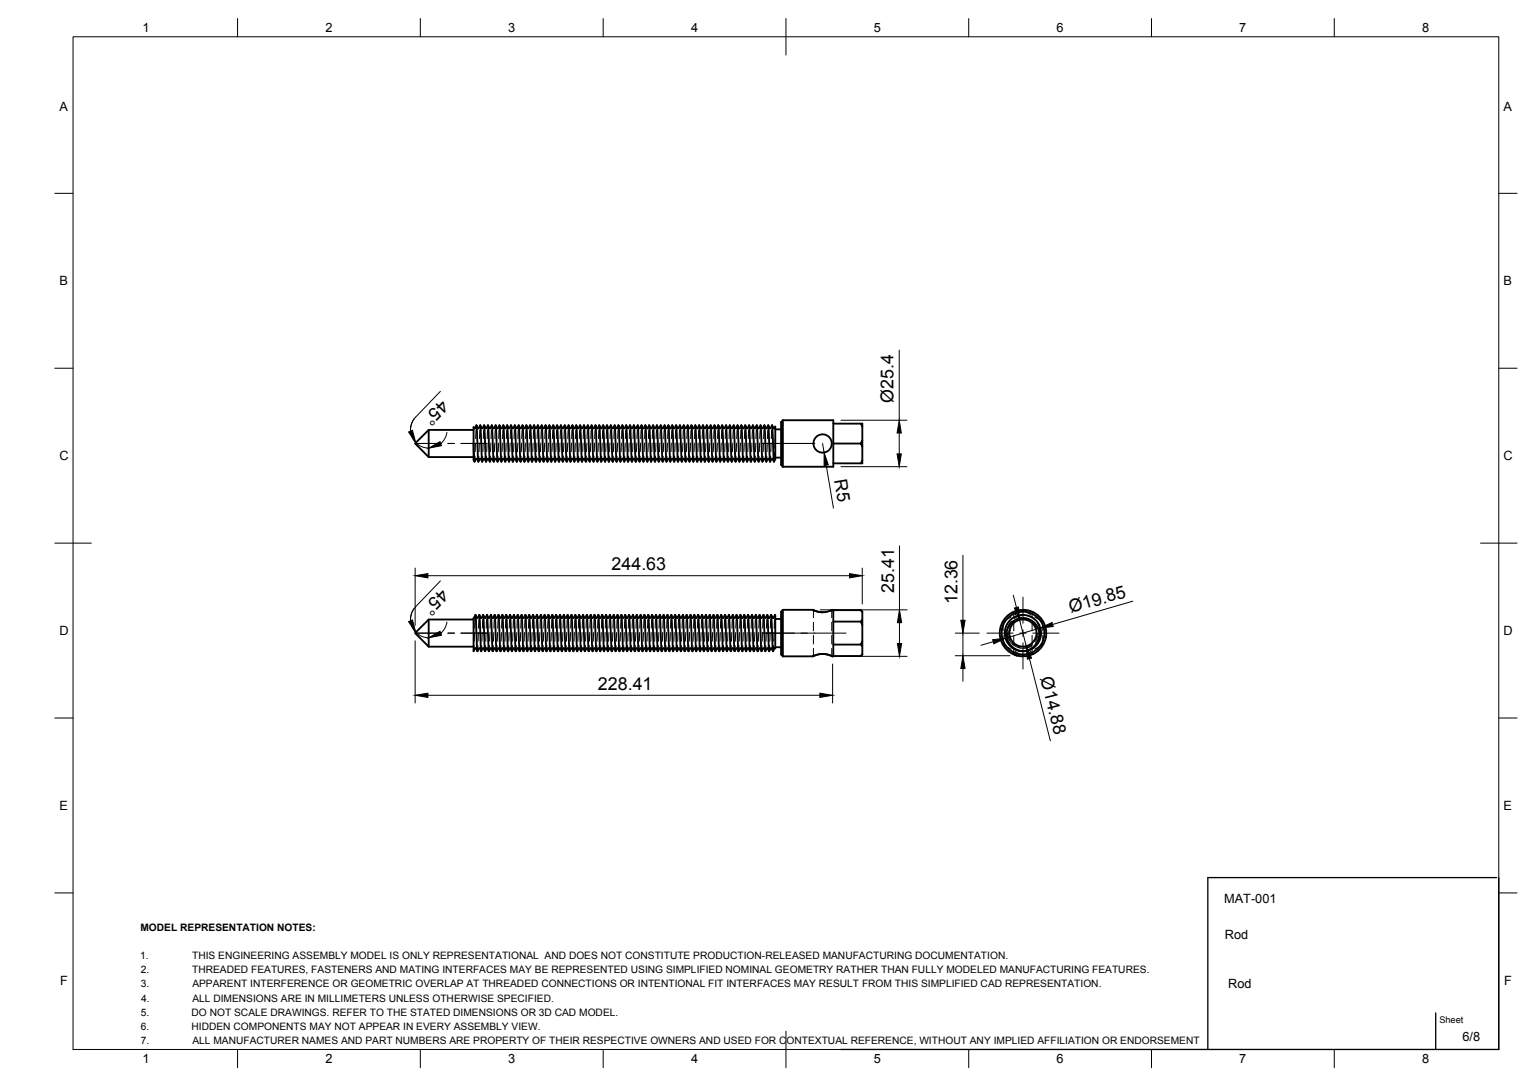
ISO-10303-21;
HEADER;
/* Generated by software containing ST-Developer
 * from STEP Tools, Inc. (www.steptools.com) 
 */

FILE_DESCRIPTION(
/* description */ ('STEP AP214'),
/* implementation_level */ '2;1');

FILE_NAME(
/* name */ 'Rod.step',
/* time_stamp */ '2026-11-14T04:30:00-08:00',
/* author */ (''),
/* organization */ (''),
/* preprocessor_version */ 'ST-DEVELOPER v20.2',
/* originating_system */ 'Autodesk Translation Framework v15.17.0.0',
/* authorisation */ '');

FILE_SCHEMA (('AUTOMOTIVE_DESIGN { 1 0 10303 214 3 1 1 }'));
ENDSEC;

DATA;
#10=MECHANICAL_DESIGN_GEOMETRIC_PRESENTATION_REPRESENTATION('',(#124),#40809);
#108=SHAPE_REPRESENTATION_RELATIONSHIP('SRR','None',#40858,#116);
#116=ADVANCED_BREP_SHAPE_REPRESENTATION('',(#132),#40802);
#124=STYLED_ITEM('',(#40907),#132);
#132=MANIFOLD_SOLID_BREP('Body1',#6299);
#176=(
BOUNDED_SURFACE()
B_SPLINE_SURFACE(3,2,((#27166,#27167,#27168),(#27169,#27170,#27171),(#27172,
#27173,#27174),(#27175,#27176,#27177),(#27178,#27179,#27180),(#27181,#27182,
#27183),(#27184,#27185,#27186),(#27187,#27188,#27189),(#27190,#27191,#27192),
(#27193,#27194,#27195),(#27196,#27197,#27198),(#27199,#27200,#27201),(#27202,
#27203,#27204),(#27205,#27206,#27207),(#27208,#27209,#27210),(#27211,#27212,
#27213),(#27214,#27215,#27216),(#27217,#27218,#27219),(#27220,#27221,#27222),
(#27223,#27224,#27225),(#27226,#27227,#27228),(#27229,#27230,#27231),(#27232,
#27233,#27234),(#27235,#27236,#27237),(#27238,#27239,#27240),(#27241,#27242,
#27243),(#27244,#27245,#27246),(#27247,#27248,#27249),(#27250,#27251,#27252),
(#27253,#27254,#27255),(#27256,#27257,#27258),(#27259,#27260,#27261),(#27262,
#27263,#27264),(#27265,#27266,#27267),(#27268,#27269,#27270),(#27271,#27272,
#27273),(#27274,#27275,#27276),(#27277,#27278,#27279),(#27280,#27281,#27282),
(#27283,#27284,#27285),(#27286,#27287,#27288),(#27289,#27290,#27291)),
 .UNSPECIFIED.,.F.,.F.,.F.)
B_SPLINE_SURFACE_WITH_KNOTS((4,2,2,2,2,2,2,2,2,2,2,2,2,2,2,2,2,2,2,2,4),
(3,3),(-7.80561738159264E-5,0.00108972446965002,0.00217944893930003,0.00326917340895005,
0.00435889787860006,0.00490376011342507,0.00544862234825008,0.00653834681790009,
0.00762807128755011,0.00871779575720013,0.00926265799202513,0.00980752022685014,
0.0103523824616751,0.0108972446965002,0.0119869691661502,0.0130766936358002,
0.0141664181054502,0.0152561425751002,0.0158010048099252,0.0163458670447502,
0.0174687351854262),(-3.31436710259121E-5,1.00007805617382),
 .UNSPECIFIED.)
GEOMETRIC_REPRESENTATION_ITEM()
RATIONAL_B_SPLINE_SURFACE(((1.00003154503853,0.524079561564375,1.00007429459434),
(1.0000315937412,0.523344783661835,1.00007440929844),(1.00003141682542,
0.526013914411658,1.00007399262799),(1.0000307068602,0.536725169717461,
1.0000723205242),(1.00003019055673,0.544514647394406,1.00007110453086),
(1.00002895723913,0.563121727335801,1.00006819983221),(1.0000282411969,
0.573924666524174,1.00006651341591),(1.00002671338234,0.596974826160331,
1.00006291512064),(1.00002591662213,0.608995558662043,1.00006103859807),
(1.00002475586398,0.626507933141575,1.00005830479079),(1.00002437347723,
0.632277007329064,1.00005740419693),(1.00002362687254,0.643541042834223,
1.00005564580019),(1.00002326100253,0.649060928800113,1.00005478410639),
(1.00002222356725,0.664712729342052,1.00005234074805),(1.00002160723677,
0.674011315953667,1.00005088917198),(1.00002057219885,0.689626947600185,
1.00004845145987),(1.00002015115486,0.695979244110157,1.00004745982082),
(1.00001958356106,0.704542539723916,1.00004612302894),(1.00001943064549,
0.706849579098284,1.00004576288355),(1.00001940985656,0.707163222049774,
1.00004571392163),(1.00001943845365,0.706731777363891,1.00004578127324),
(1.00001956476706,0.704826085066601,1.00004607876548),(1.00001966207446,
0.703358006931155,1.00004630794301),(1.00001992151192,0.69944387046907,
1.00004691896779),(1.00002008365206,0.696997659863913,1.00004730083881),
(1.00002047017319,0.691166210187756,1.00004821116994),(1.00002069610127,
0.687757630052989,1.00004874327375),(1.00002145040546,0.676377432111549,
1.00005051980428),(1.00002205383492,0.667273483461506,1.00005194099597),
(1.00002340996085,0.646813592510669,1.00005513493171),(1.0000241670402,
0.635391525693089,1.00005691799827),(1.00002570900064,0.612127947016899,
1.00006054960978),(1.00002650093244,0.600180060818586,1.00006241476052),
(1.0000280417883,0.576933146876439,1.00006604377054),(1.00002877367107,
0.565891221185074,1.00006776749435),(1.00002972027581,0.551609782278378,
1.00006999692941),(1.0000300115584,0.547215197654337,1.00007068295559),
(1.00003053161739,0.53936906050514,1.00007190779388),(1.00003076145279,
0.535901530604989,1.00007244910017),(1.00003133743645,0.527211656986592,
1.00007380565178),(1.00003154549653,0.52407265171366,1.00007429567302),
(1.00003155264458,0.523964808953251,1.00007431250805)))
REPRESENTATION_ITEM('')
SURFACE()
);
#177=(
BOUNDED_SURFACE()
B_SPLINE_SURFACE(3,2,((#27578,#27579,#27580),(#27581,#27582,#27583),(#27584,
#27585,#27586),(#27587,#27588,#27589),(#27590,#27591,#27592),(#27593,#27594,
#27595),(#27596,#27597,#27598),(#27599,#27600,#27601),(#27602,#27603,#27604),
(#27605,#27606,#27607),(#27608,#27609,#27610),(#27611,#27612,#27613),(#27614,
#27615,#27616),(#27617,#27618,#27619),(#27620,#27621,#27622),(#27623,#27624,
#27625),(#27626,#27627,#27628),(#27629,#27630,#27631),(#27632,#27633,#27634),
(#27635,#27636,#27637),(#27638,#27639,#27640),(#27641,#27642,#27643),(#27644,
#27645,#27646),(#27647,#27648,#27649),(#27650,#27651,#27652),(#27653,#27654,
#27655),(#27656,#27657,#27658),(#27659,#27660,#27661),(#27662,#27663,#27664),
(#27665,#27666,#27667),(#27668,#27669,#27670),(#27671,#27672,#27673),(#27674,
#27675,#27676),(#27677,#27678,#27679),(#27680,#27681,#27682),(#27683,#27684,
#27685),(#27686,#27687,#27688),(#27689,#27690,#27691),(#27692,#27693,#27694),
(#27695,#27696,#27697),(#27698,#27699,#27700),(#27701,#27702,#27703)),
 .UNSPECIFIED.,.F.,.F.,.F.)
B_SPLINE_SURFACE_WITH_KNOTS((4,2,2,2,2,2,2,2,2,2,2,2,2,2,2,2,2,2,2,2,4),
(3,3),(0.,0.00108936814645749,0.00217873629291499,0.00326810443937248,0.00435747258582998,
0.00490215665905872,0.00544684073228747,0.00653620887874497,0.00762557702520246,
0.00871494517165995,0.0092596292448887,0.00980431331811745,0.0103489973913462,
0.0108936814645749,0.0119830496110324,0.0130724177574899,0.0141617859039474,
0.0152511540504049,0.0157958381236337,0.0163405221968624,0.0174298903433199),
(0.,1.),.UNSPECIFIED.)
GEOMETRIC_REPRESENTATION_ITEM()
RATIONAL_B_SPLINE_SURFACE(((1.,0.706882331541542,1.),(1.,0.707679638835941,
1.),(1.,0.706337831680188,1.),(1.,0.699641298231053,1.),(1.,0.694186850878167,
1.),(1.,0.680019624674915,1.),(1.,0.671327778173696,1.),(1.,0.65139771038903,
1.),(1.,0.640295384304893,1.),(1.,0.623043177807755,1.),(1.,0.617175274503255,
1.),(1.,0.605346721741376,1.),(1.,0.599355525156456,1.),(1.,0.581798773133271,
1.),(1.,0.570600832874572,1.),(1.,0.550711868458482,1.),(1.,0.541963614343013,
1.),(1.,0.529372137830182,1.),(1.,0.525443344962623,1.),(1.,0.523784577113156,
1.),(1.,0.523945004135255,1.),(1.,0.525692544902627,1.),(1.,0.527267041649223,
1.),(1.,0.531692982742457,1.),(1.,0.534544195639033,1.),(1.,0.541381698420683,
1.),(1.,0.545393688389137,1.),(1.,0.55869257877852,1.),(1.,0.569170005808865,
1.),(1.,0.591697019613681,1.),(1.,0.603798924645628,1.),(1.,0.6273058031179,
1.),(1.,0.638830492715536,1.),(1.,0.660348218640802,1.),(1.,0.670109592161733,
1.),(1.,0.682456253372296,1.),(1.,0.686205595551818,1.),(1.,0.692883150338747,
1.),(1.,0.695824965165441,1.),(1.,0.703162804007318,1.),(1.,0.706044886129699,
1.),(1.,0.706866009891837,1.)))
REPRESENTATION_ITEM('')
SURFACE()
);
#178=(
BOUNDED_SURFACE()
B_SPLINE_SURFACE(1,2,((#28772,#28773,#28774,#28775,#28776,#28777,#28778,
#28779,#28780,#28781,#28782,#28783,#28784,#28785,#28786,#28787,#28788,#28789,
#28790,#28791,#28792,#28793,#28794,#28795,#28796,#28797,#28798,#28799,#28800,
#28801,#28802,#28803,#28804,#28805,#28806,#28807,#28808,#28809,#28810,#28811,
#28812,#28813,#28814,#28815,#28816,#28817,#28818,#28819,#28820,#28821,#28822,
#28823,#28824,#28825,#28826,#28827,#28828,#28829,#28830,#28831,#28832,#28833,
#28834,#28835,#28836,#28837,#28838,#28839,#28840,#28841,#28842,#28843,#28844,
#28845,#28846,#28847,#28848,#28849,#28850,#28851,#28852,#28853,#28854,#28855,
#28856,#28857,#28858,#28859,#28860,#28861,#28862,#28863,#28864,#28865,#28866,
#28867,#28868,#28869,#28870,#28871,#28872,#28873,#28874,#28875,#28876,#28877,
#28878,#28879,#28880,#28881,#28882,#28883,#28884,#28885,#28886,#28887,#28888,
#28889,#28890,#28891,#28892,#28893,#28894,#28895,#28896,#28897,#28898,#28899,
#28900,#28901,#28902,#28903,#28904,#28905,#28906,#28907,#28908,#28909,#28910,
#28911,#28912,#28913,#28914,#28915,#28916,#28917,#28918,#28919,#28920,#28921,
#28922,#28923,#28924,#28925,#28926,#28927,#28928,#28929,#28930,#28931,#28932,
#28933,#28934,#28935,#28936,#28937,#28938,#28939,#28940,#28941,#28942,#28943,
#28944,#28945,#28946,#28947,#28948,#28949,#28950,#28951,#28952,#28953,#28954,
#28955,#28956,#28957,#28958,#28959,#28960,#28961,#28962,#28963,#28964,#28965,
#28966,#28967,#28968,#28969,#28970,#28971,#28972,#28973,#28974,#28975,#28976,
#28977,#28978,#28979,#28980,#28981,#28982,#28983,#28984,#28985,#28986,#28987,
#28988,#28989,#28990,#28991,#28992,#28993,#28994,#28995,#28996,#28997,#28998,
#28999,#29000,#29001,#29002,#29003,#29004,#29005,#29006,#29007,#29008,#29009,
#29010,#29011,#29012,#29013,#29014,#29015,#29016,#29017,#29018,#29019,#29020,
#29021,#29022,#29023,#29024,#29025,#29026,#29027,#29028,#29029,#29030,#29031,
#29032,#29033,#29034,#29035,#29036,#29037,#29038,#29039,#29040,#29041,#29042,
#29043,#29044,#29045,#29046,#29047,#29048,#29049,#29050,#29051,#29052,#29053,
#29054,#29055,#29056,#29057,#29058,#29059,#29060,#29061,#29062,#29063,#29064,
#29065,#29066,#29067,#29068,#29069,#29070,#29071,#29072,#29073,#29074,#29075,
#29076,#29077,#29078,#29079,#29080,#29081,#29082,#29083,#29084,#29085,#29086,
#29087,#29088,#29089,#29090,#29091,#29092,#29093,#29094,#29095,#29096,#29097,
#29098,#29099,#29100,#29101,#29102,#29103,#29104,#29105,#29106,#29107,#29108,
#29109,#29110,#29111,#29112,#29113,#29114,#29115,#29116,#29117,#29118,#29119,
#29120,#29121,#29122,#29123,#29124,#29125,#29126,#29127,#29128,#29129,#29130,
#29131,#29132,#29133,#29134,#29135,#29136,#29137,#29138,#29139,#29140,#29141,
#29142,#29143,#29144,#29145,#29146,#29147,#29148,#29149,#29150,#29151,#29152,
#29153,#29154,#29155,#29156,#29157,#29158,#29159,#29160,#29161,#29162,#29163,
#29164,#29165,#29166,#29167,#29168,#29169,#29170,#29171,#29172,#29173,#29174,
#29175,#29176,#29177,#29178,#29179,#29180,#29181,#29182,#29183,#29184,#29185,
#29186,#29187,#29188,#29189,#29190,#29191,#29192,#29193,#29194,#29195,#29196,
#29197,#29198,#29199,#29200,#29201,#29202,#29203,#29204,#29205,#29206,#29207,
#29208,#29209,#29210,#29211,#29212,#29213,#29214,#29215,#29216,#29217,#29218,
#29219,#29220,#29221,#29222,#29223,#29224,#29225,#29226,#29227,#29228,#29229,
#29230,#29231,#29232,#29233,#29234,#29235,#29236,#29237,#29238,#29239,#29240,
#29241,#29242,#29243,#29244,#29245,#29246,#29247,#29248,#29249,#29250,#29251,
#29252,#29253,#29254,#29255,#29256,#29257,#29258,#29259,#29260,#29261,#29262,
#29263,#29264,#29265,#29266,#29267,#29268,#29269,#29270,#29271,#29272,#29273,
#29274,#29275,#29276,#29277,#29278,#29279,#29280,#29281,#29282,#29283,#29284,
#29285,#29286,#29287,#29288,#29289,#29290,#29291,#29292,#29293,#29294,#29295,
#29296,#29297,#29298,#29299,#29300,#29301,#29302,#29303,#29304,#29305,#29306,
#29307,#29308,#29309,#29310,#29311,#29312,#29313,#29314,#29315,#29316,#29317,
#29318,#29319,#29320,#29321,#29322,#29323,#29324,#29325,#29326,#29327,#29328,
#29329,#29330,#29331,#29332,#29333,#29334,#29335,#29336,#29337,#29338,#29339,
#29340,#29341,#29342,#29343,#29344,#29345,#29346,#29347,#29348,#29349,#29350,
#29351,#29352,#29353,#29354,#29355,#29356,#29357,#29358,#29359,#29360,#29361,
#29362,#29363,#29364,#29365,#29366,#29367,#29368,#29369,#29370,#29371,#29372,
#29373,#29374,#29375,#29376,#29377,#29378,#29379,#29380,#29381,#29382,#29383,
#29384,#29385,#29386,#29387,#29388,#29389,#29390,#29391,#29392,#29393,#29394,
#29395,#29396,#29397,#29398,#29399,#29400,#29401,#29402,#29403,#29404,#29405,
#29406,#29407,#29408,#29409,#29410,#29411,#29412,#29413,#29414,#29415,#29416,
#29417,#29418,#29419,#29420,#29421,#29422,#29423,#29424,#29425,#29426,#29427,
#29428,#29429,#29430,#29431,#29432,#29433,#29434,#29435,#29436,#29437,#29438,
#29439,#29440,#29441,#29442,#29443,#29444,#29445,#29446,#29447,#29448,#29449,
#29450,#29451,#29452,#29453,#29454,#29455,#29456,#29457,#29458,#29459,#29460,
#29461,#29462,#29463,#29464,#29465,#29466,#29467,#29468,#29469,#29470,#29471,
#29472,#29473,#29474,#29475,#29476,#29477,#29478,#29479,#29480,#29481,#29482,
#29483,#29484,#29485,#29486,#29487,#29488,#29489,#29490,#29491,#29492,#29493,
#29494,#29495,#29496,#29497,#29498,#29499,#29500,#29501,#29502,#29503,#29504,
#29505,#29506,#29507,#29508,#29509,#29510,#29511,#29512,#29513,#29514,#29515,
#29516,#29517,#29518,#29519,#29520,#29521,#29522,#29523,#29524,#29525,#29526,
#29527,#29528,#29529,#29530,#29531,#29532,#29533,#29534,#29535,#29536,#29537,
#29538,#29539,#29540,#29541,#29542,#29543,#29544,#29545,#29546,#29547,#29548,
#29549,#29550,#29551,#29552,#29553,#29554,#29555,#29556,#29557,#29558,#29559,
#29560,#29561,#29562,#29563,#29564,#29565,#29566,#29567,#29568,#29569,#29570,
#29571,#29572,#29573,#29574,#29575,#29576,#29577,#29578,#29579,#29580,#29581,
#29582,#29583,#29584,#29585,#29586,#29587,#29588,#29589,#29590,#29591,#29592,
#29593,#29594,#29595,#29596,#29597,#29598,#29599,#29600,#29601,#29602,#29603,
#29604,#29605,#29606,#29607,#29608,#29609,#29610,#29611,#29612,#29613,#29614,
#29615,#29616,#29617,#29618,#29619,#29620,#29621,#29622,#29623,#29624,#29625,
#29626,#29627,#29628,#29629,#29630,#29631,#29632,#29633,#29634,#29635,#29636,
#29637,#29638,#29639,#29640,#29641,#29642,#29643,#29644,#29645,#29646,#29647,
#29648,#29649,#29650,#29651,#29652,#29653,#29654,#29655,#29656,#29657,#29658,
#29659,#29660,#29661,#29662,#29663,#29664,#29665,#29666,#29667,#29668,#29669,
#29670,#29671,#29672,#29673,#29674,#29675,#29676,#29677,#29678,#29679,#29680,
#29681,#29682,#29683,#29684,#29685,#29686,#29687,#29688,#29689,#29690,#29691,
#29692,#29693,#29694,#29695,#29696,#29697,#29698,#29699,#29700,#29701,#29702,
#29703,#29704,#29705,#29706,#29707,#29708,#29709,#29710,#29711,#29712,#29713,
#29714,#29715,#29716,#29717,#29718,#29719,#29720,#29721,#29722,#29723,#29724,
#29725,#29726,#29727,#29728,#29729,#29730,#29731,#29732,#29733,#29734,#29735,
#29736,#29737,#29738,#29739,#29740,#29741,#29742,#29743,#29744),(#29745,
#29746,#29747,#29748,#29749,#29750,#29751,#29752,#29753,#29754,#29755,#29756,
#29757,#29758,#29759,#29760,#29761,#29762,#29763,#29764,#29765,#29766,#29767,
#29768,#29769,#29770,#29771,#29772,#29773,#29774,#29775,#29776,#29777,#29778,
#29779,#29780,#29781,#29782,#29783,#29784,#29785,#29786,#29787,#29788,#29789,
#29790,#29791,#29792,#29793,#29794,#29795,#29796,#29797,#29798,#29799,#29800,
#29801,#29802,#29803,#29804,#29805,#29806,#29807,#29808,#29809,#29810,#29811,
#29812,#29813,#29814,#29815,#29816,#29817,#29818,#29819,#29820,#29821,#29822,
#29823,#29824,#29825,#29826,#29827,#29828,#29829,#29830,#29831,#29832,#29833,
#29834,#29835,#29836,#29837,#29838,#29839,#29840,#29841,#29842,#29843,#29844,
#29845,#29846,#29847,#29848,#29849,#29850,#29851,#29852,#29853,#29854,#29855,
#29856,#29857,#29858,#29859,#29860,#29861,#29862,#29863,#29864,#29865,#29866,
#29867,#29868,#29869,#29870,#29871,#29872,#29873,#29874,#29875,#29876,#29877,
#29878,#29879,#29880,#29881,#29882,#29883,#29884,#29885,#29886,#29887,#29888,
#29889,#29890,#29891,#29892,#29893,#29894,#29895,#29896,#29897,#29898,#29899,
#29900,#29901,#29902,#29903,#29904,#29905,#29906,#29907,#29908,#29909,#29910,
#29911,#29912,#29913,#29914,#29915,#29916,#29917,#29918,#29919,#29920,#29921,
#29922,#29923,#29924,#29925,#29926,#29927,#29928,#29929,#29930,#29931,#29932,
#29933,#29934,#29935,#29936,#29937,#29938,#29939,#29940,#29941,#29942,#29943,
#29944,#29945,#29946,#29947,#29948,#29949,#29950,#29951,#29952,#29953,#29954,
#29955,#29956,#29957,#29958,#29959,#29960,#29961,#29962,#29963,#29964,#29965,
#29966,#29967,#29968,#29969,#29970,#29971,#29972,#29973,#29974,#29975,#29976,
#29977,#29978,#29979,#29980,#29981,#29982,#29983,#29984,#29985,#29986,#29987,
#29988,#29989,#29990,#29991,#29992,#29993,#29994,#29995,#29996,#29997,#29998,
#29999,#30000,#30001,#30002,#30003,#30004,#30005,#30006,#30007,#30008,#30009,
#30010,#30011,#30012,#30013,#30014,#30015,#30016,#30017,#30018,#30019,#30020,
#30021,#30022,#30023,#30024,#30025,#30026,#30027,#30028,#30029,#30030,#30031,
#30032,#30033,#30034,#30035,#30036,#30037,#30038,#30039,#30040,#30041,#30042,
#30043,#30044,#30045,#30046,#30047,#30048,#30049,#30050,#30051,#30052,#30053,
#30054,#30055,#30056,#30057,#30058,#30059,#30060,#30061,#30062,#30063,#30064,
#30065,#30066,#30067,#30068,#30069,#30070,#30071,#30072,#30073,#30074,#30075,
#30076,#30077,#30078,#30079,#30080,#30081,#30082,#30083,#30084,#30085,#30086,
#30087,#30088,#30089,#30090,#30091,#30092,#30093,#30094,#30095,#30096,#30097,
#30098,#30099,#30100,#30101,#30102,#30103,#30104,#30105,#30106,#30107,#30108,
#30109,#30110,#30111,#30112,#30113,#30114,#30115,#30116,#30117,#30118,#30119,
#30120,#30121,#30122,#30123,#30124,#30125,#30126,#30127,#30128,#30129,#30130,
#30131,#30132,#30133,#30134,#30135,#30136,#30137,#30138,#30139,#30140,#30141,
#30142,#30143,#30144,#30145,#30146,#30147,#30148,#30149,#30150,#30151,#30152,
#30153,#30154,#30155,#30156,#30157,#30158,#30159,#30160,#30161,#30162,#30163,
#30164,#30165,#30166,#30167,#30168,#30169,#30170,#30171,#30172,#30173,#30174,
#30175,#30176,#30177,#30178,#30179,#30180,#30181,#30182,#30183,#30184,#30185,
#30186,#30187,#30188,#30189,#30190,#30191,#30192,#30193,#30194,#30195,#30196,
#30197,#30198,#30199,#30200,#30201,#30202,#30203,#30204,#30205,#30206,#30207,
#30208,#30209,#30210,#30211,#30212,#30213,#30214,#30215,#30216,#30217,#30218,
#30219,#30220,#30221,#30222,#30223,#30224,#30225,#30226,#30227,#30228,#30229,
#30230,#30231,#30232,#30233,#30234,#30235,#30236,#30237,#30238,#30239,#30240,
#30241,#30242,#30243,#30244,#30245,#30246,#30247,#30248,#30249,#30250,#30251,
#30252,#30253,#30254,#30255,#30256,#30257,#30258,#30259,#30260,#30261,#30262,
#30263,#30264,#30265,#30266,#30267,#30268,#30269,#30270,#30271,#30272,#30273,
#30274,#30275,#30276,#30277,#30278,#30279,#30280,#30281,#30282,#30283,#30284,
#30285,#30286,#30287,#30288,#30289,#30290,#30291,#30292,#30293,#30294,#30295,
#30296,#30297,#30298,#30299,#30300,#30301,#30302,#30303,#30304,#30305,#30306,
#30307,#30308,#30309,#30310,#30311,#30312,#30313,#30314,#30315,#30316,#30317,
#30318,#30319,#30320,#30321,#30322,#30323,#30324,#30325,#30326,#30327,#30328,
#30329,#30330,#30331,#30332,#30333,#30334,#30335,#30336,#30337,#30338,#30339,
#30340,#30341,#30342,#30343,#30344,#30345,#30346,#30347,#30348,#30349,#30350,
#30351,#30352,#30353,#30354,#30355,#30356,#30357,#30358,#30359,#30360,#30361,
#30362,#30363,#30364,#30365,#30366,#30367,#30368,#30369,#30370,#30371,#30372,
#30373,#30374,#30375,#30376,#30377,#30378,#30379,#30380,#30381,#30382,#30383,
#30384,#30385,#30386,#30387,#30388,#30389,#30390,#30391,#30392,#30393,#30394,
#30395,#30396,#30397,#30398,#30399,#30400,#30401,#30402,#30403,#30404,#30405,
#30406,#30407,#30408,#30409,#30410,#30411,#30412,#30413,#30414,#30415,#30416,
#30417,#30418,#30419,#30420,#30421,#30422,#30423,#30424,#30425,#30426,#30427,
#30428,#30429,#30430,#30431,#30432,#30433,#30434,#30435,#30436,#30437,#30438,
#30439,#30440,#30441,#30442,#30443,#30444,#30445,#30446,#30447,#30448,#30449,
#30450,#30451,#30452,#30453,#30454,#30455,#30456,#30457,#30458,#30459,#30460,
#30461,#30462,#30463,#30464,#30465,#30466,#30467,#30468,#30469,#30470,#30471,
#30472,#30473,#30474,#30475,#30476,#30477,#30478,#30479,#30480,#30481,#30482,
#30483,#30484,#30485,#30486,#30487,#30488,#30489,#30490,#30491,#30492,#30493,
#30494,#30495,#30496,#30497,#30498,#30499,#30500,#30501,#30502,#30503,#30504,
#30505,#30506,#30507,#30508,#30509,#30510,#30511,#30512,#30513,#30514,#30515,
#30516,#30517,#30518,#30519,#30520,#30521,#30522,#30523,#30524,#30525,#30526,
#30527,#30528,#30529,#30530,#30531,#30532,#30533,#30534,#30535,#30536,#30537,
#30538,#30539,#30540,#30541,#30542,#30543,#30544,#30545,#30546,#30547,#30548,
#30549,#30550,#30551,#30552,#30553,#30554,#30555,#30556,#30557,#30558,#30559,
#30560,#30561,#30562,#30563,#30564,#30565,#30566,#30567,#30568,#30569,#30570,
#30571,#30572,#30573,#30574,#30575,#30576,#30577,#30578,#30579,#30580,#30581,
#30582,#30583,#30584,#30585,#30586,#30587,#30588,#30589,#30590,#30591,#30592,
#30593,#30594,#30595,#30596,#30597,#30598,#30599,#30600,#30601,#30602,#30603,
#30604,#30605,#30606,#30607,#30608,#30609,#30610,#30611,#30612,#30613,#30614,
#30615,#30616,#30617,#30618,#30619,#30620,#30621,#30622,#30623,#30624,#30625,
#30626,#30627,#30628,#30629,#30630,#30631,#30632,#30633,#30634,#30635,#30636,
#30637,#30638,#30639,#30640,#30641,#30642,#30643,#30644,#30645,#30646,#30647,
#30648,#30649,#30650,#30651,#30652,#30653,#30654,#30655,#30656,#30657,#30658,
#30659,#30660,#30661,#30662,#30663,#30664,#30665,#30666,#30667,#30668,#30669,
#30670,#30671,#30672,#30673,#30674,#30675,#30676,#30677,#30678,#30679,#30680,
#30681,#30682,#30683,#30684,#30685,#30686,#30687,#30688,#30689,#30690,#30691,
#30692,#30693,#30694,#30695,#30696,#30697,#30698,#30699,#30700,#30701,#30702,
#30703,#30704,#30705,#30706,#30707,#30708,#30709,#30710,#30711,#30712,#30713,
#30714,#30715,#30716,#30717)),.UNSPECIFIED.,.F.,.F.,.F.)
B_SPLINE_SURFACE_WITH_KNOTS((2,2),(3,2,2,2,2,2,2,2,2,2,2,2,2,2,2,2,2,2,
2,2,2,2,2,2,2,2,2,2,2,2,2,2,2,2,2,2,2,2,2,2,2,2,2,2,2,2,2,2,2,2,2,2,2,2,
2,2,2,2,2,2,2,2,2,2,2,2,2,2,2,2,2,2,2,2,2,2,2,2,2,2,2,2,2,2,2,2,2,2,2,2,
2,2,2,2,2,2,2,2,2,2,2,2,2,2,2,2,2,2,2,2,2,2,2,2,2,2,2,2,2,2,2,2,2,2,2,2,
2,2,2,2,2,2,2,2,2,2,2,2,2,2,2,2,2,2,2,2,2,2,2,2,2,2,2,2,2,2,2,2,2,2,2,2,
2,2,2,2,2,2,2,2,2,2,2,2,2,2,2,2,2,2,2,2,2,2,2,2,2,2,2,2,2,2,2,2,2,2,2,2,
2,2,2,2,2,2,2,2,2,2,2,2,2,2,2,2,2,2,2,2,2,2,2,2,2,2,2,2,2,2,2,2,2,2,2,2,
2,2,2,2,2,2,2,2,2,2,2,2,2,2,2,2,2,2,2,2,2,2,2,2,2,2,2,2,2,2,2,2,2,2,2,2,
2,2,2,2,2,2,2,2,2,2,2,2,2,2,2,2,2,2,2,2,2,2,2,2,2,2,2,2,2,2,2,2,2,2,2,2,
2,2,2,2,2,2,2,2,2,2,2,2,2,2,2,2,2,2,2,2,2,2,2,2,2,2,2,2,2,2,2,2,2,2,2,2,
2,2,2,2,2,2,2,2,2,2,2,2,2,2,2,2,2,2,2,2,2,2,2,2,2,2,2,2,2,2,2,2,2,2,2,2,
2,2,2,2,2,2,2,2,2,2,2,2,2,2,2,2,2,2,2,2,2,2,2,2,2,2,2,2,2,2,2,2,2,2,2,2,
2,2,2,2,2,2,2,2,2,2,2,2,2,2,2,2,2,2,2,2,2,2,2,2,2,2,2,2,2,2,2,2,2,2,2,2,
2,2,2,2,2,2,2,2,2,2,2,2,2,2,2,2,2,2,2,2,2,2,2,2,2,2,2,2,2,2,2,2,2,2,2,2,
3),(0.,1.),(0.,0.00205761316872428,0.00411522633744856,0.00617283950617284,
0.00823045267489712,0.0102880658436214,0.0123456790123457,0.01440329218107,
0.0164609053497942,0.0185185185185185,0.0205761316872428,0.0226337448559671,
0.0246913580246914,0.0267489711934156,0.0288065843621399,0.0308641975308642,
0.0329218106995885,0.0349794238683128,0.037037037037037,0.0390946502057613,
0.0411522633744856,0.0432098765432099,0.0452674897119342,0.0473251028806584,
0.0493827160493827,0.051440329218107,0.0534979423868313,0.0555555555555556,
0.0576131687242798,0.0596707818930041,0.0617283950617284,0.0637860082304527,
0.065843621399177,0.0679012345679012,0.0699588477366255,0.0720164609053498,
0.0740740740740741,0.0761316872427984,0.0781893004115226,0.0802469135802469,
0.0823045267489712,0.0843621399176955,0.0864197530864197,0.088477366255144,
0.0905349794238683,0.0925925925925926,0.0946502057613169,0.0967078189300412,
0.0987654320987654,0.10082304526749,0.102880658436214,0.104938271604938,
0.106995884773663,0.109053497942387,0.111111111111111,0.113168724279835,
0.11522633744856,0.117283950617284,0.119341563786008,0.121399176954733,
0.123456790123457,0.125514403292181,0.127572016460905,0.12962962962963,
0.131687242798354,0.133744855967078,0.135802469135802,0.137860082304527,
0.139917695473251,0.141975308641975,0.1440329218107,0.146090534979424,0.148148148148148,
0.150205761316872,0.152263374485597,0.154320987654321,0.156378600823045,
0.15843621399177,0.160493827160494,0.162551440329218,0.164609053497942,
0.166666666666667,0.168724279835391,0.170781893004115,0.172839506172839,
0.174897119341564,0.176954732510288,0.179012345679012,0.181069958847737,
0.183127572016461,0.185185185185185,0.187242798353909,0.189300411522634,
0.191358024691358,0.193415637860082,0.195473251028807,0.197530864197531,
0.199588477366255,0.201646090534979,0.203703703703704,0.205761316872428,
0.207818930041152,0.209876543209877,0.211934156378601,0.213991769547325,
0.216049382716049,0.218106995884774,0.220164609053498,0.222222222222222,
0.224279835390947,0.226337448559671,0.228395061728395,0.230452674897119,
0.232510288065844,0.234567901234568,0.236625514403292,0.238683127572016,
0.240740740740741,0.242798353909465,0.244855967078189,0.246913580246914,
0.248971193415638,0.251028806584362,0.253086419753086,0.255144032921811,
0.257201646090535,0.259259259259259,0.261316872427984,0.263374485596708,
0.265432098765432,0.267489711934156,0.269547325102881,0.271604938271605,
0.273662551440329,0.275720164609054,0.277777777777778,0.279835390946502,
0.281893004115226,0.283950617283951,0.286008230452675,0.288065843621399,
0.290123456790123,0.292181069958848,0.294238683127572,0.296296296296296,
0.298353909465021,0.300411522633745,0.302469135802469,0.304526748971193,
0.306584362139918,0.308641975308642,0.310699588477366,0.312757201646091,
0.314814814814815,0.316872427983539,0.318930041152263,0.320987654320988,
0.323045267489712,0.325102880658436,0.327160493827161,0.329218106995885,
0.331275720164609,0.333333333333333,0.335390946502058,0.337448559670782,
0.339506172839506,0.34156378600823,0.343621399176955,0.345679012345679,
0.347736625514403,0.349794238683128,0.351851851851852,0.353909465020576,
0.3559670781893,0.358024691358025,0.360082304526749,0.362139917695473,0.364197530864198,
0.366255144032922,0.368312757201646,0.37037037037037,0.372427983539095,
0.374485596707819,0.376543209876543,0.378600823045267,0.380658436213992,
0.382716049382716,0.38477366255144,0.386831275720165,0.388888888888889,
0.390946502057613,0.393004115226337,0.395061728395062,0.397119341563786,
0.39917695473251,0.401234567901235,0.403292181069959,0.405349794238683,
0.407407407407407,0.409465020576132,0.411522633744856,0.41358024691358,
0.415637860082305,0.417695473251029,0.419753086419753,0.421810699588477,
0.423868312757202,0.425925925925926,0.42798353909465,0.430041152263374,
0.432098765432099,0.434156378600823,0.436213991769547,0.438271604938272,
0.440329218106996,0.44238683127572,0.444444444444444,0.446502057613169,
0.448559670781893,0.450617283950617,0.452674897119342,0.454732510288066,
0.45679012345679,0.458847736625514,0.460905349794239,0.462962962962963,
0.465020576131687,0.467078189300412,0.469135802469136,0.47119341563786,
0.473251028806584,0.475308641975309,0.477366255144033,0.479423868312757,
0.481481481481481,0.483539094650206,0.48559670781893,0.487654320987654,
0.489711934156379,0.491769547325103,0.493827160493827,0.495884773662551,
0.497942386831276,0.5,0.502057613168724,0.504115226337449,0.506172839506173,
0.508230452674897,0.510288065843621,0.512345679012346,0.51440329218107,
0.516460905349794,0.518518518518518,0.520576131687243,0.522633744855967,
0.524691358024691,0.526748971193416,0.52880658436214,0.530864197530864,
0.532921810699588,0.534979423868313,0.537037037037037,0.539094650205761,
0.541152263374486,0.54320987654321,0.545267489711934,0.547325102880658,
0.549382716049383,0.551440329218107,0.553497942386831,0.555555555555556,
0.55761316872428,0.559670781893004,0.561728395061728,0.563786008230453,
0.565843621399177,0.567901234567901,0.569958847736626,0.57201646090535,
0.574074074074074,0.576131687242798,0.578189300411523,0.580246913580247,
0.582304526748971,0.584362139917695,0.58641975308642,0.588477366255144,
0.590534979423868,0.592592592592593,0.594650205761317,0.596707818930041,
0.598765432098765,0.60082304526749,0.602880658436214,0.604938271604938,
0.606995884773663,0.609053497942387,0.611111111111111,0.613168724279835,
0.61522633744856,0.617283950617284,0.619341563786008,0.621399176954732,
0.623456790123457,0.625514403292181,0.627572016460905,0.62962962962963,
0.631687242798354,0.633744855967078,0.635802469135803,0.637860082304527,
0.639917695473251,0.641975308641975,0.6440329218107,0.646090534979424,0.648148148148148,
0.650205761316872,0.652263374485597,0.654320987654321,0.656378600823045,
0.65843621399177,0.660493827160494,0.662551440329218,0.664609053497942,
0.666666666666667,0.668724279835391,0.670781893004115,0.672839506172839,
0.674897119341564,0.676954732510288,0.679012345679012,0.681069958847737,
0.683127572016461,0.685185185185185,0.687242798353909,0.689300411522634,
0.691358024691358,0.693415637860082,0.695473251028807,0.697530864197531,
0.699588477366255,0.701646090534979,0.703703703703704,0.705761316872428,
0.707818930041152,0.709876543209877,0.711934156378601,0.713991769547325,
0.716049382716049,0.718106995884774,0.720164609053498,0.722222222222222,
0.724279835390947,0.726337448559671,0.728395061728395,0.730452674897119,
0.732510288065844,0.734567901234568,0.736625514403292,0.738683127572016,
0.740740740740741,0.742798353909465,0.744855967078189,0.746913580246914,
0.748971193415638,0.751028806584362,0.753086419753086,0.755144032921811,
0.757201646090535,0.759259259259259,0.761316872427984,0.763374485596708,
0.765432098765432,0.767489711934156,0.769547325102881,0.771604938271605,
0.773662551440329,0.775720164609053,0.777777777777778,0.779835390946502,
0.781893004115226,0.783950617283951,0.786008230452675,0.788065843621399,
0.790123456790123,0.792181069958848,0.794238683127572,0.796296296296296,
0.798353909465021,0.800411522633745,0.802469135802469,0.804526748971193,
0.806584362139918,0.808641975308642,0.810699588477366,0.812757201646091,
0.814814814814815,0.816872427983539,0.818930041152263,0.820987654320988,
0.823045267489712,0.825102880658436,0.827160493827161,0.829218106995885,
0.831275720164609,0.833333333333333,0.835390946502058,0.837448559670782,
0.839506172839506,0.84156378600823,0.843621399176955,0.845679012345679,
0.847736625514403,0.849794238683128,0.851851851851852,0.853909465020576,
0.8559670781893,0.858024691358025,0.860082304526749,0.862139917695473,0.864197530864197,
0.866255144032922,0.868312757201646,0.87037037037037,0.872427983539095,
0.874485596707819,0.876543209876543,0.878600823045268,0.880658436213992,
0.882716049382716,0.88477366255144,0.886831275720165,0.888888888888889,
0.890946502057613,0.893004115226337,0.895061728395062,0.897119341563786,
0.89917695473251,0.901234567901235,0.903292181069959,0.905349794238683,
0.907407407407407,0.909465020576132,0.911522633744856,0.91358024691358,
0.915637860082305,0.917695473251029,0.919753086419753,0.921810699588477,
0.923868312757202,0.925925925925926,0.92798353909465,0.930041152263374,
0.932098765432099,0.934156378600823,0.936213991769547,0.938271604938272,
0.940329218106996,0.94238683127572,0.944444444444444,0.946502057613169,
0.948559670781893,0.950617283950617,0.952674897119342,0.954732510288066,
0.95679012345679,0.958847736625514,0.960905349794239,0.962962962962963,
0.965020576131687,0.967078189300412,0.969135802469136,0.97119341563786,
0.973251028806584,0.975308641975309,0.977366255144033,0.979423868312757,
0.981481481481482,0.983539094650206,0.98559670781893,0.987654320987654,
0.989711934156379,0.991769547325103,0.993827160493827,0.995884773662551,
0.997942386831276,1.),.UNSPECIFIED.)
GEOMETRIC_REPRESENTATION_ITEM()
RATIONAL_B_SPLINE_SURFACE(((1.,0.866025403784439,1.,0.866025403784439,1.,
0.866025403784439,1.,0.866025403784439,1.,0.866025403784439,1.,0.866025403784439,
1.,0.866025403784439,1.,0.866025403784439,1.,0.866025403784439,1.,0.866025403784439,
1.,0.866025403784439,1.,0.866025403784439,1.,0.866025403784439,1.,0.866025403784439,
1.,0.866025403784439,1.,0.866025403784439,1.,0.866025403784439,1.,0.866025403784439,
1.,0.866025403784439,1.,0.866025403784439,1.,0.866025403784439,1.,0.866025403784439,
1.,0.866025403784439,1.,0.866025403784439,1.,0.866025403784439,1.,0.866025403784439,
1.,0.866025403784439,1.,0.866025403784439,1.,0.866025403784439,1.,0.866025403784439,
1.,0.866025403784439,1.,0.866025403784439,1.,0.866025403784439,1.,0.866025403784439,
1.,0.866025403784439,1.,0.866025403784439,1.,0.866025403784439,1.,0.866025403784439,
1.,0.866025403784439,1.,0.866025403784439,1.,0.866025403784439,1.,0.866025403784439,
1.,0.866025403784439,1.,0.866025403784439,1.,0.866025403784439,1.,0.866025403784439,
1.,0.866025403784439,1.,0.866025403784439,1.,0.866025403784439,1.,0.866025403784439,
1.,0.866025403784439,1.,0.866025403784439,1.,0.866025403784439,1.,0.866025403784439,
1.,0.866025403784439,1.,0.866025403784439,1.,0.866025403784439,1.,0.866025403784439,
1.,0.866025403784439,1.,0.866025403784439,1.,0.866025403784439,1.,0.866025403784439,
1.,0.866025403784439,1.,0.866025403784439,1.,0.866025403784439,1.,0.866025403784439,
1.,0.866025403784439,1.,0.866025403784439,1.,0.866025403784439,1.,0.866025403784439,
1.,0.866025403784439,1.,0.866025403784439,1.,0.866025403784439,1.,0.866025403784439,
1.,0.866025403784439,1.,0.866025403784439,1.,0.866025403784439,1.,0.866025403784439,
1.,0.866025403784439,1.,0.866025403784439,1.,0.866025403784439,1.,0.866025403784439,
1.,0.866025403784439,1.,0.866025403784439,1.,0.866025403784439,1.,0.866025403784439,
1.,0.866025403784439,1.,0.866025403784439,1.,0.866025403784439,1.,0.866025403784439,
1.,0.866025403784439,1.,0.866025403784439,1.,0.866025403784439,1.,0.866025403784439,
1.,0.866025403784439,1.,0.866025403784439,1.,0.866025403784439,1.,0.866025403784439,
1.,0.866025403784439,1.,0.866025403784439,1.,0.866025403784439,1.,0.866025403784439,
1.,0.866025403784439,1.,0.866025403784439,1.,0.866025403784439,1.,0.866025403784439,
1.,0.866025403784439,1.,0.866025403784439,1.,0.866025403784439,1.,0.866025403784439,
1.,0.866025403784439,1.,0.866025403784439,1.,0.866025403784439,1.,0.866025403784439,
1.,0.866025403784439,1.,0.866025403784439,1.,0.866025403784439,1.,0.866025403784439,
1.,0.866025403784439,1.,0.866025403784439,1.,0.866025403784439,1.,0.866025403784439,
1.,0.866025403784439,1.,0.866025403784439,1.,0.866025403784439,1.,0.866025403784439,
1.,0.866025403784439,1.,0.866025403784439,1.,0.866025403784439,1.,0.866025403784439,
1.,0.866025403784439,1.,0.866025403784439,1.,0.866025403784439,1.,0.866025403784439,
1.,0.866025403784439,1.,0.866025403784439,1.,0.866025403784439,1.,0.866025403784439,
1.,0.866025403784439,1.,0.866025403784439,1.,0.866025403784439,1.,0.866025403784439,
1.,0.866025403784439,1.,0.866025403784439,1.,0.866025403784439,1.,0.866025403784439,
1.,0.866025403784439,1.,0.866025403784439,1.,0.866025403784439,1.,0.866025403784439,
1.,0.866025403784439,1.,0.866025403784439,1.,0.866025403784439,1.,0.866025403784439,
1.,0.866025403784439,1.,0.866025403784439,1.,0.866025403784439,1.,0.866025403784439,
1.,0.866025403784439,1.,0.866025403784439,1.,0.866025403784439,1.,0.866025403784439,
1.,0.866025403784439,1.,0.866025403784439,1.,0.866025403784439,1.,0.866025403784439,
1.,0.866025403784439,1.,0.866025403784439,1.,0.866025403784439,1.,0.866025403784439,
1.,0.866025403784439,1.,0.866025403784439,1.,0.866025403784439,1.,0.866025403784439,
1.,0.866025403784439,1.,0.866025403784439,1.,0.866025403784439,1.,0.866025403784439,
1.,0.866025403784439,1.,0.866025403784439,1.,0.866025403784439,1.,0.866025403784439,
1.,0.866025403784439,1.,0.866025403784439,1.,0.866025403784439,1.,0.866025403784439,
1.,0.866025403784439,1.,0.866025403784439,1.,0.866025403784439,1.,0.866025403784439,
1.,0.866025403784439,1.,0.866025403784439,1.,0.866025403784439,1.,0.866025403784439,
1.,0.866025403784439,1.,0.866025403784439,1.,0.866025403784439,1.,0.866025403784439,
1.,0.866025403784439,1.,0.866025403784439,1.,0.866025403784439,1.,0.866025403784439,
1.,0.866025403784439,1.,0.866025403784439,1.,0.866025403784439,1.,0.866025403784439,
1.,0.866025403784439,1.,0.866025403784439,1.,0.866025403784439,1.,0.866025403784439,
1.,0.866025403784439,1.,0.866025403784439,1.,0.866025403784439,1.,0.866025403784439,
1.,0.866025403784439,1.,0.866025403784439,1.,0.866025403784439,1.,0.866025403784439,
1.,0.866025403784439,1.,0.866025403784439,1.,0.866025403784439,1.,0.866025403784439,
1.,0.866025403784439,1.,0.866025403784439,1.,0.866025403784439,1.,0.866025403784439,
1.,0.866025403784439,1.,0.866025403784439,1.,0.866025403784439,1.,0.866025403784439,
1.,0.866025403784439,1.,0.866025403784439,1.,0.866025403784439,1.,0.866025403784439,
1.,0.866025403784439,1.,0.866025403784439,1.,0.866025403784439,1.,0.866025403784439,
1.,0.866025403784439,1.,0.866025403784439,1.,0.866025403784439,1.,0.866025403784439,
1.,0.866025403784439,1.,0.866025403784439,1.,0.866025403784439,1.,0.866025403784439,
1.,0.866025403784439,1.,0.866025403784439,1.,0.866025403784439,1.,0.866025403784439,
1.,0.866025403784439,1.,0.866025403784439,1.,0.866025403784439,1.,0.866025403784439,
1.,0.866025403784439,1.,0.866025403784439,1.,0.866025403784439,1.,0.866025403784439,
1.,0.866025403784439,1.,0.866025403784439,1.,0.866025403784439,1.,0.866025403784439,
1.,0.866025403784439,1.,0.866025403784439,1.,0.866025403784439,1.,0.866025403784439,
1.,0.866025403784439,1.,0.866025403784439,1.,0.866025403784439,1.,0.866025403784439,
1.,0.866025403784439,1.,0.866025403784439,1.,0.866025403784439,1.,0.866025403784439,
1.,0.866025403784439,1.,0.866025403784439,1.,0.866025403784439,1.,0.866025403784439,
1.,0.866025403784439,1.,0.866025403784439,1.,0.866025403784439,1.,0.866025403784439,
1.,0.866025403784439,1.,0.866025403784439,1.,0.866025403784439,1.,0.866025403784439,
1.,0.866025403784439,1.,0.866025403784439,1.,0.866025403784439,1.,0.866025403784439,
1.,0.866025403784439,1.,0.866025403784439,1.,0.866025403784439,1.,0.866025403784439,
1.,0.866025403784439,1.,0.866025403784439,1.,0.866025403784439,1.,0.866025403784439,
1.,0.866025403784439,1.,0.866025403784439,1.,0.866025403784439,1.,0.866025403784439,
1.,0.866025403784439,1.,0.866025403784439,1.,0.866025403784439,1.,0.866025403784439,
1.,0.866025403784439,1.,0.866025403784439,1.,0.866025403784439,1.,0.866025403784439,
1.,0.866025403784439,1.,0.866025403784439,1.,0.866025403784439,1.,0.866025403784439,
1.,0.866025403784439,1.,0.866025403784439,1.,0.866025403784439,1.,0.866025403784439,
1.,0.866025403784439,1.,0.866025403784439,1.,0.866025403784439,1.,0.866025403784439,
1.,0.866025403784439,1.,0.866025403784439,1.,0.866025403784439,1.,0.866025403784439,
1.,0.866025403784439,1.,0.866025403784439,1.,0.866025403784439,1.,0.866025403784439,
1.,0.866025403784439,1.,0.866025403784439,1.,0.866025403784439,1.,0.866025403784439,
1.,0.866025403784439,1.,0.866025403784439,1.,0.866025403784439,1.,0.866025403784439,
1.,0.866025403784439,1.,0.866025403784439,1.,0.866025403784439,1.,0.866025403784439,
1.,0.866025403784439,1.,0.866025403784439,1.,0.866025403784439,1.,0.866025403784439,
1.,0.866025403784439,1.,0.866025403784439,1.,0.866025403784439,1.,0.866025403784439,
1.,0.866025403784439,1.,0.866025403784439,1.,0.866025403784439,1.,0.866025403784439,
1.,0.866025403784439,1.,0.866025403784439,1.,0.866025403784439,1.,0.866025403784439,
1.,0.866025403784439,1.,0.866025403784439,1.,0.866025403784439,1.,0.866025403784439,
1.,0.866025403784439,1.,0.866025403784439,1.,0.866025403784439,1.,0.866025403784439,
1.,0.866025403784439,1.,0.866025403784439,1.,0.866025403784439,1.,0.866025403784439,
1.,0.866025403784439,1.,0.866025403784439,1.,0.866025403784439,1.,0.866025403784439,
1.,0.866025403784439,1.,0.866025403784439,1.,0.866025403784439,1.,0.866025403784439,
1.,0.866025403784439,1.,0.866025403784439,1.,0.866025403784439,1.,0.866025403784439,
1.,0.866025403784439,1.,0.866025403784439,1.,0.866025403784439,1.,0.866025403784439,
1.,0.866025403784439,1.,0.866025403784439,1.,0.866025403784439,1.,0.866025403784439,
1.,0.866025403784439,1.,0.866025403784439,1.,0.866025403784439,1.,0.866025403784439,
1.,0.866025403784439,1.,0.866025403784439,1.,0.866025403784439,1.,0.866025403784439,
1.,0.866025403784439,1.,0.866025403784439,1.,0.866025403784439,1.,0.866025403784439,
1.,0.866025403784439,1.,0.866025403784439,1.,0.866025403784439,1.,0.866025403784439,
1.,0.866025403784439,1.,0.866025403784439,1.,0.866025403784439,1.,0.866025403784439,
1.,0.866025403784439,1.,0.866025403784439,1.,0.866025403784439,1.,0.866025403784439,
1.,0.866025403784439,1.,0.866025403784439,1.,0.866025403784439,1.,0.866025403784439,
1.,0.866025403784439,1.,0.866025403784439,1.,0.866025403784439,1.,0.866025403784439,
1.,0.866025403784439,1.,0.866025403784439,1.,0.866025403784439,1.,0.866025403784439,
1.,0.866025403784439,1.,0.866025403784439,1.,0.866025403784439,1.,0.866025403784439,
1.,0.866025403784439,1.,0.866025403784439,1.,0.866025403784439,1.,0.866025403784439,
1.,0.866025403784439,1.,0.866025403784439,1.,0.866025403784439,1.,0.866025403784439,
1.,0.866025403784439,1.,0.866025403784439,1.,0.866025403784439,1.,0.866025403784439,
1.,0.866025403784439,1.,0.866025403784439,1.,0.866025403784439,1.,0.866025403784439,
1.,0.866025403784439,1.,0.866025403784439,1.,0.866025403784439,1.,0.866025403784439,
1.,0.866025403784439,1.,0.866025403784439,1.,0.866025403784439,1.,0.866025403784439,
1.,0.866025403784439,1.,0.866025403784439,1.,0.866025403784439,1.,0.866025403784439,
1.,0.866025403784439,1.,0.866025403784439,1.,0.866025403784439,1.,0.866025403784439,
1.,0.866025403784439,1.,0.866025403784439,1.,0.866025403784439,1.,0.866025403784439,
1.,0.866025403784439,1.,0.866025403784439,1.,0.866025403784439,1.,0.866025403784439,
1.,0.866025403784439,1.,0.866025403784439,1.,0.866025403784439,1.,0.866025403784439,
1.,0.866025403784439,1.,0.866025403784439,1.,0.866025403784439,1.,0.866025403784439,
1.,0.866025403784439,1.,0.866025403784439,1.,0.866025403784439,1.,0.866025403784439,
1.,0.866025403784439,1.,0.866025403784439,1.,0.866025403784439,1.,0.866025403784439,
1.),(1.,0.866025403784439,1.,0.866025403784439,1.,0.866025403784439,1.,
0.866025403784439,1.,0.866025403784439,1.,0.866025403784439,1.,0.866025403784439,
1.,0.866025403784439,1.,0.866025403784439,1.,0.866025403784439,1.,0.866025403784439,
1.,0.866025403784439,1.,0.866025403784439,1.,0.866025403784439,1.,0.866025403784439,
1.,0.866025403784439,1.,0.866025403784439,1.,0.866025403784439,1.,0.866025403784439,
1.,0.866025403784439,1.,0.866025403784439,1.,0.866025403784439,1.,0.866025403784439,
1.,0.866025403784439,1.,0.866025403784439,1.,0.866025403784439,1.,0.866025403784439,
1.,0.866025403784439,1.,0.866025403784439,1.,0.866025403784439,1.,0.866025403784439,
1.,0.866025403784439,1.,0.866025403784439,1.,0.866025403784439,1.,0.866025403784439,
1.,0.866025403784439,1.,0.866025403784439,1.,0.866025403784439,1.,0.866025403784439,
1.,0.866025403784439,1.,0.866025403784439,1.,0.866025403784439,1.,0.866025403784439,
1.,0.866025403784439,1.,0.866025403784439,1.,0.866025403784439,1.,0.866025403784439,
1.,0.866025403784439,1.,0.866025403784439,1.,0.866025403784439,1.,0.866025403784439,
1.,0.866025403784439,1.,0.866025403784439,1.,0.866025403784439,1.,0.866025403784439,
1.,0.866025403784439,1.,0.866025403784439,1.,0.866025403784439,1.,0.866025403784439,
1.,0.866025403784439,1.,0.866025403784439,1.,0.866025403784439,1.,0.866025403784439,
1.,0.866025403784439,1.,0.866025403784439,1.,0.866025403784439,1.,0.866025403784439,
1.,0.866025403784439,1.,0.866025403784439,1.,0.866025403784439,1.,0.866025403784439,
1.,0.866025403784439,1.,0.866025403784439,1.,0.866025403784439,1.,0.866025403784439,
1.,0.866025403784439,1.,0.866025403784439,1.,0.866025403784439,1.,0.866025403784439,
1.,0.866025403784439,1.,0.866025403784439,1.,0.866025403784439,1.,0.866025403784439,
1.,0.866025403784439,1.,0.866025403784439,1.,0.866025403784439,1.,0.866025403784439,
1.,0.866025403784439,1.,0.866025403784439,1.,0.866025403784439,1.,0.866025403784439,
1.,0.866025403784439,1.,0.866025403784439,1.,0.866025403784439,1.,0.866025403784439,
1.,0.866025403784439,1.,0.866025403784439,1.,0.866025403784439,1.,0.866025403784439,
1.,0.866025403784439,1.,0.866025403784439,1.,0.866025403784439,1.,0.866025403784439,
1.,0.866025403784439,1.,0.866025403784439,1.,0.866025403784439,1.,0.866025403784439,
1.,0.866025403784439,1.,0.866025403784439,1.,0.866025403784439,1.,0.866025403784439,
1.,0.866025403784439,1.,0.866025403784439,1.,0.866025403784439,1.,0.866025403784439,
1.,0.866025403784439,1.,0.866025403784439,1.,0.866025403784439,1.,0.866025403784439,
1.,0.866025403784439,1.,0.866025403784439,1.,0.866025403784439,1.,0.866025403784439,
1.,0.866025403784439,1.,0.866025403784439,1.,0.866025403784439,1.,0.866025403784439,
1.,0.866025403784439,1.,0.866025403784439,1.,0.866025403784439,1.,0.866025403784439,
1.,0.866025403784439,1.,0.866025403784439,1.,0.866025403784439,1.,0.866025403784439,
1.,0.866025403784439,1.,0.866025403784439,1.,0.866025403784439,1.,0.866025403784439,
1.,0.866025403784439,1.,0.866025403784439,1.,0.866025403784439,1.,0.866025403784439,
1.,0.866025403784439,1.,0.866025403784439,1.,0.866025403784439,1.,0.866025403784439,
1.,0.866025403784439,1.,0.866025403784439,1.,0.866025403784439,1.,0.866025403784439,
1.,0.866025403784439,1.,0.866025403784439,1.,0.866025403784439,1.,0.866025403784439,
1.,0.866025403784439,1.,0.866025403784439,1.,0.866025403784439,1.,0.866025403784439,
1.,0.866025403784439,1.,0.866025403784439,1.,0.866025403784439,1.,0.866025403784439,
1.,0.866025403784439,1.,0.866025403784439,1.,0.866025403784439,1.,0.866025403784439,
1.,0.866025403784439,1.,0.866025403784439,1.,0.866025403784439,1.,0.866025403784439,
1.,0.866025403784439,1.,0.866025403784439,1.,0.866025403784439,1.,0.866025403784439,
1.,0.866025403784439,1.,0.866025403784439,1.,0.866025403784439,1.,0.866025403784439,
1.,0.866025403784439,1.,0.866025403784439,1.,0.866025403784439,1.,0.866025403784439,
1.,0.866025403784439,1.,0.866025403784439,1.,0.866025403784439,1.,0.866025403784439,
1.,0.866025403784439,1.,0.866025403784439,1.,0.866025403784439,1.,0.866025403784439,
1.,0.866025403784439,1.,0.866025403784439,1.,0.866025403784439,1.,0.866025403784439,
1.,0.866025403784439,1.,0.866025403784439,1.,0.866025403784439,1.,0.866025403784439,
1.,0.866025403784439,1.,0.866025403784439,1.,0.866025403784439,1.,0.866025403784439,
1.,0.866025403784439,1.,0.866025403784439,1.,0.866025403784439,1.,0.866025403784439,
1.,0.866025403784439,1.,0.866025403784439,1.,0.866025403784439,1.,0.866025403784439,
1.,0.866025403784439,1.,0.866025403784439,1.,0.866025403784439,1.,0.866025403784439,
1.,0.866025403784439,1.,0.866025403784439,1.,0.866025403784439,1.,0.866025403784439,
1.,0.866025403784439,1.,0.866025403784439,1.,0.866025403784439,1.,0.866025403784439,
1.,0.866025403784439,1.,0.866025403784439,1.,0.866025403784439,1.,0.866025403784439,
1.,0.866025403784439,1.,0.866025403784439,1.,0.866025403784439,1.,0.866025403784439,
1.,0.866025403784439,1.,0.866025403784439,1.,0.866025403784439,1.,0.866025403784439,
1.,0.866025403784439,1.,0.866025403784439,1.,0.866025403784439,1.,0.866025403784439,
1.,0.866025403784439,1.,0.866025403784439,1.,0.866025403784439,1.,0.866025403784439,
1.,0.866025403784439,1.,0.866025403784439,1.,0.866025403784439,1.,0.866025403784439,
1.,0.866025403784439,1.,0.866025403784439,1.,0.866025403784439,1.,0.866025403784439,
1.,0.866025403784439,1.,0.866025403784439,1.,0.866025403784439,1.,0.866025403784439,
1.,0.866025403784439,1.,0.866025403784439,1.,0.866025403784439,1.,0.866025403784439,
1.,0.866025403784439,1.,0.866025403784439,1.,0.866025403784439,1.,0.866025403784439,
1.,0.866025403784439,1.,0.866025403784439,1.,0.866025403784439,1.,0.866025403784439,
1.,0.866025403784439,1.,0.866025403784439,1.,0.866025403784439,1.,0.866025403784439,
1.,0.866025403784439,1.,0.866025403784439,1.,0.866025403784439,1.,0.866025403784439,
1.,0.866025403784439,1.,0.866025403784439,1.,0.866025403784439,1.,0.866025403784439,
1.,0.866025403784439,1.,0.866025403784439,1.,0.866025403784439,1.,0.866025403784439,
1.,0.866025403784439,1.,0.866025403784439,1.,0.866025403784439,1.,0.866025403784439,
1.,0.866025403784439,1.,0.866025403784439,1.,0.866025403784439,1.,0.866025403784439,
1.,0.866025403784439,1.,0.866025403784439,1.,0.866025403784439,1.,0.866025403784439,
1.,0.866025403784439,1.,0.866025403784439,1.,0.866025403784439,1.,0.866025403784439,
1.,0.866025403784439,1.,0.866025403784439,1.,0.866025403784439,1.,0.866025403784439,
1.,0.866025403784439,1.,0.866025403784439,1.,0.866025403784439,1.,0.866025403784439,
1.,0.866025403784439,1.,0.866025403784439,1.,0.866025403784439,1.,0.866025403784439,
1.,0.866025403784439,1.,0.866025403784439,1.,0.866025403784439,1.,0.866025403784439,
1.,0.866025403784439,1.,0.866025403784439,1.,0.866025403784439,1.,0.866025403784439,
1.,0.866025403784439,1.,0.866025403784439,1.,0.866025403784439,1.,0.866025403784439,
1.,0.866025403784439,1.,0.866025403784439,1.,0.866025403784439,1.,0.866025403784439,
1.,0.866025403784439,1.,0.866025403784439,1.,0.866025403784439,1.,0.866025403784439,
1.,0.866025403784439,1.,0.866025403784439,1.,0.866025403784439,1.,0.866025403784439,
1.,0.866025403784439,1.,0.866025403784439,1.,0.866025403784439,1.,0.866025403784439,
1.,0.866025403784439,1.,0.866025403784439,1.,0.866025403784439,1.,0.866025403784439,
1.,0.866025403784439,1.,0.866025403784439,1.,0.866025403784439,1.,0.866025403784439,
1.,0.866025403784439,1.,0.866025403784439,1.,0.866025403784439,1.,0.866025403784439,
1.,0.866025403784439,1.,0.866025403784439,1.,0.866025403784439,1.,0.866025403784439,
1.,0.866025403784439,1.,0.866025403784439,1.,0.866025403784439,1.,0.866025403784439,
1.,0.866025403784439,1.,0.866025403784439,1.,0.866025403784439,1.,0.866025403784439,
1.,0.866025403784439,1.,0.866025403784439,1.,0.866025403784439,1.,0.866025403784439,
1.,0.866025403784439,1.,0.866025403784439,1.,0.866025403784439,1.,0.866025403784439,
1.,0.866025403784439,1.,0.866025403784439,1.,0.866025403784439,1.,0.866025403784439,
1.,0.866025403784439,1.,0.866025403784439,1.,0.866025403784439,1.,0.866025403784439,
1.,0.866025403784439,1.,0.866025403784439,1.,0.866025403784439,1.,0.866025403784439,
1.,0.866025403784439,1.,0.866025403784439,1.,0.866025403784439,1.,0.866025403784439,
1.,0.866025403784439,1.,0.866025403784439,1.,0.866025403784439,1.,0.866025403784439,
1.,0.866025403784439,1.,0.866025403784439,1.,0.866025403784439,1.,0.866025403784439,
1.,0.866025403784439,1.,0.866025403784439,1.,0.866025403784439,1.,0.866025403784439,
1.,0.866025403784439,1.,0.866025403784439,1.,0.866025403784439,1.,0.866025403784439,
1.,0.866025403784439,1.,0.866025403784439,1.,0.866025403784439,1.,0.866025403784439,
1.,0.866025403784439,1.,0.866025403784439,1.,0.866025403784439,1.,0.866025403784439,
1.,0.866025403784439,1.,0.866025403784439,1.,0.866025403784439,1.,0.866025403784439,
1.,0.866025403784439,1.,0.866025403784439,1.,0.866025403784439,1.,0.866025403784439,
1.,0.866025403784439,1.,0.866025403784439,1.,0.866025403784439,1.,0.866025403784439,
1.,0.866025403784439,1.,0.866025403784439,1.,0.866025403784439,1.,0.866025403784439,
1.,0.866025403784439,1.,0.866025403784439,1.,0.866025403784439,1.,0.866025403784439,
1.,0.866025403784439,1.,0.866025403784439,1.,0.866025403784439,1.,0.866025403784439,
1.,0.866025403784439,1.,0.866025403784439,1.,0.866025403784439,1.,0.866025403784439,
1.,0.866025403784439,1.,0.866025403784439,1.,0.866025403784439,1.,0.866025403784439,
1.,0.866025403784439,1.,0.866025403784439,1.,0.866025403784439,1.,0.866025403784439,
1.,0.866025403784439,1.,0.866025403784439,1.,0.866025403784439,1.,0.866025403784439,
1.,0.866025403784439,1.,0.866025403784439,1.,0.866025403784439,1.,0.866025403784439,
1.,0.866025403784439,1.,0.866025403784439,1.,0.866025403784439,1.,0.866025403784439,
1.,0.866025403784439,1.,0.866025403784439,1.,0.866025403784439,1.,0.866025403784439,
1.,0.866025403784439,1.,0.866025403784439,1.,0.866025403784439,1.,0.866025403784439,
1.,0.866025403784439,1.,0.866025403784439,1.,0.866025403784439,1.,0.866025403784439,
1.,0.866025403784439,1.,0.866025403784439,1.,0.866025403784439,1.,0.866025403784439,
1.,0.866025403784439,1.,0.866025403784439,1.,0.866025403784439,1.,0.866025403784439,
1.,0.866025403784439,1.,0.866025403784439,1.,0.866025403784439,1.,0.866025403784439,
1.,0.866025403784439,1.,0.866025403784439,1.,0.866025403784439,1.)))
REPRESENTATION_ITEM('')
SURFACE()
);
#179=(
BOUNDED_SURFACE()
B_SPLINE_SURFACE(3,2,((#32628,#32629,#32630,#32631,#32632,#32633,#32634,
#32635,#32636,#32637,#32638,#32639,#32640,#32641,#32642,#32643,#32644,#32645,
#32646,#32647,#32648,#32649,#32650,#32651,#32652,#32653,#32654,#32655,#32656,
#32657,#32658,#32659,#32660,#32661,#32662,#32663,#32664,#32665,#32666,#32667,
#32668,#32669,#32670,#32671,#32672,#32673,#32674,#32675,#32676,#32677,#32678,
#32679,#32680,#32681,#32682,#32683,#32684,#32685,#32686,#32687,#32688,#32689,
#32690,#32691,#32692,#32693,#32694,#32695,#32696,#32697,#32698,#32699,#32700,
#32701,#32702,#32703,#32704,#32705,#32706,#32707,#32708,#32709,#32710,#32711,
#32712,#32713,#32714,#32715,#32716,#32717,#32718,#32719,#32720,#32721,#32722,
#32723,#32724,#32725,#32726,#32727,#32728,#32729,#32730,#32731,#32732,#32733,
#32734,#32735,#32736,#32737,#32738,#32739,#32740,#32741,#32742,#32743,#32744,
#32745,#32746,#32747,#32748,#32749,#32750,#32751,#32752,#32753,#32754,#32755,
#32756,#32757,#32758,#32759,#32760,#32761,#32762,#32763,#32764,#32765,#32766,
#32767,#32768,#32769,#32770,#32771,#32772,#32773,#32774,#32775,#32776,#32777,
#32778,#32779,#32780,#32781,#32782,#32783,#32784,#32785,#32786,#32787,#32788,
#32789,#32790,#32791,#32792,#32793,#32794,#32795,#32796,#32797,#32798,#32799,
#32800,#32801,#32802,#32803,#32804,#32805,#32806,#32807,#32808,#32809,#32810,
#32811,#32812,#32813,#32814,#32815,#32816,#32817,#32818,#32819,#32820,#32821,
#32822,#32823,#32824,#32825,#32826,#32827,#32828,#32829,#32830,#32831,#32832,
#32833,#32834,#32835,#32836,#32837,#32838,#32839,#32840,#32841,#32842,#32843,
#32844,#32845,#32846,#32847,#32848,#32849,#32850,#32851,#32852,#32853,#32854,
#32855,#32856,#32857,#32858,#32859,#32860,#32861,#32862,#32863,#32864,#32865,
#32866,#32867,#32868,#32869,#32870,#32871,#32872,#32873,#32874,#32875,#32876,
#32877,#32878,#32879,#32880,#32881,#32882,#32883,#32884,#32885,#32886,#32887,
#32888,#32889,#32890,#32891,#32892,#32893,#32894,#32895,#32896,#32897,#32898,
#32899,#32900,#32901,#32902,#32903,#32904,#32905,#32906,#32907,#32908,#32909,
#32910,#32911,#32912,#32913,#32914,#32915,#32916,#32917,#32918,#32919,#32920,
#32921,#32922,#32923,#32924,#32925,#32926,#32927,#32928,#32929,#32930,#32931,
#32932,#32933,#32934,#32935,#32936,#32937,#32938,#32939,#32940,#32941,#32942,
#32943,#32944,#32945,#32946,#32947,#32948,#32949,#32950,#32951,#32952,#32953,
#32954,#32955,#32956,#32957,#32958,#32959,#32960,#32961,#32962,#32963,#32964,
#32965,#32966,#32967,#32968,#32969,#32970,#32971,#32972,#32973,#32974,#32975,
#32976,#32977,#32978,#32979,#32980,#32981,#32982,#32983,#32984,#32985,#32986,
#32987,#32988,#32989,#32990,#32991,#32992,#32993,#32994,#32995,#32996,#32997,
#32998,#32999,#33000,#33001,#33002,#33003,#33004,#33005,#33006,#33007,#33008,
#33009,#33010,#33011,#33012,#33013,#33014,#33015,#33016,#33017,#33018,#33019,
#33020,#33021,#33022,#33023,#33024,#33025,#33026,#33027,#33028,#33029,#33030,
#33031,#33032,#33033,#33034,#33035,#33036,#33037,#33038,#33039,#33040,#33041,
#33042,#33043,#33044,#33045,#33046,#33047,#33048,#33049,#33050,#33051,#33052,
#33053,#33054,#33055,#33056,#33057,#33058,#33059,#33060,#33061,#33062,#33063,
#33064,#33065,#33066,#33067,#33068,#33069,#33070,#33071,#33072,#33073,#33074,
#33075,#33076,#33077,#33078,#33079,#33080,#33081,#33082,#33083,#33084,#33085,
#33086,#33087,#33088,#33089,#33090,#33091,#33092,#33093,#33094,#33095,#33096,
#33097,#33098,#33099,#33100,#33101,#33102,#33103,#33104,#33105,#33106,#33107,
#33108,#33109,#33110,#33111,#33112,#33113,#33114,#33115,#33116,#33117,#33118,
#33119,#33120,#33121,#33122,#33123,#33124,#33125,#33126,#33127,#33128,#33129,
#33130,#33131,#33132,#33133,#33134,#33135,#33136,#33137,#33138,#33139,#33140,
#33141,#33142,#33143,#33144,#33145,#33146,#33147,#33148,#33149,#33150,#33151,
#33152,#33153,#33154,#33155,#33156,#33157,#33158,#33159,#33160,#33161,#33162,
#33163,#33164,#33165,#33166,#33167,#33168,#33169,#33170,#33171,#33172,#33173,
#33174,#33175,#33176,#33177,#33178,#33179,#33180,#33181,#33182,#33183,#33184,
#33185,#33186,#33187,#33188,#33189,#33190,#33191,#33192,#33193,#33194,#33195,
#33196,#33197,#33198,#33199,#33200,#33201,#33202,#33203,#33204,#33205,#33206,
#33207,#33208,#33209,#33210,#33211,#33212,#33213,#33214,#33215,#33216,#33217,
#33218,#33219,#33220,#33221,#33222,#33223,#33224,#33225,#33226,#33227,#33228,
#33229,#33230,#33231,#33232,#33233,#33234,#33235,#33236,#33237,#33238,#33239,
#33240,#33241,#33242,#33243,#33244,#33245,#33246,#33247,#33248,#33249,#33250,
#33251,#33252,#33253,#33254,#33255,#33256,#33257,#33258,#33259,#33260,#33261,
#33262,#33263,#33264,#33265,#33266,#33267,#33268,#33269,#33270,#33271,#33272,
#33273,#33274,#33275,#33276,#33277,#33278,#33279,#33280,#33281,#33282,#33283,
#33284,#33285,#33286,#33287,#33288,#33289,#33290,#33291,#33292,#33293,#33294,
#33295,#33296,#33297,#33298,#33299,#33300,#33301,#33302,#33303,#33304,#33305,
#33306,#33307,#33308,#33309,#33310,#33311,#33312,#33313,#33314,#33315,#33316,
#33317,#33318,#33319,#33320,#33321,#33322,#33323,#33324,#33325,#33326,#33327,
#33328,#33329,#33330,#33331,#33332,#33333,#33334,#33335,#33336,#33337,#33338,
#33339,#33340,#33341,#33342,#33343,#33344,#33345,#33346,#33347,#33348,#33349,
#33350,#33351,#33352,#33353,#33354,#33355,#33356,#33357,#33358,#33359,#33360,
#33361,#33362,#33363,#33364,#33365,#33366,#33367,#33368,#33369,#33370,#33371,
#33372,#33373,#33374,#33375,#33376,#33377,#33378,#33379,#33380,#33381,#33382,
#33383,#33384,#33385,#33386,#33387,#33388,#33389,#33390,#33391,#33392,#33393,
#33394,#33395,#33396,#33397,#33398,#33399,#33400,#33401,#33402,#33403,#33404,
#33405,#33406,#33407,#33408,#33409,#33410,#33411,#33412,#33413,#33414,#33415,
#33416,#33417,#33418,#33419,#33420,#33421,#33422,#33423,#33424,#33425,#33426,
#33427,#33428,#33429,#33430,#33431,#33432,#33433,#33434,#33435,#33436,#33437,
#33438,#33439,#33440,#33441,#33442,#33443,#33444,#33445,#33446,#33447,#33448,
#33449,#33450,#33451,#33452,#33453,#33454,#33455,#33456,#33457,#33458,#33459,
#33460,#33461,#33462,#33463,#33464,#33465,#33466,#33467,#33468,#33469,#33470,
#33471,#33472,#33473,#33474,#33475,#33476,#33477,#33478,#33479,#33480,#33481,
#33482,#33483,#33484,#33485,#33486,#33487,#33488,#33489,#33490,#33491,#33492,
#33493,#33494,#33495,#33496,#33497,#33498,#33499,#33500,#33501,#33502,#33503,
#33504,#33505,#33506,#33507,#33508,#33509,#33510,#33511,#33512,#33513,#33514,
#33515,#33516,#33517,#33518,#33519,#33520,#33521,#33522,#33523,#33524,#33525,
#33526,#33527,#33528,#33529,#33530,#33531,#33532,#33533,#33534,#33535,#33536,
#33537,#33538,#33539,#33540,#33541,#33542,#33543,#33544,#33545,#33546,#33547,
#33548,#33549,#33550,#33551,#33552,#33553,#33554,#33555,#33556,#33557,#33558,
#33559,#33560,#33561,#33562,#33563,#33564,#33565,#33566,#33567,#33568,#33569,
#33570,#33571,#33572,#33573,#33574,#33575,#33576,#33577,#33578,#33579,#33580,
#33581,#33582,#33583,#33584,#33585,#33586,#33587,#33588,#33589,#33590,#33591,
#33592,#33593,#33594,#33595,#33596,#33597,#33598,#33599,#33600),(#33601,
#33602,#33603,#33604,#33605,#33606,#33607,#33608,#33609,#33610,#33611,#33612,
#33613,#33614,#33615,#33616,#33617,#33618,#33619,#33620,#33621,#33622,#33623,
#33624,#33625,#33626,#33627,#33628,#33629,#33630,#33631,#33632,#33633,#33634,
#33635,#33636,#33637,#33638,#33639,#33640,#33641,#33642,#33643,#33644,#33645,
#33646,#33647,#33648,#33649,#33650,#33651,#33652,#33653,#33654,#33655,#33656,
#33657,#33658,#33659,#33660,#33661,#33662,#33663,#33664,#33665,#33666,#33667,
#33668,#33669,#33670,#33671,#33672,#33673,#33674,#33675,#33676,#33677,#33678,
#33679,#33680,#33681,#33682,#33683,#33684,#33685,#33686,#33687,#33688,#33689,
#33690,#33691,#33692,#33693,#33694,#33695,#33696,#33697,#33698,#33699,#33700,
#33701,#33702,#33703,#33704,#33705,#33706,#33707,#33708,#33709,#33710,#33711,
#33712,#33713,#33714,#33715,#33716,#33717,#33718,#33719,#33720,#33721,#33722,
#33723,#33724,#33725,#33726,#33727,#33728,#33729,#33730,#33731,#33732,#33733,
#33734,#33735,#33736,#33737,#33738,#33739,#33740,#33741,#33742,#33743,#33744,
#33745,#33746,#33747,#33748,#33749,#33750,#33751,#33752,#33753,#33754,#33755,
#33756,#33757,#33758,#33759,#33760,#33761,#33762,#33763,#33764,#33765,#33766,
#33767,#33768,#33769,#33770,#33771,#33772,#33773,#33774,#33775,#33776,#33777,
#33778,#33779,#33780,#33781,#33782,#33783,#33784,#33785,#33786,#33787,#33788,
#33789,#33790,#33791,#33792,#33793,#33794,#33795,#33796,#33797,#33798,#33799,
#33800,#33801,#33802,#33803,#33804,#33805,#33806,#33807,#33808,#33809,#33810,
#33811,#33812,#33813,#33814,#33815,#33816,#33817,#33818,#33819,#33820,#33821,
#33822,#33823,#33824,#33825,#33826,#33827,#33828,#33829,#33830,#33831,#33832,
#33833,#33834,#33835,#33836,#33837,#33838,#33839,#33840,#33841,#33842,#33843,
#33844,#33845,#33846,#33847,#33848,#33849,#33850,#33851,#33852,#33853,#33854,
#33855,#33856,#33857,#33858,#33859,#33860,#33861,#33862,#33863,#33864,#33865,
#33866,#33867,#33868,#33869,#33870,#33871,#33872,#33873,#33874,#33875,#33876,
#33877,#33878,#33879,#33880,#33881,#33882,#33883,#33884,#33885,#33886,#33887,
#33888,#33889,#33890,#33891,#33892,#33893,#33894,#33895,#33896,#33897,#33898,
#33899,#33900,#33901,#33902,#33903,#33904,#33905,#33906,#33907,#33908,#33909,
#33910,#33911,#33912,#33913,#33914,#33915,#33916,#33917,#33918,#33919,#33920,
#33921,#33922,#33923,#33924,#33925,#33926,#33927,#33928,#33929,#33930,#33931,
#33932,#33933,#33934,#33935,#33936,#33937,#33938,#33939,#33940,#33941,#33942,
#33943,#33944,#33945,#33946,#33947,#33948,#33949,#33950,#33951,#33952,#33953,
#33954,#33955,#33956,#33957,#33958,#33959,#33960,#33961,#33962,#33963,#33964,
#33965,#33966,#33967,#33968,#33969,#33970,#33971,#33972,#33973,#33974,#33975,
#33976,#33977,#33978,#33979,#33980,#33981,#33982,#33983,#33984,#33985,#33986,
#33987,#33988,#33989,#33990,#33991,#33992,#33993,#33994,#33995,#33996,#33997,
#33998,#33999,#34000,#34001,#34002,#34003,#34004,#34005,#34006,#34007,#34008,
#34009,#34010,#34011,#34012,#34013,#34014,#34015,#34016,#34017,#34018,#34019,
#34020,#34021,#34022,#34023,#34024,#34025,#34026,#34027,#34028,#34029,#34030,
#34031,#34032,#34033,#34034,#34035,#34036,#34037,#34038,#34039,#34040,#34041,
#34042,#34043,#34044,#34045,#34046,#34047,#34048,#34049,#34050,#34051,#34052,
#34053,#34054,#34055,#34056,#34057,#34058,#34059,#34060,#34061,#34062,#34063,
#34064,#34065,#34066,#34067,#34068,#34069,#34070,#34071,#34072,#34073,#34074,
#34075,#34076,#34077,#34078,#34079,#34080,#34081,#34082,#34083,#34084,#34085,
#34086,#34087,#34088,#34089,#34090,#34091,#34092,#34093,#34094,#34095,#34096,
#34097,#34098,#34099,#34100,#34101,#34102,#34103,#34104,#34105,#34106,#34107,
#34108,#34109,#34110,#34111,#34112,#34113,#34114,#34115,#34116,#34117,#34118,
#34119,#34120,#34121,#34122,#34123,#34124,#34125,#34126,#34127,#34128,#34129,
#34130,#34131,#34132,#34133,#34134,#34135,#34136,#34137,#34138,#34139,#34140,
#34141,#34142,#34143,#34144,#34145,#34146,#34147,#34148,#34149,#34150,#34151,
#34152,#34153,#34154,#34155,#34156,#34157,#34158,#34159,#34160,#34161,#34162,
#34163,#34164,#34165,#34166,#34167,#34168,#34169,#34170,#34171,#34172,#34173,
#34174,#34175,#34176,#34177,#34178,#34179,#34180,#34181,#34182,#34183,#34184,
#34185,#34186,#34187,#34188,#34189,#34190,#34191,#34192,#34193,#34194,#34195,
#34196,#34197,#34198,#34199,#34200,#34201,#34202,#34203,#34204,#34205,#34206,
#34207,#34208,#34209,#34210,#34211,#34212,#34213,#34214,#34215,#34216,#34217,
#34218,#34219,#34220,#34221,#34222,#34223,#34224,#34225,#34226,#34227,#34228,
#34229,#34230,#34231,#34232,#34233,#34234,#34235,#34236,#34237,#34238,#34239,
#34240,#34241,#34242,#34243,#34244,#34245,#34246,#34247,#34248,#34249,#34250,
#34251,#34252,#34253,#34254,#34255,#34256,#34257,#34258,#34259,#34260,#34261,
#34262,#34263,#34264,#34265,#34266,#34267,#34268,#34269,#34270,#34271,#34272,
#34273,#34274,#34275,#34276,#34277,#34278,#34279,#34280,#34281,#34282,#34283,
#34284,#34285,#34286,#34287,#34288,#34289,#34290,#34291,#34292,#34293,#34294,
#34295,#34296,#34297,#34298,#34299,#34300,#34301,#34302,#34303,#34304,#34305,
#34306,#34307,#34308,#34309,#34310,#34311,#34312,#34313,#34314,#34315,#34316,
#34317,#34318,#34319,#34320,#34321,#34322,#34323,#34324,#34325,#34326,#34327,
#34328,#34329,#34330,#34331,#34332,#34333,#34334,#34335,#34336,#34337,#34338,
#34339,#34340,#34341,#34342,#34343,#34344,#34345,#34346,#34347,#34348,#34349,
#34350,#34351,#34352,#34353,#34354,#34355,#34356,#34357,#34358,#34359,#34360,
#34361,#34362,#34363,#34364,#34365,#34366,#34367,#34368,#34369,#34370,#34371,
#34372,#34373,#34374,#34375,#34376,#34377,#34378,#34379,#34380,#34381,#34382,
#34383,#34384,#34385,#34386,#34387,#34388,#34389,#34390,#34391,#34392,#34393,
#34394,#34395,#34396,#34397,#34398,#34399,#34400,#34401,#34402,#34403,#34404,
#34405,#34406,#34407,#34408,#34409,#34410,#34411,#34412,#34413,#34414,#34415,
#34416,#34417,#34418,#34419,#34420,#34421,#34422,#34423,#34424,#34425,#34426,
#34427,#34428,#34429,#34430,#34431,#34432,#34433,#34434,#34435,#34436,#34437,
#34438,#34439,#34440,#34441,#34442,#34443,#34444,#34445,#34446,#34447,#34448,
#34449,#34450,#34451,#34452,#34453,#34454,#34455,#34456,#34457,#34458,#34459,
#34460,#34461,#34462,#34463,#34464,#34465,#34466,#34467,#34468,#34469,#34470,
#34471,#34472,#34473,#34474,#34475,#34476,#34477,#34478,#34479,#34480,#34481,
#34482,#34483,#34484,#34485,#34486,#34487,#34488,#34489,#34490,#34491,#34492,
#34493,#34494,#34495,#34496,#34497,#34498,#34499,#34500,#34501,#34502,#34503,
#34504,#34505,#34506,#34507,#34508,#34509,#34510,#34511,#34512,#34513,#34514,
#34515,#34516,#34517,#34518,#34519,#34520,#34521,#34522,#34523,#34524,#34525,
#34526,#34527,#34528,#34529,#34530,#34531,#34532,#34533,#34534,#34535,#34536,
#34537,#34538,#34539,#34540,#34541,#34542,#34543,#34544,#34545,#34546,#34547,
#34548,#34549,#34550,#34551,#34552,#34553,#34554,#34555,#34556,#34557,#34558,
#34559,#34560,#34561,#34562,#34563,#34564,#34565,#34566,#34567,#34568,#34569,
#34570,#34571,#34572,#34573),(#34574,#34575,#34576,#34577,#34578,#34579,
#34580,#34581,#34582,#34583,#34584,#34585,#34586,#34587,#34588,#34589,#34590,
#34591,#34592,#34593,#34594,#34595,#34596,#34597,#34598,#34599,#34600,#34601,
#34602,#34603,#34604,#34605,#34606,#34607,#34608,#34609,#34610,#34611,#34612,
#34613,#34614,#34615,#34616,#34617,#34618,#34619,#34620,#34621,#34622,#34623,
#34624,#34625,#34626,#34627,#34628,#34629,#34630,#34631,#34632,#34633,#34634,
#34635,#34636,#34637,#34638,#34639,#34640,#34641,#34642,#34643,#34644,#34645,
#34646,#34647,#34648,#34649,#34650,#34651,#34652,#34653,#34654,#34655,#34656,
#34657,#34658,#34659,#34660,#34661,#34662,#34663,#34664,#34665,#34666,#34667,
#34668,#34669,#34670,#34671,#34672,#34673,#34674,#34675,#34676,#34677,#34678,
#34679,#34680,#34681,#34682,#34683,#34684,#34685,#34686,#34687,#34688,#34689,
#34690,#34691,#34692,#34693,#34694,#34695,#34696,#34697,#34698,#34699,#34700,
#34701,#34702,#34703,#34704,#34705,#34706,#34707,#34708,#34709,#34710,#34711,
#34712,#34713,#34714,#34715,#34716,#34717,#34718,#34719,#34720,#34721,#34722,
#34723,#34724,#34725,#34726,#34727,#34728,#34729,#34730,#34731,#34732,#34733,
#34734,#34735,#34736,#34737,#34738,#34739,#34740,#34741,#34742,#34743,#34744,
#34745,#34746,#34747,#34748,#34749,#34750,#34751,#34752,#34753,#34754,#34755,
#34756,#34757,#34758,#34759,#34760,#34761,#34762,#34763,#34764,#34765,#34766,
#34767,#34768,#34769,#34770,#34771,#34772,#34773,#34774,#34775,#34776,#34777,
#34778,#34779,#34780,#34781,#34782,#34783,#34784,#34785,#34786,#34787,#34788,
#34789,#34790,#34791,#34792,#34793,#34794,#34795,#34796,#34797,#34798,#34799,
#34800,#34801,#34802,#34803,#34804,#34805,#34806,#34807,#34808,#34809,#34810,
#34811,#34812,#34813,#34814,#34815,#34816,#34817,#34818,#34819,#34820,#34821,
#34822,#34823,#34824,#34825,#34826,#34827,#34828,#34829,#34830,#34831,#34832,
#34833,#34834,#34835,#34836,#34837,#34838,#34839,#34840,#34841,#34842,#34843,
#34844,#34845,#34846,#34847,#34848,#34849,#34850,#34851,#34852,#34853,#34854,
#34855,#34856,#34857,#34858,#34859,#34860,#34861,#34862,#34863,#34864,#34865,
#34866,#34867,#34868,#34869,#34870,#34871,#34872,#34873,#34874,#34875,#34876,
#34877,#34878,#34879,#34880,#34881,#34882,#34883,#34884,#34885,#34886,#34887,
#34888,#34889,#34890,#34891,#34892,#34893,#34894,#34895,#34896,#34897,#34898,
#34899,#34900,#34901,#34902,#34903,#34904,#34905,#34906,#34907,#34908,#34909,
#34910,#34911,#34912,#34913,#34914,#34915,#34916,#34917,#34918,#34919,#34920,
#34921,#34922,#34923,#34924,#34925,#34926,#34927,#34928,#34929,#34930,#34931,
#34932,#34933,#34934,#34935,#34936,#34937,#34938,#34939,#34940,#34941,#34942,
#34943,#34944,#34945,#34946,#34947,#34948,#34949,#34950,#34951,#34952,#34953,
#34954,#34955,#34956,#34957,#34958,#34959,#34960,#34961,#34962,#34963,#34964,
#34965,#34966,#34967,#34968,#34969,#34970,#34971,#34972,#34973,#34974,#34975,
#34976,#34977,#34978,#34979,#34980,#34981,#34982,#34983,#34984,#34985,#34986,
#34987,#34988,#34989,#34990,#34991,#34992,#34993,#34994,#34995,#34996,#34997,
#34998,#34999,#35000,#35001,#35002,#35003,#35004,#35005,#35006,#35007,#35008,
#35009,#35010,#35011,#35012,#35013,#35014,#35015,#35016,#35017,#35018,#35019,
#35020,#35021,#35022,#35023,#35024,#35025,#35026,#35027,#35028,#35029,#35030,
#35031,#35032,#35033,#35034,#35035,#35036,#35037,#35038,#35039,#35040,#35041,
#35042,#35043,#35044,#35045,#35046,#35047,#35048,#35049,#35050,#35051,#35052,
#35053,#35054,#35055,#35056,#35057,#35058,#35059,#35060,#35061,#35062,#35063,
#35064,#35065,#35066,#35067,#35068,#35069,#35070,#35071,#35072,#35073,#35074,
#35075,#35076,#35077,#35078,#35079,#35080,#35081,#35082,#35083,#35084,#35085,
#35086,#35087,#35088,#35089,#35090,#35091,#35092,#35093,#35094,#35095,#35096,
#35097,#35098,#35099,#35100,#35101,#35102,#35103,#35104,#35105,#35106,#35107,
#35108,#35109,#35110,#35111,#35112,#35113,#35114,#35115,#35116,#35117,#35118,
#35119,#35120,#35121,#35122,#35123,#35124,#35125,#35126,#35127,#35128,#35129,
#35130,#35131,#35132,#35133,#35134,#35135,#35136,#35137,#35138,#35139,#35140,
#35141,#35142,#35143,#35144,#35145,#35146,#35147,#35148,#35149,#35150,#35151,
#35152,#35153,#35154,#35155,#35156,#35157,#35158,#35159,#35160,#35161,#35162,
#35163,#35164,#35165,#35166,#35167,#35168,#35169,#35170,#35171,#35172,#35173,
#35174,#35175,#35176,#35177,#35178,#35179,#35180,#35181,#35182,#35183,#35184,
#35185,#35186,#35187,#35188,#35189,#35190,#35191,#35192,#35193,#35194,#35195,
#35196,#35197,#35198,#35199,#35200,#35201,#35202,#35203,#35204,#35205,#35206,
#35207,#35208,#35209,#35210,#35211,#35212,#35213,#35214,#35215,#35216,#35217,
#35218,#35219,#35220,#35221,#35222,#35223,#35224,#35225,#35226,#35227,#35228,
#35229,#35230,#35231,#35232,#35233,#35234,#35235,#35236,#35237,#35238,#35239,
#35240,#35241,#35242,#35243,#35244,#35245,#35246,#35247,#35248,#35249,#35250,
#35251,#35252,#35253,#35254,#35255,#35256,#35257,#35258,#35259,#35260,#35261,
#35262,#35263,#35264,#35265,#35266,#35267,#35268,#35269,#35270,#35271,#35272,
#35273,#35274,#35275,#35276,#35277,#35278,#35279,#35280,#35281,#35282,#35283,
#35284,#35285,#35286,#35287,#35288,#35289,#35290,#35291,#35292,#35293,#35294,
#35295,#35296,#35297,#35298,#35299,#35300,#35301,#35302,#35303,#35304,#35305,
#35306,#35307,#35308,#35309,#35310,#35311,#35312,#35313,#35314,#35315,#35316,
#35317,#35318,#35319,#35320,#35321,#35322,#35323,#35324,#35325,#35326,#35327,
#35328,#35329,#35330,#35331,#35332,#35333,#35334,#35335,#35336,#35337,#35338,
#35339,#35340,#35341,#35342,#35343,#35344,#35345,#35346,#35347,#35348,#35349,
#35350,#35351,#35352,#35353,#35354,#35355,#35356,#35357,#35358,#35359,#35360,
#35361,#35362,#35363,#35364,#35365,#35366,#35367,#35368,#35369,#35370,#35371,
#35372,#35373,#35374,#35375,#35376,#35377,#35378,#35379,#35380,#35381,#35382,
#35383,#35384,#35385,#35386,#35387,#35388,#35389,#35390,#35391,#35392,#35393,
#35394,#35395,#35396,#35397,#35398,#35399,#35400,#35401,#35402,#35403,#35404,
#35405,#35406,#35407,#35408,#35409,#35410,#35411,#35412,#35413,#35414,#35415,
#35416,#35417,#35418,#35419,#35420,#35421,#35422,#35423,#35424,#35425,#35426,
#35427,#35428,#35429,#35430,#35431,#35432,#35433,#35434,#35435,#35436,#35437,
#35438,#35439,#35440,#35441,#35442,#35443,#35444,#35445,#35446,#35447,#35448,
#35449,#35450,#35451,#35452,#35453,#35454,#35455,#35456,#35457,#35458,#35459,
#35460,#35461,#35462,#35463,#35464,#35465,#35466,#35467,#35468,#35469,#35470,
#35471,#35472,#35473,#35474,#35475,#35476,#35477,#35478,#35479,#35480,#35481,
#35482,#35483,#35484,#35485,#35486,#35487,#35488,#35489,#35490,#35491,#35492,
#35493,#35494,#35495,#35496,#35497,#35498,#35499,#35500,#35501,#35502,#35503,
#35504,#35505,#35506,#35507,#35508,#35509,#35510,#35511,#35512,#35513,#35514,
#35515,#35516,#35517,#35518,#35519,#35520,#35521,#35522,#35523,#35524,#35525,
#35526,#35527,#35528,#35529,#35530,#35531,#35532,#35533,#35534,#35535,#35536,
#35537,#35538,#35539,#35540,#35541,#35542,#35543,#35544,#35545,#35546),
(#35547,#35548,#35549,#35550,#35551,#35552,#35553,#35554,#35555,#35556,
#35557,#35558,#35559,#35560,#35561,#35562,#35563,#35564,#35565,#35566,#35567,
#35568,#35569,#35570,#35571,#35572,#35573,#35574,#35575,#35576,#35577,#35578,
#35579,#35580,#35581,#35582,#35583,#35584,#35585,#35586,#35587,#35588,#35589,
#35590,#35591,#35592,#35593,#35594,#35595,#35596,#35597,#35598,#35599,#35600,
#35601,#35602,#35603,#35604,#35605,#35606,#35607,#35608,#35609,#35610,#35611,
#35612,#35613,#35614,#35615,#35616,#35617,#35618,#35619,#35620,#35621,#35622,
#35623,#35624,#35625,#35626,#35627,#35628,#35629,#35630,#35631,#35632,#35633,
#35634,#35635,#35636,#35637,#35638,#35639,#35640,#35641,#35642,#35643,#35644,
#35645,#35646,#35647,#35648,#35649,#35650,#35651,#35652,#35653,#35654,#35655,
#35656,#35657,#35658,#35659,#35660,#35661,#35662,#35663,#35664,#35665,#35666,
#35667,#35668,#35669,#35670,#35671,#35672,#35673,#35674,#35675,#35676,#35677,
#35678,#35679,#35680,#35681,#35682,#35683,#35684,#35685,#35686,#35687,#35688,
#35689,#35690,#35691,#35692,#35693,#35694,#35695,#35696,#35697,#35698,#35699,
#35700,#35701,#35702,#35703,#35704,#35705,#35706,#35707,#35708,#35709,#35710,
#35711,#35712,#35713,#35714,#35715,#35716,#35717,#35718,#35719,#35720,#35721,
#35722,#35723,#35724,#35725,#35726,#35727,#35728,#35729,#35730,#35731,#35732,
#35733,#35734,#35735,#35736,#35737,#35738,#35739,#35740,#35741,#35742,#35743,
#35744,#35745,#35746,#35747,#35748,#35749,#35750,#35751,#35752,#35753,#35754,
#35755,#35756,#35757,#35758,#35759,#35760,#35761,#35762,#35763,#35764,#35765,
#35766,#35767,#35768,#35769,#35770,#35771,#35772,#35773,#35774,#35775,#35776,
#35777,#35778,#35779,#35780,#35781,#35782,#35783,#35784,#35785,#35786,#35787,
#35788,#35789,#35790,#35791,#35792,#35793,#35794,#35795,#35796,#35797,#35798,
#35799,#35800,#35801,#35802,#35803,#35804,#35805,#35806,#35807,#35808,#35809,
#35810,#35811,#35812,#35813,#35814,#35815,#35816,#35817,#35818,#35819,#35820,
#35821,#35822,#35823,#35824,#35825,#35826,#35827,#35828,#35829,#35830,#35831,
#35832,#35833,#35834,#35835,#35836,#35837,#35838,#35839,#35840,#35841,#35842,
#35843,#35844,#35845,#35846,#35847,#35848,#35849,#35850,#35851,#35852,#35853,
#35854,#35855,#35856,#35857,#35858,#35859,#35860,#35861,#35862,#35863,#35864,
#35865,#35866,#35867,#35868,#35869,#35870,#35871,#35872,#35873,#35874,#35875,
#35876,#35877,#35878,#35879,#35880,#35881,#35882,#35883,#35884,#35885,#35886,
#35887,#35888,#35889,#35890,#35891,#35892,#35893,#35894,#35895,#35896,#35897,
#35898,#35899,#35900,#35901,#35902,#35903,#35904,#35905,#35906,#35907,#35908,
#35909,#35910,#35911,#35912,#35913,#35914,#35915,#35916,#35917,#35918,#35919,
#35920,#35921,#35922,#35923,#35924,#35925,#35926,#35927,#35928,#35929,#35930,
#35931,#35932,#35933,#35934,#35935,#35936,#35937,#35938,#35939,#35940,#35941,
#35942,#35943,#35944,#35945,#35946,#35947,#35948,#35949,#35950,#35951,#35952,
#35953,#35954,#35955,#35956,#35957,#35958,#35959,#35960,#35961,#35962,#35963,
#35964,#35965,#35966,#35967,#35968,#35969,#35970,#35971,#35972,#35973,#35974,
#35975,#35976,#35977,#35978,#35979,#35980,#35981,#35982,#35983,#35984,#35985,
#35986,#35987,#35988,#35989,#35990,#35991,#35992,#35993,#35994,#35995,#35996,
#35997,#35998,#35999,#36000,#36001,#36002,#36003,#36004,#36005,#36006,#36007,
#36008,#36009,#36010,#36011,#36012,#36013,#36014,#36015,#36016,#36017,#36018,
#36019,#36020,#36021,#36022,#36023,#36024,#36025,#36026,#36027,#36028,#36029,
#36030,#36031,#36032,#36033,#36034,#36035,#36036,#36037,#36038,#36039,#36040,
#36041,#36042,#36043,#36044,#36045,#36046,#36047,#36048,#36049,#36050,#36051,
#36052,#36053,#36054,#36055,#36056,#36057,#36058,#36059,#36060,#36061,#36062,
#36063,#36064,#36065,#36066,#36067,#36068,#36069,#36070,#36071,#36072,#36073,
#36074,#36075,#36076,#36077,#36078,#36079,#36080,#36081,#36082,#36083,#36084,
#36085,#36086,#36087,#36088,#36089,#36090,#36091,#36092,#36093,#36094,#36095,
#36096,#36097,#36098,#36099,#36100,#36101,#36102,#36103,#36104,#36105,#36106,
#36107,#36108,#36109,#36110,#36111,#36112,#36113,#36114,#36115,#36116,#36117,
#36118,#36119,#36120,#36121,#36122,#36123,#36124,#36125,#36126,#36127,#36128,
#36129,#36130,#36131,#36132,#36133,#36134,#36135,#36136,#36137,#36138,#36139,
#36140,#36141,#36142,#36143,#36144,#36145,#36146,#36147,#36148,#36149,#36150,
#36151,#36152,#36153,#36154,#36155,#36156,#36157,#36158,#36159,#36160,#36161,
#36162,#36163,#36164,#36165,#36166,#36167,#36168,#36169,#36170,#36171,#36172,
#36173,#36174,#36175,#36176,#36177,#36178,#36179,#36180,#36181,#36182,#36183,
#36184,#36185,#36186,#36187,#36188,#36189,#36190,#36191,#36192,#36193,#36194,
#36195,#36196,#36197,#36198,#36199,#36200,#36201,#36202,#36203,#36204,#36205,
#36206,#36207,#36208,#36209,#36210,#36211,#36212,#36213,#36214,#36215,#36216,
#36217,#36218,#36219,#36220,#36221,#36222,#36223,#36224,#36225,#36226,#36227,
#36228,#36229,#36230,#36231,#36232,#36233,#36234,#36235,#36236,#36237,#36238,
#36239,#36240,#36241,#36242,#36243,#36244,#36245,#36246,#36247,#36248,#36249,
#36250,#36251,#36252,#36253,#36254,#36255,#36256,#36257,#36258,#36259,#36260,
#36261,#36262,#36263,#36264,#36265,#36266,#36267,#36268,#36269,#36270,#36271,
#36272,#36273,#36274,#36275,#36276,#36277,#36278,#36279,#36280,#36281,#36282,
#36283,#36284,#36285,#36286,#36287,#36288,#36289,#36290,#36291,#36292,#36293,
#36294,#36295,#36296,#36297,#36298,#36299,#36300,#36301,#36302,#36303,#36304,
#36305,#36306,#36307,#36308,#36309,#36310,#36311,#36312,#36313,#36314,#36315,
#36316,#36317,#36318,#36319,#36320,#36321,#36322,#36323,#36324,#36325,#36326,
#36327,#36328,#36329,#36330,#36331,#36332,#36333,#36334,#36335,#36336,#36337,
#36338,#36339,#36340,#36341,#36342,#36343,#36344,#36345,#36346,#36347,#36348,
#36349,#36350,#36351,#36352,#36353,#36354,#36355,#36356,#36357,#36358,#36359,
#36360,#36361,#36362,#36363,#36364,#36365,#36366,#36367,#36368,#36369,#36370,
#36371,#36372,#36373,#36374,#36375,#36376,#36377,#36378,#36379,#36380,#36381,
#36382,#36383,#36384,#36385,#36386,#36387,#36388,#36389,#36390,#36391,#36392,
#36393,#36394,#36395,#36396,#36397,#36398,#36399,#36400,#36401,#36402,#36403,
#36404,#36405,#36406,#36407,#36408,#36409,#36410,#36411,#36412,#36413,#36414,
#36415,#36416,#36417,#36418,#36419,#36420,#36421,#36422,#36423,#36424,#36425,
#36426,#36427,#36428,#36429,#36430,#36431,#36432,#36433,#36434,#36435,#36436,
#36437,#36438,#36439,#36440,#36441,#36442,#36443,#36444,#36445,#36446,#36447,
#36448,#36449,#36450,#36451,#36452,#36453,#36454,#36455,#36456,#36457,#36458,
#36459,#36460,#36461,#36462,#36463,#36464,#36465,#36466,#36467,#36468,#36469,
#36470,#36471,#36472,#36473,#36474,#36475,#36476,#36477,#36478,#36479,#36480,
#36481,#36482,#36483,#36484,#36485,#36486,#36487,#36488,#36489,#36490,#36491,
#36492,#36493,#36494,#36495,#36496,#36497,#36498,#36499,#36500,#36501,#36502,
#36503,#36504,#36505,#36506,#36507,#36508,#36509,#36510,#36511,#36512,#36513,
#36514,#36515,#36516,#36517,#36518,#36519)),.UNSPECIFIED.,.F.,.F.,.F.)
B_SPLINE_SURFACE_WITH_KNOTS((4,4),(3,2,2,2,2,2,2,2,2,2,2,2,2,2,2,2,2,2,
2,2,2,2,2,2,2,2,2,2,2,2,2,2,2,2,2,2,2,2,2,2,2,2,2,2,2,2,2,2,2,2,2,2,2,2,
2,2,2,2,2,2,2,2,2,2,2,2,2,2,2,2,2,2,2,2,2,2,2,2,2,2,2,2,2,2,2,2,2,2,2,2,
2,2,2,2,2,2,2,2,2,2,2,2,2,2,2,2,2,2,2,2,2,2,2,2,2,2,2,2,2,2,2,2,2,2,2,2,
2,2,2,2,2,2,2,2,2,2,2,2,2,2,2,2,2,2,2,2,2,2,2,2,2,2,2,2,2,2,2,2,2,2,2,2,
2,2,2,2,2,2,2,2,2,2,2,2,2,2,2,2,2,2,2,2,2,2,2,2,2,2,2,2,2,2,2,2,2,2,2,2,
2,2,2,2,2,2,2,2,2,2,2,2,2,2,2,2,2,2,2,2,2,2,2,2,2,2,2,2,2,2,2,2,2,2,2,2,
2,2,2,2,2,2,2,2,2,2,2,2,2,2,2,2,2,2,2,2,2,2,2,2,2,2,2,2,2,2,2,2,2,2,2,2,
2,2,2,2,2,2,2,2,2,2,2,2,2,2,2,2,2,2,2,2,2,2,2,2,2,2,2,2,2,2,2,2,2,2,2,2,
2,2,2,2,2,2,2,2,2,2,2,2,2,2,2,2,2,2,2,2,2,2,2,2,2,2,2,2,2,2,2,2,2,2,2,2,
2,2,2,2,2,2,2,2,2,2,2,2,2,2,2,2,2,2,2,2,2,2,2,2,2,2,2,2,2,2,2,2,2,2,2,2,
2,2,2,2,2,2,2,2,2,2,2,2,2,2,2,2,2,2,2,2,2,2,2,2,2,2,2,2,2,2,2,2,2,2,2,2,
2,2,2,2,2,2,2,2,2,2,2,2,2,2,2,2,2,2,2,2,2,2,2,2,2,2,2,2,2,2,2,2,2,2,2,2,
2,2,2,2,2,2,2,2,2,2,2,2,2,2,2,2,2,2,2,2,2,2,2,2,2,2,2,2,2,2,2,2,2,2,2,2,
3),(0.,1.),(0.,0.00205761316872428,0.00411522633744856,0.00617283950617284,
0.00823045267489712,0.0102880658436214,0.0123456790123457,0.01440329218107,
0.0164609053497942,0.0185185185185185,0.0205761316872428,0.0226337448559671,
0.0246913580246914,0.0267489711934156,0.0288065843621399,0.0308641975308642,
0.0329218106995885,0.0349794238683128,0.037037037037037,0.0390946502057613,
0.0411522633744856,0.0432098765432099,0.0452674897119342,0.0473251028806584,
0.0493827160493827,0.051440329218107,0.0534979423868313,0.0555555555555556,
0.0576131687242798,0.0596707818930041,0.0617283950617284,0.0637860082304527,
0.065843621399177,0.0679012345679012,0.0699588477366255,0.0720164609053498,
0.0740740740740741,0.0761316872427984,0.0781893004115226,0.0802469135802469,
0.0823045267489712,0.0843621399176955,0.0864197530864197,0.088477366255144,
0.0905349794238683,0.0925925925925926,0.0946502057613169,0.0967078189300412,
0.0987654320987654,0.10082304526749,0.102880658436214,0.104938271604938,
0.106995884773663,0.109053497942387,0.111111111111111,0.113168724279835,
0.11522633744856,0.117283950617284,0.119341563786008,0.121399176954733,
0.123456790123457,0.125514403292181,0.127572016460905,0.12962962962963,
0.131687242798354,0.133744855967078,0.135802469135802,0.137860082304527,
0.139917695473251,0.141975308641975,0.1440329218107,0.146090534979424,0.148148148148148,
0.150205761316872,0.152263374485597,0.154320987654321,0.156378600823045,
0.15843621399177,0.160493827160494,0.162551440329218,0.164609053497942,
0.166666666666667,0.168724279835391,0.170781893004115,0.172839506172839,
0.174897119341564,0.176954732510288,0.179012345679012,0.181069958847737,
0.183127572016461,0.185185185185185,0.187242798353909,0.189300411522634,
0.191358024691358,0.193415637860082,0.195473251028807,0.197530864197531,
0.199588477366255,0.201646090534979,0.203703703703704,0.205761316872428,
0.207818930041152,0.209876543209877,0.211934156378601,0.213991769547325,
0.216049382716049,0.218106995884774,0.220164609053498,0.222222222222222,
0.224279835390947,0.226337448559671,0.228395061728395,0.230452674897119,
0.232510288065844,0.234567901234568,0.236625514403292,0.238683127572016,
0.240740740740741,0.242798353909465,0.244855967078189,0.246913580246914,
0.248971193415638,0.251028806584362,0.253086419753086,0.255144032921811,
0.257201646090535,0.259259259259259,0.261316872427984,0.263374485596708,
0.265432098765432,0.267489711934156,0.269547325102881,0.271604938271605,
0.273662551440329,0.275720164609054,0.277777777777778,0.279835390946502,
0.281893004115226,0.283950617283951,0.286008230452675,0.288065843621399,
0.290123456790123,0.292181069958848,0.294238683127572,0.296296296296296,
0.298353909465021,0.300411522633745,0.302469135802469,0.304526748971193,
0.306584362139918,0.308641975308642,0.310699588477366,0.312757201646091,
0.314814814814815,0.316872427983539,0.318930041152263,0.320987654320988,
0.323045267489712,0.325102880658436,0.327160493827161,0.329218106995885,
0.331275720164609,0.333333333333333,0.335390946502058,0.337448559670782,
0.339506172839506,0.34156378600823,0.343621399176955,0.345679012345679,
0.347736625514403,0.349794238683128,0.351851851851852,0.353909465020576,
0.3559670781893,0.358024691358025,0.360082304526749,0.362139917695473,0.364197530864198,
0.366255144032922,0.368312757201646,0.37037037037037,0.372427983539095,
0.374485596707819,0.376543209876543,0.378600823045267,0.380658436213992,
0.382716049382716,0.38477366255144,0.386831275720165,0.388888888888889,
0.390946502057613,0.393004115226337,0.395061728395062,0.397119341563786,
0.39917695473251,0.401234567901235,0.403292181069959,0.405349794238683,
0.407407407407407,0.409465020576132,0.411522633744856,0.41358024691358,
0.415637860082305,0.417695473251029,0.419753086419753,0.421810699588477,
0.423868312757202,0.425925925925926,0.42798353909465,0.430041152263374,
0.432098765432099,0.434156378600823,0.436213991769547,0.438271604938272,
0.440329218106996,0.44238683127572,0.444444444444444,0.446502057613169,
0.448559670781893,0.450617283950617,0.452674897119342,0.454732510288066,
0.45679012345679,0.458847736625514,0.460905349794239,0.462962962962963,
0.465020576131687,0.467078189300412,0.469135802469136,0.47119341563786,
0.473251028806584,0.475308641975309,0.477366255144033,0.479423868312757,
0.481481481481481,0.483539094650206,0.48559670781893,0.487654320987654,
0.489711934156379,0.491769547325103,0.493827160493827,0.495884773662551,
0.497942386831276,0.5,0.502057613168724,0.504115226337449,0.506172839506173,
0.508230452674897,0.510288065843621,0.512345679012346,0.51440329218107,
0.516460905349794,0.518518518518518,0.520576131687243,0.522633744855967,
0.524691358024691,0.526748971193416,0.52880658436214,0.530864197530864,
0.532921810699588,0.534979423868313,0.537037037037037,0.539094650205761,
0.541152263374486,0.54320987654321,0.545267489711934,0.547325102880658,
0.549382716049383,0.551440329218107,0.553497942386831,0.555555555555556,
0.55761316872428,0.559670781893004,0.561728395061728,0.563786008230453,
0.565843621399177,0.567901234567901,0.569958847736626,0.57201646090535,
0.574074074074074,0.576131687242798,0.578189300411523,0.580246913580247,
0.582304526748971,0.584362139917695,0.58641975308642,0.588477366255144,
0.590534979423868,0.592592592592593,0.594650205761317,0.596707818930041,
0.598765432098765,0.60082304526749,0.602880658436214,0.604938271604938,
0.606995884773663,0.609053497942387,0.611111111111111,0.613168724279835,
0.61522633744856,0.617283950617284,0.619341563786008,0.621399176954732,
0.623456790123457,0.625514403292181,0.627572016460905,0.62962962962963,
0.631687242798354,0.633744855967078,0.635802469135803,0.637860082304527,
0.639917695473251,0.641975308641975,0.6440329218107,0.646090534979424,0.648148148148148,
0.650205761316872,0.652263374485597,0.654320987654321,0.656378600823045,
0.65843621399177,0.660493827160494,0.662551440329218,0.664609053497942,
0.666666666666667,0.668724279835391,0.670781893004115,0.672839506172839,
0.674897119341564,0.676954732510288,0.679012345679012,0.681069958847737,
0.683127572016461,0.685185185185185,0.687242798353909,0.689300411522634,
0.691358024691358,0.693415637860082,0.695473251028807,0.697530864197531,
0.699588477366255,0.701646090534979,0.703703703703704,0.705761316872428,
0.707818930041152,0.709876543209877,0.711934156378601,0.713991769547325,
0.716049382716049,0.718106995884774,0.720164609053498,0.722222222222222,
0.724279835390947,0.726337448559671,0.728395061728395,0.730452674897119,
0.732510288065844,0.734567901234568,0.736625514403292,0.738683127572016,
0.740740740740741,0.742798353909465,0.744855967078189,0.746913580246914,
0.748971193415638,0.751028806584362,0.753086419753086,0.755144032921811,
0.757201646090535,0.759259259259259,0.761316872427984,0.763374485596708,
0.765432098765432,0.767489711934156,0.769547325102881,0.771604938271605,
0.773662551440329,0.775720164609053,0.777777777777778,0.779835390946502,
0.781893004115226,0.783950617283951,0.786008230452675,0.788065843621399,
0.790123456790123,0.792181069958848,0.794238683127572,0.796296296296296,
0.798353909465021,0.800411522633745,0.802469135802469,0.804526748971193,
0.806584362139918,0.808641975308642,0.810699588477366,0.812757201646091,
0.814814814814815,0.816872427983539,0.818930041152263,0.820987654320988,
0.823045267489712,0.825102880658436,0.827160493827161,0.829218106995885,
0.831275720164609,0.833333333333333,0.835390946502058,0.837448559670782,
0.839506172839506,0.84156378600823,0.843621399176955,0.845679012345679,
0.847736625514403,0.849794238683128,0.851851851851852,0.853909465020576,
0.8559670781893,0.858024691358025,0.860082304526749,0.862139917695473,0.864197530864197,
0.866255144032922,0.868312757201646,0.87037037037037,0.872427983539095,
0.874485596707819,0.876543209876543,0.878600823045268,0.880658436213992,
0.882716049382716,0.88477366255144,0.886831275720165,0.888888888888889,
0.890946502057613,0.893004115226337,0.895061728395062,0.897119341563786,
0.89917695473251,0.901234567901235,0.903292181069959,0.905349794238683,
0.907407407407407,0.909465020576132,0.911522633744856,0.91358024691358,
0.915637860082305,0.917695473251029,0.919753086419753,0.921810699588477,
0.923868312757202,0.925925925925926,0.92798353909465,0.930041152263374,
0.932098765432099,0.934156378600823,0.936213991769547,0.938271604938272,
0.940329218106996,0.94238683127572,0.944444444444444,0.946502057613169,
0.948559670781893,0.950617283950617,0.952674897119342,0.954732510288066,
0.95679012345679,0.958847736625514,0.960905349794239,0.962962962962963,
0.965020576131687,0.967078189300412,0.969135802469136,0.97119341563786,
0.973251028806584,0.975308641975309,0.977366255144033,0.979423868312757,
0.981481481481482,0.983539094650206,0.98559670781893,0.987654320987654,
0.989711934156379,0.991769547325103,0.993827160493827,0.995884773662551,
0.997942386831276,1.),.UNSPECIFIED.)
GEOMETRIC_REPRESENTATION_ITEM()
RATIONAL_B_SPLINE_SURFACE(((1.,0.866025403784439,1.,0.866025403784439,1.,
0.866025403784439,1.,0.866025403784439,1.,0.866025403784439,1.,0.866025403784439,
1.,0.866025403784439,1.,0.866025403784439,1.,0.866025403784439,1.,0.866025403784439,
1.,0.866025403784439,1.,0.866025403784439,1.,0.866025403784439,1.,0.866025403784439,
1.,0.866025403784439,1.,0.866025403784439,1.,0.866025403784439,1.,0.866025403784439,
1.,0.866025403784439,1.,0.866025403784439,1.,0.866025403784439,1.,0.866025403784439,
1.,0.866025403784439,1.,0.866025403784439,1.,0.866025403784439,1.,0.866025403784439,
1.,0.866025403784439,1.,0.866025403784439,1.,0.866025403784439,1.,0.866025403784439,
1.,0.866025403784439,1.,0.866025403784439,1.,0.866025403784439,1.,0.866025403784439,
1.,0.866025403784439,1.,0.866025403784439,1.,0.866025403784439,1.,0.866025403784439,
1.,0.866025403784439,1.,0.866025403784439,1.,0.866025403784439,1.,0.866025403784439,
1.,0.866025403784439,1.,0.866025403784439,1.,0.866025403784439,1.,0.866025403784439,
1.,0.866025403784439,1.,0.866025403784439,1.,0.866025403784439,1.,0.866025403784439,
1.,0.866025403784439,1.,0.866025403784439,1.,0.866025403784439,1.,0.866025403784439,
1.,0.866025403784439,1.,0.866025403784439,1.,0.866025403784439,1.,0.866025403784439,
1.,0.866025403784439,1.,0.866025403784439,1.,0.866025403784439,1.,0.866025403784439,
1.,0.866025403784439,1.,0.866025403784439,1.,0.866025403784439,1.,0.866025403784439,
1.,0.866025403784439,1.,0.866025403784439,1.,0.866025403784439,1.,0.866025403784439,
1.,0.866025403784439,1.,0.866025403784439,1.,0.866025403784439,1.,0.866025403784439,
1.,0.866025403784439,1.,0.866025403784439,1.,0.866025403784439,1.,0.866025403784439,
1.,0.866025403784439,1.,0.866025403784439,1.,0.866025403784439,1.,0.866025403784439,
1.,0.866025403784439,1.,0.866025403784439,1.,0.866025403784439,1.,0.866025403784439,
1.,0.866025403784439,1.,0.866025403784439,1.,0.866025403784439,1.,0.866025403784439,
1.,0.866025403784439,1.,0.866025403784439,1.,0.866025403784439,1.,0.866025403784439,
1.,0.866025403784439,1.,0.866025403784439,1.,0.866025403784439,1.,0.866025403784439,
1.,0.866025403784439,1.,0.866025403784439,1.,0.866025403784439,1.,0.866025403784439,
1.,0.866025403784439,1.,0.866025403784439,1.,0.866025403784439,1.,0.866025403784439,
1.,0.866025403784439,1.,0.866025403784439,1.,0.866025403784439,1.,0.866025403784439,
1.,0.866025403784439,1.,0.866025403784439,1.,0.866025403784439,1.,0.866025403784439,
1.,0.866025403784439,1.,0.866025403784439,1.,0.866025403784439,1.,0.866025403784439,
1.,0.866025403784439,1.,0.866025403784439,1.,0.866025403784439,1.,0.866025403784439,
1.,0.866025403784439,1.,0.866025403784439,1.,0.866025403784439,1.,0.866025403784439,
1.,0.866025403784439,1.,0.866025403784439,1.,0.866025403784439,1.,0.866025403784439,
1.,0.866025403784439,1.,0.866025403784439,1.,0.866025403784439,1.,0.866025403784439,
1.,0.866025403784439,1.,0.866025403784439,1.,0.866025403784439,1.,0.866025403784439,
1.,0.866025403784439,1.,0.866025403784439,1.,0.866025403784439,1.,0.866025403784439,
1.,0.866025403784439,1.,0.866025403784439,1.,0.866025403784439,1.,0.866025403784439,
1.,0.866025403784439,1.,0.866025403784439,1.,0.866025403784439,1.,0.866025403784439,
1.,0.866025403784439,1.,0.866025403784439,1.,0.866025403784439,1.,0.866025403784439,
1.,0.866025403784439,1.,0.866025403784439,1.,0.866025403784439,1.,0.866025403784439,
1.,0.866025403784439,1.,0.866025403784439,1.,0.866025403784439,1.,0.866025403784439,
1.,0.866025403784439,1.,0.866025403784439,1.,0.866025403784439,1.,0.866025403784439,
1.,0.866025403784439,1.,0.866025403784439,1.,0.866025403784439,1.,0.866025403784439,
1.,0.866025403784439,1.,0.866025403784439,1.,0.866025403784439,1.,0.866025403784439,
1.,0.866025403784439,1.,0.866025403784439,1.,0.866025403784439,1.,0.866025403784439,
1.,0.866025403784439,1.,0.866025403784439,1.,0.866025403784439,1.,0.866025403784439,
1.,0.866025403784439,1.,0.866025403784439,1.,0.866025403784439,1.,0.866025403784439,
1.,0.866025403784439,1.,0.866025403784439,1.,0.866025403784439,1.,0.866025403784439,
1.,0.866025403784439,1.,0.866025403784439,1.,0.866025403784439,1.,0.866025403784439,
1.,0.866025403784439,1.,0.866025403784439,1.,0.866025403784439,1.,0.866025403784439,
1.,0.866025403784439,1.,0.866025403784439,1.,0.866025403784439,1.,0.866025403784439,
1.,0.866025403784439,1.,0.866025403784439,1.,0.866025403784439,1.,0.866025403784439,
1.,0.866025403784439,1.,0.866025403784439,1.,0.866025403784439,1.,0.866025403784439,
1.,0.866025403784439,1.,0.866025403784439,1.,0.866025403784439,1.,0.866025403784439,
1.,0.866025403784439,1.,0.866025403784439,1.,0.866025403784439,1.,0.866025403784439,
1.,0.866025403784439,1.,0.866025403784439,1.,0.866025403784439,1.,0.866025403784439,
1.,0.866025403784439,1.,0.866025403784439,1.,0.866025403784439,1.,0.866025403784439,
1.,0.866025403784439,1.,0.866025403784439,1.,0.866025403784439,1.,0.866025403784439,
1.,0.866025403784439,1.,0.866025403784439,1.,0.866025403784439,1.,0.866025403784439,
1.,0.866025403784439,1.,0.866025403784439,1.,0.866025403784439,1.,0.866025403784439,
1.,0.866025403784439,1.,0.866025403784439,1.,0.866025403784439,1.,0.866025403784439,
1.,0.866025403784439,1.,0.866025403784439,1.,0.866025403784439,1.,0.866025403784439,
1.,0.866025403784439,1.,0.866025403784439,1.,0.866025403784439,1.,0.866025403784439,
1.,0.866025403784439,1.,0.866025403784439,1.,0.866025403784439,1.,0.866025403784439,
1.,0.866025403784439,1.,0.866025403784439,1.,0.866025403784439,1.,0.866025403784439,
1.,0.866025403784439,1.,0.866025403784439,1.,0.866025403784439,1.,0.866025403784439,
1.,0.866025403784439,1.,0.866025403784439,1.,0.866025403784439,1.,0.866025403784439,
1.,0.866025403784439,1.,0.866025403784439,1.,0.866025403784439,1.,0.866025403784439,
1.,0.866025403784439,1.,0.866025403784439,1.,0.866025403784439,1.,0.866025403784439,
1.,0.866025403784439,1.,0.866025403784439,1.,0.866025403784439,1.,0.866025403784439,
1.,0.866025403784439,1.,0.866025403784439,1.,0.866025403784439,1.,0.866025403784439,
1.,0.866025403784439,1.,0.866025403784439,1.,0.866025403784439,1.,0.866025403784439,
1.,0.866025403784439,1.,0.866025403784439,1.,0.866025403784439,1.,0.866025403784439,
1.,0.866025403784439,1.,0.866025403784439,1.,0.866025403784439,1.,0.866025403784439,
1.,0.866025403784439,1.,0.866025403784439,1.,0.866025403784439,1.,0.866025403784439,
1.,0.866025403784439,1.,0.866025403784439,1.,0.866025403784439,1.,0.866025403784439,
1.,0.866025403784439,1.,0.866025403784439,1.,0.866025403784439,1.,0.866025403784439,
1.,0.866025403784439,1.,0.866025403784439,1.,0.866025403784439,1.,0.866025403784439,
1.,0.866025403784439,1.,0.866025403784439,1.,0.866025403784439,1.,0.866025403784439,
1.,0.866025403784439,1.,0.866025403784439,1.,0.866025403784439,1.,0.866025403784439,
1.,0.866025403784439,1.,0.866025403784439,1.,0.866025403784439,1.,0.866025403784439,
1.,0.866025403784439,1.,0.866025403784439,1.,0.866025403784439,1.,0.866025403784439,
1.,0.866025403784439,1.,0.866025403784439,1.,0.866025403784439,1.,0.866025403784439,
1.,0.866025403784439,1.,0.866025403784439,1.,0.866025403784439,1.,0.866025403784439,
1.,0.866025403784439,1.,0.866025403784439,1.,0.866025403784439,1.,0.866025403784439,
1.,0.866025403784439,1.,0.866025403784439,1.,0.866025403784439,1.,0.866025403784439,
1.,0.866025403784439,1.,0.866025403784439,1.,0.866025403784439,1.,0.866025403784439,
1.,0.866025403784439,1.,0.866025403784439,1.,0.866025403784439,1.,0.866025403784439,
1.,0.866025403784439,1.,0.866025403784439,1.,0.866025403784439,1.,0.866025403784439,
1.,0.866025403784439,1.,0.866025403784439,1.,0.866025403784439,1.,0.866025403784439,
1.,0.866025403784439,1.,0.866025403784439,1.,0.866025403784439,1.,0.866025403784439,
1.,0.866025403784439,1.,0.866025403784439,1.,0.866025403784439,1.,0.866025403784439,
1.,0.866025403784439,1.,0.866025403784439,1.,0.866025403784439,1.,0.866025403784439,
1.,0.866025403784439,1.,0.866025403784439,1.,0.866025403784439,1.,0.866025403784439,
1.,0.866025403784439,1.,0.866025403784439,1.,0.866025403784439,1.,0.866025403784439,
1.,0.866025403784439,1.,0.866025403784439,1.,0.866025403784439,1.,0.866025403784439,
1.,0.866025403784439,1.,0.866025403784439,1.,0.866025403784439,1.,0.866025403784439,
1.,0.866025403784439,1.,0.866025403784439,1.,0.866025403784439,1.,0.866025403784439,
1.,0.866025403784439,1.,0.866025403784439,1.,0.866025403784439,1.,0.866025403784439,
1.,0.866025403784439,1.,0.866025403784439,1.,0.866025403784439,1.,0.866025403784439,
1.,0.866025403784439,1.,0.866025403784439,1.,0.866025403784439,1.,0.866025403784439,
1.,0.866025403784439,1.,0.866025403784439,1.,0.866025403784439,1.,0.866025403784439,
1.,0.866025403784439,1.,0.866025403784439,1.,0.866025403784439,1.,0.866025403784439,
1.,0.866025403784439,1.,0.866025403784439,1.,0.866025403784439,1.,0.866025403784439,
1.,0.866025403784439,1.,0.866025403784439,1.,0.866025403784439,1.,0.866025403784439,
1.,0.866025403784439,1.,0.866025403784439,1.,0.866025403784439,1.,0.866025403784439,
1.,0.866025403784439,1.,0.866025403784439,1.,0.866025403784439,1.,0.866025403784439,
1.,0.866025403784439,1.,0.866025403784439,1.,0.866025403784439,1.,0.866025403784439,
1.,0.866025403784439,1.,0.866025403784439,1.,0.866025403784439,1.,0.866025403784439,
1.,0.866025403784439,1.,0.866025403784439,1.,0.866025403784439,1.,0.866025403784439,
1.,0.866025403784439,1.,0.866025403784439,1.,0.866025403784439,1.,0.866025403784439,
1.,0.866025403784439,1.,0.866025403784439,1.,0.866025403784439,1.,0.866025403784439,
1.,0.866025403784439,1.,0.866025403784439,1.,0.866025403784439,1.,0.866025403784439,
1.,0.866025403784439,1.,0.866025403784439,1.,0.866025403784439,1.,0.866025403784439,
1.,0.866025403784439,1.,0.866025403784439,1.,0.866025403784439,1.,0.866025403784439,
1.,0.866025403784439,1.,0.866025403784439,1.,0.866025403784439,1.,0.866025403784439,
1.,0.866025403784439,1.,0.866025403784439,1.,0.866025403784439,1.,0.866025403784439,
1.,0.866025403784439,1.,0.866025403784439,1.,0.866025403784439,1.,0.866025403784439,
1.,0.866025403784439,1.,0.866025403784439,1.,0.866025403784439,1.,0.866025403784439,
1.,0.866025403784439,1.,0.866025403784439,1.,0.866025403784439,1.,0.866025403784439,
1.,0.866025403784439,1.,0.866025403784439,1.,0.866025403784439,1.,0.866025403784439,
1.,0.866025403784439,1.,0.866025403784439,1.,0.866025403784439,1.,0.866025403784439,
1.),(0.641165742156689,0.555265820743996,0.641165742156689,0.555265820743996,
0.641165742156689,0.555265820743996,0.641165742156689,0.555265820743996,
0.641165742156689,0.555265820743996,0.641165742156689,0.555265820743996,
0.641165742156689,0.555265820743996,0.641165742156689,0.555265820743996,
0.641165742156689,0.555265820743996,0.641165742156689,0.555265820743996,
0.641165742156689,0.555265820743996,0.641165742156689,0.555265820743996,
0.641165742156689,0.555265820743996,0.641165742156689,0.555265820743996,
0.641165742156689,0.555265820743996,0.641165742156689,0.555265820743996,
0.641165742156689,0.555265820743996,0.641165742156689,0.555265820743996,
0.641165742156689,0.555265820743996,0.641165742156689,0.555265820743996,
0.641165742156689,0.555265820743996,0.641165742156689,0.555265820743996,
0.641165742156689,0.555265820743996,0.641165742156689,0.555265820743996,
0.641165742156689,0.555265820743996,0.641165742156689,0.555265820743996,
0.641165742156689,0.555265820743996,0.641165742156689,0.555265820743996,
0.641165742156689,0.555265820743996,0.641165742156689,0.555265820743996,
0.641165742156689,0.555265820743996,0.641165742156689,0.555265820743996,
0.641165742156689,0.555265820743996,0.641165742156689,0.555265820743996,
0.641165742156689,0.555265820743996,0.641165742156689,0.555265820743996,
0.641165742156689,0.555265820743996,0.641165742156689,0.555265820743996,
0.641165742156689,0.555265820743996,0.641165742156689,0.555265820743996,
0.641165742156689,0.555265820743996,0.641165742156689,0.555265820743996,
0.641165742156689,0.555265820743996,0.641165742156689,0.555265820743996,
0.641165742156689,0.555265820743996,0.641165742156689,0.555265820743996,
0.641165742156689,0.555265820743996,0.641165742156689,0.555265820743996,
0.641165742156689,0.555265820743996,0.641165742156689,0.555265820743996,
0.641165742156689,0.555265820743996,0.641165742156689,0.555265820743996,
0.641165742156689,0.555265820743996,0.641165742156689,0.555265820743996,
0.641165742156689,0.555265820743996,0.641165742156689,0.555265820743996,
0.641165742156689,0.555265820743996,0.641165742156689,0.555265820743996,
0.641165742156689,0.555265820743996,0.641165742156689,0.555265820743996,
0.641165742156689,0.555265820743996,0.641165742156689,0.555265820743996,
0.641165742156689,0.555265820743996,0.641165742156689,0.555265820743996,
0.641165742156689,0.555265820743996,0.641165742156689,0.555265820743996,
0.641165742156689,0.555265820743996,0.641165742156689,0.555265820743996,
0.641165742156689,0.555265820743996,0.641165742156689,0.555265820743996,
0.641165742156689,0.555265820743996,0.641165742156689,0.555265820743996,
0.641165742156689,0.555265820743996,0.641165742156689,0.555265820743996,
0.641165742156689,0.555265820743996,0.641165742156689,0.555265820743996,
0.641165742156689,0.555265820743996,0.641165742156689,0.555265820743996,
0.641165742156689,0.555265820743996,0.641165742156689,0.555265820743996,
0.641165742156689,0.555265820743996,0.641165742156689,0.555265820743996,
0.641165742156689,0.555265820743996,0.641165742156689,0.555265820743996,
0.641165742156689,0.555265820743996,0.641165742156689,0.555265820743996,
0.641165742156689,0.555265820743996,0.641165742156689,0.555265820743996,
0.641165742156689,0.555265820743996,0.641165742156689,0.555265820743996,
0.641165742156689,0.555265820743996,0.641165742156689,0.555265820743996,
0.641165742156689,0.555265820743996,0.641165742156689,0.555265820743996,
0.641165742156689,0.555265820743996,0.641165742156689,0.555265820743996,
0.641165742156689,0.555265820743996,0.641165742156689,0.555265820743996,
0.641165742156689,0.555265820743996,0.641165742156689,0.555265820743996,
0.641165742156689,0.555265820743996,0.641165742156689,0.555265820743996,
0.641165742156689,0.555265820743996,0.641165742156689,0.555265820743996,
0.641165742156689,0.555265820743996,0.641165742156689,0.555265820743996,
0.641165742156689,0.555265820743996,0.641165742156689,0.555265820743996,
0.641165742156689,0.555265820743996,0.641165742156689,0.555265820743996,
0.641165742156689,0.555265820743996,0.641165742156689,0.555265820743996,
0.641165742156689,0.555265820743996,0.641165742156689,0.555265820743996,
0.641165742156689,0.555265820743996,0.641165742156689,0.555265820743996,
0.641165742156689,0.555265820743996,0.641165742156689,0.555265820743996,
0.641165742156689,0.555265820743996,0.641165742156689,0.555265820743996,
0.641165742156689,0.555265820743996,0.641165742156689,0.555265820743996,
0.641165742156689,0.555265820743996,0.641165742156689,0.555265820743996,
0.641165742156689,0.555265820743996,0.641165742156689,0.555265820743996,
0.641165742156689,0.555265820743996,0.641165742156689,0.555265820743996,
0.641165742156689,0.555265820743996,0.641165742156689,0.555265820743996,
0.641165742156689,0.555265820743996,0.641165742156689,0.555265820743996,
0.641165742156689,0.555265820743996,0.641165742156689,0.555265820743996,
0.641165742156689,0.555265820743996,0.641165742156689,0.555265820743996,
0.641165742156689,0.555265820743996,0.641165742156689,0.555265820743996,
0.641165742156689,0.555265820743996,0.641165742156689,0.555265820743996,
0.641165742156689,0.555265820743996,0.641165742156689,0.555265820743996,
0.641165742156689,0.555265820743996,0.641165742156689,0.555265820743996,
0.641165742156689,0.555265820743996,0.641165742156689,0.555265820743996,
0.641165742156689,0.555265820743996,0.641165742156689,0.555265820743996,
0.641165742156689,0.555265820743996,0.641165742156689,0.555265820743996,
0.641165742156689,0.555265820743996,0.641165742156689,0.555265820743996,
0.641165742156689,0.555265820743996,0.641165742156689,0.555265820743996,
0.641165742156689,0.555265820743996,0.641165742156689,0.555265820743996,
0.641165742156689,0.555265820743996,0.641165742156689,0.555265820743996,
0.641165742156689,0.555265820743996,0.641165742156689,0.555265820743996,
0.641165742156689,0.555265820743996,0.641165742156689,0.555265820743996,
0.641165742156689,0.555265820743996,0.641165742156689,0.555265820743996,
0.641165742156689,0.555265820743996,0.641165742156689,0.555265820743996,
0.641165742156689,0.555265820743996,0.641165742156689,0.555265820743996,
0.641165742156689,0.555265820743996,0.641165742156689,0.555265820743996,
0.641165742156689,0.555265820743996,0.641165742156689,0.555265820743996,
0.641165742156689,0.555265820743996,0.641165742156689,0.555265820743996,
0.641165742156689,0.555265820743996,0.641165742156689,0.555265820743996,
0.641165742156689,0.555265820743996,0.641165742156689,0.555265820743996,
0.641165742156689,0.555265820743996,0.641165742156689,0.555265820743996,
0.641165742156689,0.555265820743996,0.641165742156689,0.555265820743996,
0.641165742156689,0.555265820743996,0.641165742156689,0.555265820743996,
0.641165742156689,0.555265820743996,0.641165742156689,0.555265820743996,
0.641165742156689,0.555265820743996,0.641165742156689,0.555265820743996,
0.641165742156689,0.555265820743996,0.641165742156689,0.555265820743996,
0.641165742156689,0.555265820743996,0.641165742156689,0.555265820743996,
0.641165742156689,0.555265820743996,0.641165742156689,0.555265820743996,
0.641165742156689,0.555265820743996,0.641165742156689,0.555265820743996,
0.641165742156689,0.555265820743996,0.641165742156689,0.555265820743996,
0.641165742156689,0.555265820743996,0.641165742156689,0.555265820743996,
0.641165742156689,0.555265820743996,0.641165742156689,0.555265820743996,
0.641165742156689,0.555265820743996,0.641165742156689,0.555265820743996,
0.641165742156689,0.555265820743996,0.641165742156689,0.555265820743996,
0.641165742156689,0.555265820743996,0.641165742156689,0.555265820743996,
0.641165742156689,0.555265820743996,0.641165742156689,0.555265820743996,
0.641165742156689,0.555265820743996,0.641165742156689,0.555265820743996,
0.641165742156689,0.555265820743996,0.641165742156689,0.555265820743996,
0.641165742156689,0.555265820743996,0.641165742156689,0.555265820743996,
0.641165742156689,0.555265820743996,0.641165742156689,0.555265820743996,
0.641165742156689,0.555265820743996,0.641165742156689,0.555265820743996,
0.641165742156689,0.555265820743996,0.641165742156689,0.555265820743996,
0.641165742156689,0.555265820743996,0.641165742156689,0.555265820743996,
0.641165742156689,0.555265820743996,0.641165742156689,0.555265820743996,
0.641165742156689,0.555265820743996,0.641165742156689,0.555265820743996,
0.641165742156689,0.555265820743996,0.641165742156689,0.555265820743996,
0.641165742156689,0.555265820743996,0.641165742156689,0.555265820743996,
0.641165742156689,0.555265820743996,0.641165742156689,0.555265820743996,
0.641165742156689,0.555265820743996,0.641165742156689,0.555265820743996,
0.641165742156689,0.555265820743996,0.641165742156689,0.555265820743996,
0.641165742156689,0.555265820743996,0.641165742156689,0.555265820743996,
0.641165742156689,0.555265820743996,0.641165742156689,0.555265820743996,
0.641165742156689,0.555265820743996,0.641165742156689,0.555265820743996,
0.641165742156689,0.555265820743996,0.641165742156689,0.555265820743996,
0.641165742156689,0.555265820743996,0.641165742156689,0.555265820743996,
0.641165742156689,0.555265820743996,0.641165742156689,0.555265820743996,
0.641165742156689,0.555265820743996,0.641165742156689,0.555265820743996,
0.641165742156689,0.555265820743996,0.641165742156689,0.555265820743996,
0.641165742156689,0.555265820743996,0.641165742156689,0.555265820743996,
0.641165742156689,0.555265820743996,0.641165742156689,0.555265820743996,
0.641165742156689,0.555265820743996,0.641165742156689,0.555265820743996,
0.641165742156689,0.555265820743996,0.641165742156689,0.555265820743996,
0.641165742156689,0.555265820743996,0.641165742156689,0.555265820743996,
0.641165742156689,0.555265820743996,0.641165742156689,0.555265820743996,
0.641165742156689,0.555265820743996,0.641165742156689,0.555265820743996,
0.641165742156689,0.555265820743996,0.641165742156689,0.555265820743996,
0.641165742156689,0.555265820743996,0.641165742156689,0.555265820743996,
0.641165742156689,0.555265820743996,0.641165742156689,0.555265820743996,
0.641165742156689,0.555265820743996,0.641165742156689,0.555265820743996,
0.641165742156689,0.555265820743996,0.641165742156689,0.555265820743996,
0.641165742156689,0.555265820743996,0.641165742156689,0.555265820743996,
0.641165742156689,0.555265820743996,0.641165742156689,0.555265820743996,
0.641165742156689,0.555265820743996,0.641165742156689,0.555265820743996,
0.641165742156689,0.555265820743996,0.641165742156689,0.555265820743996,
0.641165742156689,0.555265820743996,0.641165742156689,0.555265820743996,
0.641165742156689,0.555265820743996,0.641165742156689,0.555265820743996,
0.641165742156689,0.555265820743996,0.641165742156689,0.555265820743996,
0.641165742156689,0.555265820743996,0.641165742156689,0.555265820743996,
0.641165742156689,0.555265820743996,0.641165742156689,0.555265820743996,
0.641165742156689,0.555265820743996,0.641165742156689,0.555265820743996,
0.641165742156689,0.555265820743996,0.641165742156689,0.555265820743996,
0.641165742156689,0.555265820743996,0.641165742156689,0.555265820743996,
0.641165742156689,0.555265820743996,0.641165742156689,0.555265820743996,
0.641165742156689,0.555265820743996,0.641165742156689,0.555265820743996,
0.641165742156689,0.555265820743996,0.641165742156689,0.555265820743996,
0.641165742156689,0.555265820743996,0.641165742156689,0.555265820743996,
0.641165742156689,0.555265820743996,0.641165742156689,0.555265820743996,
0.641165742156689,0.555265820743996,0.641165742156689,0.555265820743996,
0.641165742156689,0.555265820743996,0.641165742156689,0.555265820743996,
0.641165742156689,0.555265820743996,0.641165742156689,0.555265820743996,
0.641165742156689,0.555265820743996,0.641165742156689,0.555265820743996,
0.641165742156689,0.555265820743996,0.641165742156689,0.555265820743996,
0.641165742156689,0.555265820743996,0.641165742156689,0.555265820743996,
0.641165742156689,0.555265820743996,0.641165742156689,0.555265820743996,
0.641165742156689,0.555265820743996,0.641165742156689,0.555265820743996,
0.641165742156689,0.555265820743996,0.641165742156689,0.555265820743996,
0.641165742156689,0.555265820743996,0.641165742156689,0.555265820743996,
0.641165742156689,0.555265820743996,0.641165742156689,0.555265820743996,
0.641165742156689,0.555265820743996,0.641165742156689,0.555265820743996,
0.641165742156689,0.555265820743996,0.641165742156689,0.555265820743996,
0.641165742156689,0.555265820743996,0.641165742156689,0.555265820743996,
0.641165742156689,0.555265820743996,0.641165742156689,0.555265820743996,
0.641165742156689,0.555265820743996,0.641165742156689,0.555265820743996,
0.641165742156689,0.555265820743996,0.641165742156689,0.555265820743996,
0.641165742156689,0.555265820743996,0.641165742156689,0.555265820743996,
0.641165742156689,0.555265820743996,0.641165742156689,0.555265820743996,
0.641165742156689,0.555265820743996,0.641165742156689,0.555265820743996,
0.641165742156689,0.555265820743996,0.641165742156689,0.555265820743996,
0.641165742156689,0.555265820743996,0.641165742156689,0.555265820743996,
0.641165742156689,0.555265820743996,0.641165742156689,0.555265820743996,
0.641165742156689,0.555265820743996,0.641165742156689,0.555265820743996,
0.641165742156689,0.555265820743996,0.641165742156689,0.555265820743996,
0.641165742156689,0.555265820743996,0.641165742156689,0.555265820743996,
0.641165742156689,0.555265820743996,0.641165742156689,0.555265820743996,
0.641165742156689,0.555265820743996,0.641165742156689,0.555265820743996,
0.641165742156689,0.555265820743996,0.641165742156689,0.555265820743996,
0.641165742156689,0.555265820743996,0.641165742156689,0.555265820743996,
0.641165742156689,0.555265820743996,0.641165742156689,0.555265820743996,
0.641165742156689,0.555265820743996,0.641165742156689,0.555265820743996,
0.641165742156689,0.555265820743996,0.641165742156689,0.555265820743996,
0.641165742156689,0.555265820743996,0.641165742156689,0.555265820743996,
0.641165742156689,0.555265820743996,0.641165742156689,0.555265820743996,
0.641165742156689,0.555265820743996,0.641165742156689,0.555265820743996,
0.641165742156689,0.555265820743996,0.641165742156689,0.555265820743996,
0.641165742156689,0.555265820743996,0.641165742156689,0.555265820743996,
0.641165742156689,0.555265820743996,0.641165742156689,0.555265820743996,
0.641165742156689,0.555265820743996,0.641165742156689,0.555265820743996,
0.641165742156689,0.555265820743996,0.641165742156689,0.555265820743996,
0.641165742156689,0.555265820743996,0.641165742156689,0.555265820743996,
0.641165742156689,0.555265820743996,0.641165742156689,0.555265820743996,
0.641165742156689,0.555265820743996,0.641165742156689,0.555265820743996,
0.641165742156689,0.555265820743996,0.641165742156689,0.555265820743996,
0.641165742156689,0.555265820743996,0.641165742156689,0.555265820743996,
0.641165742156689,0.555265820743996,0.641165742156689,0.555265820743996,
0.641165742156689,0.555265820743996,0.641165742156689,0.555265820743996,
0.641165742156689,0.555265820743996,0.641165742156689,0.555265820743996,
0.641165742156689,0.555265820743996,0.641165742156689,0.555265820743996,
0.641165742156689,0.555265820743996,0.641165742156689,0.555265820743996,
0.641165742156689,0.555265820743996,0.641165742156689,0.555265820743996,
0.641165742156689,0.555265820743996,0.641165742156689,0.555265820743996,
0.641165742156689,0.555265820743996,0.641165742156689,0.555265820743996,
0.641165742156689,0.555265820743996,0.641165742156689,0.555265820743996,
0.641165742156689,0.555265820743996,0.641165742156689,0.555265820743996,
0.641165742156689,0.555265820743996,0.641165742156689,0.555265820743996,
0.641165742156689,0.555265820743996,0.641165742156689,0.555265820743996,
0.641165742156689,0.555265820743996,0.641165742156689,0.555265820743996,
0.641165742156689,0.555265820743996,0.641165742156689,0.555265820743996,
0.641165742156689,0.555265820743996,0.641165742156689,0.555265820743996,
0.641165742156689,0.555265820743996,0.641165742156689,0.555265820743996,
0.641165742156689,0.555265820743996,0.641165742156689,0.555265820743996,
0.641165742156689,0.555265820743996,0.641165742156689,0.555265820743996,
0.641165742156689,0.555265820743996,0.641165742156689,0.555265820743996,
0.641165742156689,0.555265820743996,0.641165742156689,0.555265820743996,
0.641165742156689,0.555265820743996,0.641165742156689,0.555265820743996,
0.641165742156689,0.555265820743996,0.641165742156689,0.555265820743996,
0.641165742156689,0.555265820743996,0.641165742156689,0.555265820743996,
0.641165742156689,0.555265820743996,0.641165742156689,0.555265820743996,
0.641165742156689,0.555265820743996,0.641165742156689,0.555265820743996,
0.641165742156689,0.555265820743996,0.641165742156689,0.555265820743996,
0.641165742156689,0.555265820743996,0.641165742156689,0.555265820743996,
0.641165742156689,0.555265820743996,0.641165742156689,0.555265820743996,
0.641165742156689,0.555265820743996,0.641165742156689,0.555265820743996,
0.641165742156689,0.555265820743996,0.641165742156689,0.555265820743996,
0.641165742156689,0.555265820743996,0.641165742156689,0.555265820743996,
0.641165742156689,0.555265820743996,0.641165742156689,0.555265820743996,
0.641165742156689,0.555265820743996,0.641165742156689,0.555265820743996,
0.641165742156689,0.555265820743996,0.641165742156689,0.555265820743996,
0.641165742156689,0.555265820743996,0.641165742156689,0.555265820743996,
0.641165742156689,0.555265820743996,0.641165742156689,0.555265820743996,
0.641165742156689,0.555265820743996,0.641165742156689,0.555265820743996,
0.641165742156689,0.555265820743996,0.641165742156689,0.555265820743996,
0.641165742156689,0.555265820743996,0.641165742156689,0.555265820743996,
0.641165742156689,0.555265820743996,0.641165742156689,0.555265820743996,
0.641165742156689,0.555265820743996,0.641165742156689,0.555265820743996,
0.641165742156689),(0.641165742156689,0.555265820743996,0.641165742156689,
0.555265820743996,0.641165742156689,0.555265820743996,0.641165742156689,
0.555265820743996,0.641165742156689,0.555265820743996,0.641165742156689,
0.555265820743996,0.641165742156689,0.555265820743996,0.641165742156689,
0.555265820743996,0.641165742156689,0.555265820743996,0.641165742156689,
0.555265820743996,0.641165742156689,0.555265820743996,0.641165742156689,
0.555265820743996,0.641165742156689,0.555265820743996,0.641165742156689,
0.555265820743996,0.641165742156689,0.555265820743996,0.641165742156689,
0.555265820743996,0.641165742156689,0.555265820743996,0.641165742156689,
0.555265820743996,0.641165742156689,0.555265820743996,0.641165742156689,
0.555265820743996,0.641165742156689,0.555265820743996,0.641165742156689,
0.555265820743996,0.641165742156689,0.555265820743996,0.641165742156689,
0.555265820743996,0.641165742156689,0.555265820743996,0.641165742156689,
0.555265820743996,0.641165742156689,0.555265820743996,0.641165742156689,
0.555265820743996,0.641165742156689,0.555265820743996,0.641165742156689,
0.555265820743996,0.641165742156689,0.555265820743996,0.641165742156689,
0.555265820743996,0.641165742156689,0.555265820743996,0.641165742156689,
0.555265820743996,0.641165742156689,0.555265820743996,0.641165742156689,
0.555265820743996,0.641165742156689,0.555265820743996,0.641165742156689,
0.555265820743996,0.641165742156689,0.555265820743996,0.641165742156689,
0.555265820743996,0.641165742156689,0.555265820743996,0.641165742156689,
0.555265820743996,0.641165742156689,0.555265820743996,0.641165742156689,
0.555265820743996,0.641165742156689,0.555265820743996,0.641165742156689,
0.555265820743996,0.641165742156689,0.555265820743996,0.641165742156689,
0.555265820743996,0.641165742156689,0.555265820743996,0.641165742156689,
0.555265820743996,0.641165742156689,0.555265820743996,0.641165742156689,
0.555265820743996,0.641165742156689,0.555265820743996,0.641165742156689,
0.555265820743996,0.641165742156689,0.555265820743996,0.641165742156689,
0.555265820743996,0.641165742156689,0.555265820743996,0.641165742156689,
0.555265820743996,0.641165742156689,0.555265820743996,0.641165742156689,
0.555265820743996,0.641165742156689,0.555265820743996,0.641165742156689,
0.555265820743996,0.641165742156689,0.555265820743996,0.641165742156689,
0.555265820743996,0.641165742156689,0.555265820743996,0.641165742156689,
0.555265820743996,0.641165742156689,0.555265820743996,0.641165742156689,
0.555265820743996,0.641165742156689,0.555265820743996,0.641165742156689,
0.555265820743996,0.641165742156689,0.555265820743996,0.641165742156689,
0.555265820743996,0.641165742156689,0.555265820743996,0.641165742156689,
0.555265820743996,0.641165742156689,0.555265820743996,0.641165742156689,
0.555265820743996,0.641165742156689,0.555265820743996,0.641165742156689,
0.555265820743996,0.641165742156689,0.555265820743996,0.641165742156689,
0.555265820743996,0.641165742156689,0.555265820743996,0.641165742156689,
0.555265820743996,0.641165742156689,0.555265820743996,0.641165742156689,
0.555265820743996,0.641165742156689,0.555265820743996,0.641165742156689,
0.555265820743996,0.641165742156689,0.555265820743996,0.641165742156689,
0.555265820743996,0.641165742156689,0.555265820743996,0.641165742156689,
0.555265820743996,0.641165742156689,0.555265820743996,0.641165742156689,
0.555265820743996,0.641165742156689,0.555265820743996,0.641165742156689,
0.555265820743996,0.641165742156689,0.555265820743996,0.641165742156689,
0.555265820743996,0.641165742156689,0.555265820743996,0.641165742156689,
0.555265820743996,0.641165742156689,0.555265820743996,0.641165742156689,
0.555265820743996,0.641165742156689,0.555265820743996,0.641165742156689,
0.555265820743996,0.641165742156689,0.555265820743996,0.641165742156689,
0.555265820743996,0.641165742156689,0.555265820743996,0.641165742156689,
0.555265820743996,0.641165742156689,0.555265820743996,0.641165742156689,
0.555265820743996,0.641165742156689,0.555265820743996,0.641165742156689,
0.555265820743996,0.641165742156689,0.555265820743996,0.641165742156689,
0.555265820743996,0.641165742156689,0.555265820743996,0.641165742156689,
0.555265820743996,0.641165742156689,0.555265820743996,0.641165742156689,
0.555265820743996,0.641165742156689,0.555265820743996,0.641165742156689,
0.555265820743996,0.641165742156689,0.555265820743996,0.641165742156689,
0.555265820743996,0.641165742156689,0.555265820743996,0.641165742156689,
0.555265820743996,0.641165742156689,0.555265820743996,0.641165742156689,
0.555265820743996,0.641165742156689,0.555265820743996,0.641165742156689,
0.555265820743996,0.641165742156689,0.555265820743996,0.641165742156689,
0.555265820743996,0.641165742156689,0.555265820743996,0.641165742156689,
0.555265820743996,0.641165742156689,0.555265820743996,0.641165742156689,
0.555265820743996,0.641165742156689,0.555265820743996,0.641165742156689,
0.555265820743996,0.641165742156689,0.555265820743996,0.641165742156689,
0.555265820743996,0.641165742156689,0.555265820743996,0.641165742156689,
0.555265820743996,0.641165742156689,0.555265820743996,0.641165742156689,
0.555265820743996,0.641165742156689,0.555265820743996,0.641165742156689,
0.555265820743996,0.641165742156689,0.555265820743996,0.641165742156689,
0.555265820743996,0.641165742156689,0.555265820743996,0.641165742156689,
0.555265820743996,0.641165742156689,0.555265820743996,0.641165742156689,
0.555265820743996,0.641165742156689,0.555265820743996,0.641165742156689,
0.555265820743996,0.641165742156689,0.555265820743996,0.641165742156689,
0.555265820743996,0.641165742156689,0.555265820743996,0.641165742156689,
0.555265820743996,0.641165742156689,0.555265820743996,0.641165742156689,
0.555265820743996,0.641165742156689,0.555265820743996,0.641165742156689,
0.555265820743996,0.641165742156689,0.555265820743996,0.641165742156689,
0.555265820743996,0.641165742156689,0.555265820743996,0.641165742156689,
0.555265820743996,0.641165742156689,0.555265820743996,0.641165742156689,
0.555265820743996,0.641165742156689,0.555265820743996,0.641165742156689,
0.555265820743996,0.641165742156689,0.555265820743996,0.641165742156689,
0.555265820743996,0.641165742156689,0.555265820743996,0.641165742156689,
0.555265820743996,0.641165742156689,0.555265820743996,0.641165742156689,
0.555265820743996,0.641165742156689,0.555265820743996,0.641165742156689,
0.555265820743996,0.641165742156689,0.555265820743996,0.641165742156689,
0.555265820743996,0.641165742156689,0.555265820743996,0.641165742156689,
0.555265820743996,0.641165742156689,0.555265820743996,0.641165742156689,
0.555265820743996,0.641165742156689,0.555265820743996,0.641165742156689,
0.555265820743996,0.641165742156689,0.555265820743996,0.641165742156689,
0.555265820743996,0.641165742156689,0.555265820743996,0.641165742156689,
0.555265820743996,0.641165742156689,0.555265820743996,0.641165742156689,
0.555265820743996,0.641165742156689,0.555265820743996,0.641165742156689,
0.555265820743996,0.641165742156689,0.555265820743996,0.641165742156689,
0.555265820743996,0.641165742156689,0.555265820743996,0.641165742156689,
0.555265820743996,0.641165742156689,0.555265820743996,0.641165742156689,
0.555265820743996,0.641165742156689,0.555265820743996,0.641165742156689,
0.555265820743996,0.641165742156689,0.555265820743996,0.641165742156689,
0.555265820743996,0.641165742156689,0.555265820743996,0.641165742156689,
0.555265820743996,0.641165742156689,0.555265820743996,0.641165742156689,
0.555265820743996,0.641165742156689,0.555265820743996,0.641165742156689,
0.555265820743996,0.641165742156689,0.555265820743996,0.641165742156689,
0.555265820743996,0.641165742156689,0.555265820743996,0.641165742156689,
0.555265820743996,0.641165742156689,0.555265820743996,0.641165742156689,
0.555265820743996,0.641165742156689,0.555265820743996,0.641165742156689,
0.555265820743996,0.641165742156689,0.555265820743996,0.641165742156689,
0.555265820743996,0.641165742156689,0.555265820743996,0.641165742156689,
0.555265820743996,0.641165742156689,0.555265820743996,0.641165742156689,
0.555265820743996,0.641165742156689,0.555265820743996,0.641165742156689,
0.555265820743996,0.641165742156689,0.555265820743996,0.641165742156689,
0.555265820743996,0.641165742156689,0.555265820743996,0.641165742156689,
0.555265820743996,0.641165742156689,0.555265820743996,0.641165742156689,
0.555265820743996,0.641165742156689,0.555265820743996,0.641165742156689,
0.555265820743996,0.641165742156689,0.555265820743996,0.641165742156689,
0.555265820743996,0.641165742156689,0.555265820743996,0.641165742156689,
0.555265820743996,0.641165742156689,0.555265820743996,0.641165742156689,
0.555265820743996,0.641165742156689,0.555265820743996,0.641165742156689,
0.555265820743996,0.641165742156689,0.555265820743996,0.641165742156689,
0.555265820743996,0.641165742156689,0.555265820743996,0.641165742156689,
0.555265820743996,0.641165742156689,0.555265820743996,0.641165742156689,
0.555265820743996,0.641165742156689,0.555265820743996,0.641165742156689,
0.555265820743996,0.641165742156689,0.555265820743996,0.641165742156689,
0.555265820743996,0.641165742156689,0.555265820743996,0.641165742156689,
0.555265820743996,0.641165742156689,0.555265820743996,0.641165742156689,
0.555265820743996,0.641165742156689,0.555265820743996,0.641165742156689,
0.555265820743996,0.641165742156689,0.555265820743996,0.641165742156689,
0.555265820743996,0.641165742156689,0.555265820743996,0.641165742156689,
0.555265820743996,0.641165742156689,0.555265820743996,0.641165742156689,
0.555265820743996,0.641165742156689,0.555265820743996,0.641165742156689,
0.555265820743996,0.641165742156689,0.555265820743996,0.641165742156689,
0.555265820743996,0.641165742156689,0.555265820743996,0.641165742156689,
0.555265820743996,0.641165742156689,0.555265820743996,0.641165742156689,
0.555265820743996,0.641165742156689,0.555265820743996,0.641165742156689,
0.555265820743996,0.641165742156689,0.555265820743996,0.641165742156689,
0.555265820743996,0.641165742156689,0.555265820743996,0.641165742156689,
0.555265820743996,0.641165742156689,0.555265820743996,0.641165742156689,
0.555265820743996,0.641165742156689,0.555265820743996,0.641165742156689,
0.555265820743996,0.641165742156689,0.555265820743996,0.641165742156689,
0.555265820743996,0.641165742156689,0.555265820743996,0.641165742156689,
0.555265820743996,0.641165742156689,0.555265820743996,0.641165742156689,
0.555265820743996,0.641165742156689,0.555265820743996,0.641165742156689,
0.555265820743996,0.641165742156689,0.555265820743996,0.641165742156689,
0.555265820743996,0.641165742156689,0.555265820743996,0.641165742156689,
0.555265820743996,0.641165742156689,0.555265820743996,0.641165742156689,
0.555265820743996,0.641165742156689,0.555265820743996,0.641165742156689,
0.555265820743996,0.641165742156689,0.555265820743996,0.641165742156689,
0.555265820743996,0.641165742156689,0.555265820743996,0.641165742156689,
0.555265820743996,0.641165742156689,0.555265820743996,0.641165742156689,
0.555265820743996,0.641165742156689,0.555265820743996,0.641165742156689,
0.555265820743996,0.641165742156689,0.555265820743996,0.641165742156689,
0.555265820743996,0.641165742156689,0.555265820743996,0.641165742156689,
0.555265820743996,0.641165742156689,0.555265820743996,0.641165742156689,
0.555265820743996,0.641165742156689,0.555265820743996,0.641165742156689,
0.555265820743996,0.641165742156689,0.555265820743996,0.641165742156689,
0.555265820743996,0.641165742156689,0.555265820743996,0.641165742156689,
0.555265820743996,0.641165742156689,0.555265820743996,0.641165742156689,
0.555265820743996,0.641165742156689,0.555265820743996,0.641165742156689,
0.555265820743996,0.641165742156689,0.555265820743996,0.641165742156689,
0.555265820743996,0.641165742156689,0.555265820743996,0.641165742156689,
0.555265820743996,0.641165742156689,0.555265820743996,0.641165742156689,
0.555265820743996,0.641165742156689,0.555265820743996,0.641165742156689,
0.555265820743996,0.641165742156689,0.555265820743996,0.641165742156689,
0.555265820743996,0.641165742156689,0.555265820743996,0.641165742156689,
0.555265820743996,0.641165742156689,0.555265820743996,0.641165742156689,
0.555265820743996,0.641165742156689,0.555265820743996,0.641165742156689,
0.555265820743996,0.641165742156689,0.555265820743996,0.641165742156689,
0.555265820743996,0.641165742156689,0.555265820743996,0.641165742156689,
0.555265820743996,0.641165742156689,0.555265820743996,0.641165742156689,
0.555265820743996,0.641165742156689,0.555265820743996,0.641165742156689,
0.555265820743996,0.641165742156689,0.555265820743996,0.641165742156689,
0.555265820743996,0.641165742156689,0.555265820743996,0.641165742156689,
0.555265820743996,0.641165742156689,0.555265820743996,0.641165742156689,
0.555265820743996,0.641165742156689,0.555265820743996,0.641165742156689,
0.555265820743996,0.641165742156689,0.555265820743996,0.641165742156689,
0.555265820743996,0.641165742156689,0.555265820743996,0.641165742156689,
0.555265820743996,0.641165742156689,0.555265820743996,0.641165742156689,
0.555265820743996,0.641165742156689,0.555265820743996,0.641165742156689,
0.555265820743996,0.641165742156689,0.555265820743996,0.641165742156689,
0.555265820743996,0.641165742156689,0.555265820743996,0.641165742156689,
0.555265820743996,0.641165742156689,0.555265820743996,0.641165742156689,
0.555265820743996,0.641165742156689,0.555265820743996,0.641165742156689,
0.555265820743996,0.641165742156689,0.555265820743996,0.641165742156689,
0.555265820743996,0.641165742156689,0.555265820743996,0.641165742156689,
0.555265820743996,0.641165742156689,0.555265820743996,0.641165742156689,
0.555265820743996,0.641165742156689,0.555265820743996,0.641165742156689,
0.555265820743996,0.641165742156689,0.555265820743996,0.641165742156689,
0.555265820743996,0.641165742156689,0.555265820743996,0.641165742156689,
0.555265820743996,0.641165742156689,0.555265820743996,0.641165742156689,
0.555265820743996,0.641165742156689,0.555265820743996,0.641165742156689,
0.555265820743996,0.641165742156689,0.555265820743996,0.641165742156689,
0.555265820743996,0.641165742156689,0.555265820743996,0.641165742156689,
0.555265820743996,0.641165742156689,0.555265820743996,0.641165742156689,
0.555265820743996,0.641165742156689,0.555265820743996,0.641165742156689,
0.555265820743996,0.641165742156689,0.555265820743996,0.641165742156689,
0.555265820743996,0.641165742156689,0.555265820743996,0.641165742156689,
0.555265820743996,0.641165742156689,0.555265820743996,0.641165742156689,
0.555265820743996,0.641165742156689,0.555265820743996,0.641165742156689,
0.555265820743996,0.641165742156689,0.555265820743996,0.641165742156689,
0.555265820743996,0.641165742156689,0.555265820743996,0.641165742156689,
0.555265820743996,0.641165742156689,0.555265820743996,0.641165742156689,
0.555265820743996,0.641165742156689,0.555265820743996,0.641165742156689,
0.555265820743996,0.641165742156689,0.555265820743996,0.641165742156689,
0.555265820743996,0.641165742156689,0.555265820743996,0.641165742156689,
0.555265820743996,0.641165742156689,0.555265820743996,0.641165742156689,
0.555265820743996,0.641165742156689,0.555265820743996,0.641165742156689,
0.555265820743996,0.641165742156689,0.555265820743996,0.641165742156689,
0.555265820743996,0.641165742156689,0.555265820743996,0.641165742156689,
0.555265820743996,0.641165742156689,0.555265820743996,0.641165742156689,
0.555265820743996,0.641165742156689,0.555265820743996,0.641165742156689,
0.555265820743996,0.641165742156689,0.555265820743996,0.641165742156689,
0.555265820743996,0.641165742156689,0.555265820743996,0.641165742156689,
0.555265820743996,0.641165742156689,0.555265820743996,0.641165742156689,
0.555265820743996,0.641165742156689,0.555265820743996,0.641165742156689,
0.555265820743996,0.641165742156689,0.555265820743996,0.641165742156689,
0.555265820743996,0.641165742156689,0.555265820743996,0.641165742156689,
0.555265820743996,0.641165742156689,0.555265820743996,0.641165742156689,
0.555265820743996,0.641165742156689,0.555265820743996,0.641165742156689,
0.555265820743996,0.641165742156689,0.555265820743996,0.641165742156689,
0.555265820743996,0.641165742156689,0.555265820743996,0.641165742156689,
0.555265820743996,0.641165742156689,0.555265820743996,0.641165742156689,
0.555265820743996,0.641165742156689,0.555265820743996,0.641165742156689,
0.555265820743996,0.641165742156689,0.555265820743996,0.641165742156689,
0.555265820743996,0.641165742156689,0.555265820743996,0.641165742156689,
0.555265820743996,0.641165742156689,0.555265820743996,0.641165742156689,
0.555265820743996,0.641165742156689,0.555265820743996,0.641165742156689,
0.555265820743996,0.641165742156689,0.555265820743996,0.641165742156689,
0.555265820743996,0.641165742156689,0.555265820743996,0.641165742156689,
0.555265820743996,0.641165742156689,0.555265820743996,0.641165742156689,
0.555265820743996,0.641165742156689,0.555265820743996,0.641165742156689,
0.555265820743996,0.641165742156689,0.555265820743996,0.641165742156689,
0.555265820743996,0.641165742156689,0.555265820743996,0.641165742156689,
0.555265820743996,0.641165742156689,0.555265820743996,0.641165742156689,
0.555265820743996,0.641165742156689,0.555265820743996,0.641165742156689,
0.555265820743996,0.641165742156689,0.555265820743996,0.641165742156689,
0.555265820743996,0.641165742156689,0.555265820743996,0.641165742156689,
0.555265820743996,0.641165742156689,0.555265820743996,0.641165742156689,
0.555265820743996,0.641165742156689,0.555265820743996,0.641165742156689,
0.555265820743996,0.641165742156689,0.555265820743996,0.641165742156689,
0.555265820743996,0.641165742156689,0.555265820743996,0.641165742156689,
0.555265820743996,0.641165742156689,0.555265820743996,0.641165742156689,
0.555265820743996,0.641165742156689,0.555265820743996,0.641165742156689,
0.555265820743996,0.641165742156689),(1.,0.866025403784439,1.,0.866025403784439,
1.,0.866025403784439,1.,0.866025403784439,1.,0.866025403784439,1.,0.866025403784439,
1.,0.866025403784439,1.,0.866025403784439,1.,0.866025403784439,1.,0.866025403784439,
1.,0.866025403784439,1.,0.866025403784439,1.,0.866025403784439,1.,0.866025403784439,
1.,0.866025403784439,1.,0.866025403784439,1.,0.866025403784439,1.,0.866025403784439,
1.,0.866025403784439,1.,0.866025403784439,1.,0.866025403784439,1.,0.866025403784439,
1.,0.866025403784439,1.,0.866025403784439,1.,0.866025403784439,1.,0.866025403784439,
1.,0.866025403784439,1.,0.866025403784439,1.,0.866025403784439,1.,0.866025403784439,
1.,0.866025403784439,1.,0.866025403784439,1.,0.866025403784439,1.,0.866025403784439,
1.,0.866025403784439,1.,0.866025403784439,1.,0.866025403784439,1.,0.866025403784439,
1.,0.866025403784439,1.,0.866025403784439,1.,0.866025403784439,1.,0.866025403784439,
1.,0.866025403784439,1.,0.866025403784439,1.,0.866025403784439,1.,0.866025403784439,
1.,0.866025403784439,1.,0.866025403784439,1.,0.866025403784439,1.,0.866025403784439,
1.,0.866025403784439,1.,0.866025403784439,1.,0.866025403784439,1.,0.866025403784439,
1.,0.866025403784439,1.,0.866025403784439,1.,0.866025403784439,1.,0.866025403784439,
1.,0.866025403784439,1.,0.866025403784439,1.,0.866025403784439,1.,0.866025403784439,
1.,0.866025403784439,1.,0.866025403784439,1.,0.866025403784439,1.,0.866025403784439,
1.,0.866025403784439,1.,0.866025403784439,1.,0.866025403784439,1.,0.866025403784439,
1.,0.866025403784439,1.,0.866025403784439,1.,0.866025403784439,1.,0.866025403784439,
1.,0.866025403784439,1.,0.866025403784439,1.,0.866025403784439,1.,0.866025403784439,
1.,0.866025403784439,1.,0.866025403784439,1.,0.866025403784439,1.,0.866025403784439,
1.,0.866025403784439,1.,0.866025403784439,1.,0.866025403784439,1.,0.866025403784439,
1.,0.866025403784439,1.,0.866025403784439,1.,0.866025403784439,1.,0.866025403784439,
1.,0.866025403784439,1.,0.866025403784439,1.,0.866025403784439,1.,0.866025403784439,
1.,0.866025403784439,1.,0.866025403784439,1.,0.866025403784439,1.,0.866025403784439,
1.,0.866025403784439,1.,0.866025403784439,1.,0.866025403784439,1.,0.866025403784439,
1.,0.866025403784439,1.,0.866025403784439,1.,0.866025403784439,1.,0.866025403784439,
1.,0.866025403784439,1.,0.866025403784439,1.,0.866025403784439,1.,0.866025403784439,
1.,0.866025403784439,1.,0.866025403784439,1.,0.866025403784439,1.,0.866025403784439,
1.,0.866025403784439,1.,0.866025403784439,1.,0.866025403784439,1.,0.866025403784439,
1.,0.866025403784439,1.,0.866025403784439,1.,0.866025403784439,1.,0.866025403784439,
1.,0.866025403784439,1.,0.866025403784439,1.,0.866025403784439,1.,0.866025403784439,
1.,0.866025403784439,1.,0.866025403784439,1.,0.866025403784439,1.,0.866025403784439,
1.,0.866025403784439,1.,0.866025403784439,1.,0.866025403784439,1.,0.866025403784439,
1.,0.866025403784439,1.,0.866025403784439,1.,0.866025403784439,1.,0.866025403784439,
1.,0.866025403784439,1.,0.866025403784439,1.,0.866025403784439,1.,0.866025403784439,
1.,0.866025403784439,1.,0.866025403784439,1.,0.866025403784439,1.,0.866025403784439,
1.,0.866025403784439,1.,0.866025403784439,1.,0.866025403784439,1.,0.866025403784439,
1.,0.866025403784439,1.,0.866025403784439,1.,0.866025403784439,1.,0.866025403784439,
1.,0.866025403784439,1.,0.866025403784439,1.,0.866025403784439,1.,0.866025403784439,
1.,0.866025403784439,1.,0.866025403784439,1.,0.866025403784439,1.,0.866025403784439,
1.,0.866025403784439,1.,0.866025403784439,1.,0.866025403784439,1.,0.866025403784439,
1.,0.866025403784439,1.,0.866025403784439,1.,0.866025403784439,1.,0.866025403784439,
1.,0.866025403784439,1.,0.866025403784439,1.,0.866025403784439,1.,0.866025403784439,
1.,0.866025403784439,1.,0.866025403784439,1.,0.866025403784439,1.,0.866025403784439,
1.,0.866025403784439,1.,0.866025403784439,1.,0.866025403784439,1.,0.866025403784439,
1.,0.866025403784439,1.,0.866025403784439,1.,0.866025403784439,1.,0.866025403784439,
1.,0.866025403784439,1.,0.866025403784439,1.,0.866025403784439,1.,0.866025403784439,
1.,0.866025403784439,1.,0.866025403784439,1.,0.866025403784439,1.,0.866025403784439,
1.,0.866025403784439,1.,0.866025403784439,1.,0.866025403784439,1.,0.866025403784439,
1.,0.866025403784439,1.,0.866025403784439,1.,0.866025403784439,1.,0.866025403784439,
1.,0.866025403784439,1.,0.866025403784439,1.,0.866025403784439,1.,0.866025403784439,
1.,0.866025403784439,1.,0.866025403784439,1.,0.866025403784439,1.,0.866025403784439,
1.,0.866025403784439,1.,0.866025403784439,1.,0.866025403784439,1.,0.866025403784439,
1.,0.866025403784439,1.,0.866025403784439,1.,0.866025403784439,1.,0.866025403784439,
1.,0.866025403784439,1.,0.866025403784439,1.,0.866025403784439,1.,0.866025403784439,
1.,0.866025403784439,1.,0.866025403784439,1.,0.866025403784439,1.,0.866025403784439,
1.,0.866025403784439,1.,0.866025403784439,1.,0.866025403784439,1.,0.866025403784439,
1.,0.866025403784439,1.,0.866025403784439,1.,0.866025403784439,1.,0.866025403784439,
1.,0.866025403784439,1.,0.866025403784439,1.,0.866025403784439,1.,0.866025403784439,
1.,0.866025403784439,1.,0.866025403784439,1.,0.866025403784439,1.,0.866025403784439,
1.,0.866025403784439,1.,0.866025403784439,1.,0.866025403784439,1.,0.866025403784439,
1.,0.866025403784439,1.,0.866025403784439,1.,0.866025403784439,1.,0.866025403784439,
1.,0.866025403784439,1.,0.866025403784439,1.,0.866025403784439,1.,0.866025403784439,
1.,0.866025403784439,1.,0.866025403784439,1.,0.866025403784439,1.,0.866025403784439,
1.,0.866025403784439,1.,0.866025403784439,1.,0.866025403784439,1.,0.866025403784439,
1.,0.866025403784439,1.,0.866025403784439,1.,0.866025403784439,1.,0.866025403784439,
1.,0.866025403784439,1.,0.866025403784439,1.,0.866025403784439,1.,0.866025403784439,
1.,0.866025403784439,1.,0.866025403784439,1.,0.866025403784439,1.,0.866025403784439,
1.,0.866025403784439,1.,0.866025403784439,1.,0.866025403784439,1.,0.866025403784439,
1.,0.866025403784439,1.,0.866025403784439,1.,0.866025403784439,1.,0.866025403784439,
1.,0.866025403784439,1.,0.866025403784439,1.,0.866025403784439,1.,0.866025403784439,
1.,0.866025403784439,1.,0.866025403784439,1.,0.866025403784439,1.,0.866025403784439,
1.,0.866025403784439,1.,0.866025403784439,1.,0.866025403784439,1.,0.866025403784439,
1.,0.866025403784439,1.,0.866025403784439,1.,0.866025403784439,1.,0.866025403784439,
1.,0.866025403784439,1.,0.866025403784439,1.,0.866025403784439,1.,0.866025403784439,
1.,0.866025403784439,1.,0.866025403784439,1.,0.866025403784439,1.,0.866025403784439,
1.,0.866025403784439,1.,0.866025403784439,1.,0.866025403784439,1.,0.866025403784439,
1.,0.866025403784439,1.,0.866025403784439,1.,0.866025403784439,1.,0.866025403784439,
1.,0.866025403784439,1.,0.866025403784439,1.,0.866025403784439,1.,0.866025403784439,
1.,0.866025403784439,1.,0.866025403784439,1.,0.866025403784439,1.,0.866025403784439,
1.,0.866025403784439,1.,0.866025403784439,1.,0.866025403784439,1.,0.866025403784439,
1.,0.866025403784439,1.,0.866025403784439,1.,0.866025403784439,1.,0.866025403784439,
1.,0.866025403784439,1.,0.866025403784439,1.,0.866025403784439,1.,0.866025403784439,
1.,0.866025403784439,1.,0.866025403784439,1.,0.866025403784439,1.,0.866025403784439,
1.,0.866025403784439,1.,0.866025403784439,1.,0.866025403784439,1.,0.866025403784439,
1.,0.866025403784439,1.,0.866025403784439,1.,0.866025403784439,1.,0.866025403784439,
1.,0.866025403784439,1.,0.866025403784439,1.,0.866025403784439,1.,0.866025403784439,
1.,0.866025403784439,1.,0.866025403784439,1.,0.866025403784439,1.,0.866025403784439,
1.,0.866025403784439,1.,0.866025403784439,1.,0.866025403784439,1.,0.866025403784439,
1.,0.866025403784439,1.,0.866025403784439,1.,0.866025403784439,1.,0.866025403784439,
1.,0.866025403784439,1.,0.866025403784439,1.,0.866025403784439,1.,0.866025403784439,
1.,0.866025403784439,1.,0.866025403784439,1.,0.866025403784439,1.,0.866025403784439,
1.,0.866025403784439,1.,0.866025403784439,1.,0.866025403784439,1.,0.866025403784439,
1.,0.866025403784439,1.,0.866025403784439,1.,0.866025403784439,1.,0.866025403784439,
1.,0.866025403784439,1.,0.866025403784439,1.,0.866025403784439,1.,0.866025403784439,
1.,0.866025403784439,1.,0.866025403784439,1.,0.866025403784439,1.,0.866025403784439,
1.,0.866025403784439,1.,0.866025403784439,1.,0.866025403784439,1.,0.866025403784439,
1.,0.866025403784439,1.,0.866025403784439,1.,0.866025403784439,1.,0.866025403784439,
1.,0.866025403784439,1.,0.866025403784439,1.,0.866025403784439,1.,0.866025403784439,
1.,0.866025403784439,1.,0.866025403784439,1.,0.866025403784439,1.,0.866025403784439,
1.,0.866025403784439,1.,0.866025403784439,1.,0.866025403784439,1.,0.866025403784439,
1.,0.866025403784439,1.,0.866025403784439,1.,0.866025403784439,1.,0.866025403784439,
1.,0.866025403784439,1.,0.866025403784439,1.,0.866025403784439,1.,0.866025403784439,
1.,0.866025403784439,1.,0.866025403784439,1.,0.866025403784439,1.,0.866025403784439,
1.,0.866025403784439,1.,0.866025403784439,1.,0.866025403784439,1.,0.866025403784439,
1.,0.866025403784439,1.,0.866025403784439,1.,0.866025403784439,1.,0.866025403784439,
1.,0.866025403784439,1.,0.866025403784439,1.,0.866025403784439,1.,0.866025403784439,
1.,0.866025403784439,1.,0.866025403784439,1.,0.866025403784439,1.,0.866025403784439,
1.,0.866025403784439,1.,0.866025403784439,1.,0.866025403784439,1.,0.866025403784439,
1.,0.866025403784439,1.,0.866025403784439,1.,0.866025403784439,1.,0.866025403784439,
1.,0.866025403784439,1.,0.866025403784439,1.,0.866025403784439,1.,0.866025403784439,
1.,0.866025403784439,1.,0.866025403784439,1.,0.866025403784439,1.,0.866025403784439,
1.,0.866025403784439,1.,0.866025403784439,1.,0.866025403784439,1.,0.866025403784439,
1.,0.866025403784439,1.,0.866025403784439,1.,0.866025403784439,1.,0.866025403784439,
1.,0.866025403784439,1.,0.866025403784439,1.,0.866025403784439,1.,0.866025403784439,
1.,0.866025403784439,1.,0.866025403784439,1.,0.866025403784439,1.,0.866025403784439,
1.,0.866025403784439,1.,0.866025403784439,1.,0.866025403784439,1.,0.866025403784439,
1.,0.866025403784439,1.,0.866025403784439,1.,0.866025403784439,1.,0.866025403784439,
1.,0.866025403784439,1.,0.866025403784439,1.,0.866025403784439,1.,0.866025403784439,
1.,0.866025403784439,1.,0.866025403784439,1.,0.866025403784439,1.,0.866025403784439,
1.,0.866025403784439,1.,0.866025403784439,1.,0.866025403784439,1.,0.866025403784439,
1.)))
REPRESENTATION_ITEM('')
SURFACE()
);
#180=(
BOUNDED_SURFACE()
B_SPLINE_SURFACE(1,2,((#37476,#37477,#37478,#37479,#37480,#37481,#37482,
#37483,#37484,#37485,#37486,#37487,#37488,#37489,#37490,#37491,#37492,#37493,
#37494,#37495,#37496,#37497,#37498,#37499,#37500,#37501,#37502,#37503,#37504,
#37505,#37506,#37507,#37508,#37509,#37510,#37511,#37512,#37513,#37514,#37515,
#37516,#37517,#37518,#37519,#37520,#37521,#37522,#37523,#37524,#37525,#37526,
#37527,#37528,#37529,#37530,#37531,#37532,#37533,#37534,#37535,#37536,#37537,
#37538,#37539,#37540,#37541,#37542,#37543,#37544,#37545,#37546,#37547,#37548,
#37549,#37550,#37551,#37552,#37553,#37554,#37555,#37556,#37557,#37558,#37559,
#37560,#37561,#37562,#37563,#37564,#37565,#37566,#37567,#37568,#37569,#37570,
#37571,#37572,#37573,#37574,#37575,#37576,#37577,#37578,#37579,#37580,#37581,
#37582,#37583,#37584,#37585,#37586,#37587,#37588,#37589,#37590,#37591,#37592,
#37593,#37594,#37595,#37596,#37597,#37598,#37599,#37600,#37601,#37602,#37603,
#37604,#37605,#37606,#37607,#37608,#37609,#37610,#37611,#37612,#37613,#37614,
#37615,#37616,#37617,#37618,#37619,#37620,#37621,#37622,#37623,#37624,#37625,
#37626,#37627,#37628,#37629,#37630,#37631,#37632,#37633,#37634,#37635,#37636,
#37637,#37638,#37639,#37640,#37641,#37642,#37643,#37644,#37645,#37646,#37647,
#37648,#37649,#37650,#37651,#37652,#37653,#37654,#37655,#37656,#37657,#37658,
#37659,#37660,#37661,#37662,#37663,#37664,#37665,#37666,#37667,#37668,#37669,
#37670,#37671,#37672,#37673,#37674,#37675,#37676,#37677,#37678,#37679,#37680,
#37681,#37682,#37683,#37684,#37685,#37686,#37687,#37688,#37689,#37690,#37691,
#37692,#37693,#37694,#37695,#37696,#37697,#37698,#37699,#37700,#37701,#37702,
#37703,#37704,#37705,#37706,#37707,#37708,#37709,#37710,#37711,#37712,#37713,
#37714,#37715,#37716,#37717,#37718,#37719,#37720,#37721,#37722,#37723,#37724,
#37725,#37726,#37727,#37728,#37729,#37730,#37731,#37732,#37733,#37734,#37735,
#37736,#37737,#37738,#37739,#37740,#37741,#37742,#37743,#37744,#37745,#37746,
#37747,#37748,#37749,#37750,#37751,#37752,#37753,#37754,#37755,#37756,#37757,
#37758,#37759,#37760,#37761,#37762,#37763,#37764,#37765,#37766,#37767,#37768,
#37769,#37770,#37771,#37772,#37773,#37774,#37775,#37776,#37777,#37778,#37779,
#37780,#37781,#37782,#37783,#37784,#37785,#37786,#37787,#37788,#37789,#37790,
#37791,#37792,#37793,#37794,#37795,#37796,#37797,#37798,#37799,#37800,#37801,
#37802,#37803,#37804,#37805,#37806,#37807,#37808,#37809,#37810,#37811,#37812,
#37813,#37814,#37815,#37816,#37817,#37818,#37819,#37820,#37821,#37822,#37823,
#37824,#37825,#37826,#37827,#37828,#37829,#37830,#37831,#37832,#37833,#37834,
#37835,#37836,#37837,#37838,#37839,#37840,#37841,#37842,#37843,#37844,#37845,
#37846,#37847,#37848,#37849,#37850,#37851,#37852,#37853,#37854,#37855,#37856,
#37857,#37858,#37859,#37860,#37861,#37862,#37863,#37864,#37865,#37866,#37867,
#37868,#37869,#37870,#37871,#37872,#37873,#37874,#37875,#37876,#37877,#37878,
#37879,#37880,#37881,#37882,#37883,#37884,#37885,#37886,#37887,#37888,#37889,
#37890,#37891,#37892,#37893,#37894,#37895,#37896,#37897,#37898,#37899,#37900,
#37901,#37902,#37903,#37904,#37905,#37906,#37907,#37908,#37909,#37910,#37911,
#37912,#37913,#37914,#37915,#37916,#37917,#37918,#37919,#37920,#37921,#37922,
#37923,#37924,#37925,#37926,#37927,#37928,#37929,#37930,#37931,#37932,#37933,
#37934,#37935,#37936,#37937,#37938,#37939,#37940,#37941,#37942,#37943,#37944,
#37945,#37946,#37947,#37948,#37949,#37950,#37951,#37952,#37953,#37954,#37955,
#37956,#37957,#37958,#37959,#37960,#37961,#37962,#37963,#37964,#37965,#37966,
#37967,#37968,#37969,#37970,#37971,#37972,#37973,#37974,#37975,#37976,#37977,
#37978,#37979,#37980,#37981,#37982,#37983,#37984,#37985,#37986,#37987,#37988,
#37989,#37990,#37991,#37992,#37993,#37994,#37995,#37996,#37997,#37998,#37999,
#38000,#38001,#38002,#38003,#38004,#38005,#38006,#38007,#38008,#38009,#38010,
#38011,#38012,#38013,#38014,#38015,#38016,#38017,#38018,#38019,#38020,#38021,
#38022,#38023,#38024,#38025,#38026,#38027,#38028,#38029,#38030,#38031,#38032,
#38033,#38034,#38035,#38036,#38037,#38038,#38039,#38040,#38041,#38042,#38043,
#38044,#38045,#38046,#38047,#38048,#38049,#38050,#38051,#38052,#38053,#38054,
#38055,#38056,#38057,#38058,#38059,#38060,#38061,#38062,#38063,#38064,#38065,
#38066,#38067,#38068,#38069,#38070,#38071,#38072,#38073,#38074,#38075,#38076,
#38077,#38078,#38079,#38080,#38081,#38082,#38083,#38084,#38085,#38086,#38087,
#38088,#38089,#38090,#38091,#38092,#38093,#38094,#38095,#38096,#38097,#38098,
#38099,#38100,#38101,#38102,#38103,#38104,#38105,#38106,#38107,#38108,#38109,
#38110,#38111,#38112,#38113,#38114,#38115,#38116,#38117,#38118,#38119,#38120,
#38121,#38122,#38123,#38124,#38125,#38126,#38127,#38128,#38129,#38130,#38131,
#38132,#38133,#38134,#38135,#38136,#38137,#38138,#38139,#38140,#38141,#38142,
#38143,#38144,#38145,#38146,#38147,#38148,#38149,#38150,#38151,#38152,#38153,
#38154,#38155,#38156,#38157,#38158,#38159,#38160,#38161,#38162,#38163,#38164,
#38165,#38166,#38167,#38168,#38169,#38170,#38171,#38172,#38173,#38174,#38175,
#38176,#38177,#38178,#38179,#38180,#38181,#38182,#38183,#38184,#38185,#38186,
#38187,#38188,#38189,#38190,#38191,#38192,#38193,#38194,#38195,#38196,#38197,
#38198,#38199,#38200,#38201,#38202,#38203,#38204,#38205,#38206,#38207,#38208,
#38209,#38210,#38211,#38212,#38213,#38214,#38215,#38216,#38217,#38218,#38219,
#38220,#38221,#38222,#38223,#38224,#38225,#38226,#38227,#38228,#38229,#38230,
#38231,#38232,#38233,#38234,#38235,#38236,#38237,#38238,#38239,#38240,#38241,
#38242,#38243,#38244,#38245,#38246,#38247,#38248,#38249,#38250,#38251,#38252,
#38253,#38254,#38255,#38256,#38257,#38258,#38259,#38260,#38261,#38262,#38263,
#38264,#38265,#38266,#38267,#38268,#38269,#38270,#38271,#38272,#38273,#38274,
#38275,#38276,#38277,#38278,#38279,#38280,#38281,#38282,#38283,#38284,#38285,
#38286,#38287,#38288,#38289,#38290,#38291,#38292,#38293,#38294,#38295,#38296,
#38297,#38298,#38299,#38300,#38301,#38302,#38303,#38304,#38305,#38306,#38307,
#38308,#38309,#38310,#38311,#38312,#38313,#38314,#38315,#38316,#38317,#38318,
#38319,#38320,#38321,#38322,#38323,#38324,#38325,#38326,#38327,#38328,#38329,
#38330,#38331,#38332,#38333,#38334,#38335,#38336,#38337,#38338,#38339,#38340,
#38341,#38342,#38343,#38344,#38345,#38346,#38347,#38348,#38349,#38350,#38351,
#38352,#38353,#38354,#38355,#38356,#38357,#38358,#38359,#38360,#38361,#38362,
#38363,#38364,#38365,#38366,#38367,#38368,#38369,#38370,#38371,#38372,#38373,
#38374,#38375,#38376,#38377,#38378,#38379,#38380,#38381,#38382,#38383,#38384,
#38385,#38386,#38387,#38388,#38389,#38390,#38391,#38392,#38393,#38394,#38395,
#38396,#38397,#38398,#38399,#38400,#38401,#38402,#38403,#38404,#38405,#38406,
#38407,#38408,#38409,#38410,#38411,#38412,#38413,#38414,#38415,#38416,#38417,
#38418,#38419,#38420,#38421,#38422,#38423,#38424,#38425,#38426,#38427,#38428,
#38429,#38430,#38431,#38432,#38433,#38434,#38435,#38436,#38437,#38438,#38439,
#38440,#38441,#38442,#38443,#38444,#38445,#38446,#38447,#38448),(#38449,
#38450,#38451,#38452,#38453,#38454,#38455,#38456,#38457,#38458,#38459,#38460,
#38461,#38462,#38463,#38464,#38465,#38466,#38467,#38468,#38469,#38470,#38471,
#38472,#38473,#38474,#38475,#38476,#38477,#38478,#38479,#38480,#38481,#38482,
#38483,#38484,#38485,#38486,#38487,#38488,#38489,#38490,#38491,#38492,#38493,
#38494,#38495,#38496,#38497,#38498,#38499,#38500,#38501,#38502,#38503,#38504,
#38505,#38506,#38507,#38508,#38509,#38510,#38511,#38512,#38513,#38514,#38515,
#38516,#38517,#38518,#38519,#38520,#38521,#38522,#38523,#38524,#38525,#38526,
#38527,#38528,#38529,#38530,#38531,#38532,#38533,#38534,#38535,#38536,#38537,
#38538,#38539,#38540,#38541,#38542,#38543,#38544,#38545,#38546,#38547,#38548,
#38549,#38550,#38551,#38552,#38553,#38554,#38555,#38556,#38557,#38558,#38559,
#38560,#38561,#38562,#38563,#38564,#38565,#38566,#38567,#38568,#38569,#38570,
#38571,#38572,#38573,#38574,#38575,#38576,#38577,#38578,#38579,#38580,#38581,
#38582,#38583,#38584,#38585,#38586,#38587,#38588,#38589,#38590,#38591,#38592,
#38593,#38594,#38595,#38596,#38597,#38598,#38599,#38600,#38601,#38602,#38603,
#38604,#38605,#38606,#38607,#38608,#38609,#38610,#38611,#38612,#38613,#38614,
#38615,#38616,#38617,#38618,#38619,#38620,#38621,#38622,#38623,#38624,#38625,
#38626,#38627,#38628,#38629,#38630,#38631,#38632,#38633,#38634,#38635,#38636,
#38637,#38638,#38639,#38640,#38641,#38642,#38643,#38644,#38645,#38646,#38647,
#38648,#38649,#38650,#38651,#38652,#38653,#38654,#38655,#38656,#38657,#38658,
#38659,#38660,#38661,#38662,#38663,#38664,#38665,#38666,#38667,#38668,#38669,
#38670,#38671,#38672,#38673,#38674,#38675,#38676,#38677,#38678,#38679,#38680,
#38681,#38682,#38683,#38684,#38685,#38686,#38687,#38688,#38689,#38690,#38691,
#38692,#38693,#38694,#38695,#38696,#38697,#38698,#38699,#38700,#38701,#38702,
#38703,#38704,#38705,#38706,#38707,#38708,#38709,#38710,#38711,#38712,#38713,
#38714,#38715,#38716,#38717,#38718,#38719,#38720,#38721,#38722,#38723,#38724,
#38725,#38726,#38727,#38728,#38729,#38730,#38731,#38732,#38733,#38734,#38735,
#38736,#38737,#38738,#38739,#38740,#38741,#38742,#38743,#38744,#38745,#38746,
#38747,#38748,#38749,#38750,#38751,#38752,#38753,#38754,#38755,#38756,#38757,
#38758,#38759,#38760,#38761,#38762,#38763,#38764,#38765,#38766,#38767,#38768,
#38769,#38770,#38771,#38772,#38773,#38774,#38775,#38776,#38777,#38778,#38779,
#38780,#38781,#38782,#38783,#38784,#38785,#38786,#38787,#38788,#38789,#38790,
#38791,#38792,#38793,#38794,#38795,#38796,#38797,#38798,#38799,#38800,#38801,
#38802,#38803,#38804,#38805,#38806,#38807,#38808,#38809,#38810,#38811,#38812,
#38813,#38814,#38815,#38816,#38817,#38818,#38819,#38820,#38821,#38822,#38823,
#38824,#38825,#38826,#38827,#38828,#38829,#38830,#38831,#38832,#38833,#38834,
#38835,#38836,#38837,#38838,#38839,#38840,#38841,#38842,#38843,#38844,#38845,
#38846,#38847,#38848,#38849,#38850,#38851,#38852,#38853,#38854,#38855,#38856,
#38857,#38858,#38859,#38860,#38861,#38862,#38863,#38864,#38865,#38866,#38867,
#38868,#38869,#38870,#38871,#38872,#38873,#38874,#38875,#38876,#38877,#38878,
#38879,#38880,#38881,#38882,#38883,#38884,#38885,#38886,#38887,#38888,#38889,
#38890,#38891,#38892,#38893,#38894,#38895,#38896,#38897,#38898,#38899,#38900,
#38901,#38902,#38903,#38904,#38905,#38906,#38907,#38908,#38909,#38910,#38911,
#38912,#38913,#38914,#38915,#38916,#38917,#38918,#38919,#38920,#38921,#38922,
#38923,#38924,#38925,#38926,#38927,#38928,#38929,#38930,#38931,#38932,#38933,
#38934,#38935,#38936,#38937,#38938,#38939,#38940,#38941,#38942,#38943,#38944,
#38945,#38946,#38947,#38948,#38949,#38950,#38951,#38952,#38953,#38954,#38955,
#38956,#38957,#38958,#38959,#38960,#38961,#38962,#38963,#38964,#38965,#38966,
#38967,#38968,#38969,#38970,#38971,#38972,#38973,#38974,#38975,#38976,#38977,
#38978,#38979,#38980,#38981,#38982,#38983,#38984,#38985,#38986,#38987,#38988,
#38989,#38990,#38991,#38992,#38993,#38994,#38995,#38996,#38997,#38998,#38999,
#39000,#39001,#39002,#39003,#39004,#39005,#39006,#39007,#39008,#39009,#39010,
#39011,#39012,#39013,#39014,#39015,#39016,#39017,#39018,#39019,#39020,#39021,
#39022,#39023,#39024,#39025,#39026,#39027,#39028,#39029,#39030,#39031,#39032,
#39033,#39034,#39035,#39036,#39037,#39038,#39039,#39040,#39041,#39042,#39043,
#39044,#39045,#39046,#39047,#39048,#39049,#39050,#39051,#39052,#39053,#39054,
#39055,#39056,#39057,#39058,#39059,#39060,#39061,#39062,#39063,#39064,#39065,
#39066,#39067,#39068,#39069,#39070,#39071,#39072,#39073,#39074,#39075,#39076,
#39077,#39078,#39079,#39080,#39081,#39082,#39083,#39084,#39085,#39086,#39087,
#39088,#39089,#39090,#39091,#39092,#39093,#39094,#39095,#39096,#39097,#39098,
#39099,#39100,#39101,#39102,#39103,#39104,#39105,#39106,#39107,#39108,#39109,
#39110,#39111,#39112,#39113,#39114,#39115,#39116,#39117,#39118,#39119,#39120,
#39121,#39122,#39123,#39124,#39125,#39126,#39127,#39128,#39129,#39130,#39131,
#39132,#39133,#39134,#39135,#39136,#39137,#39138,#39139,#39140,#39141,#39142,
#39143,#39144,#39145,#39146,#39147,#39148,#39149,#39150,#39151,#39152,#39153,
#39154,#39155,#39156,#39157,#39158,#39159,#39160,#39161,#39162,#39163,#39164,
#39165,#39166,#39167,#39168,#39169,#39170,#39171,#39172,#39173,#39174,#39175,
#39176,#39177,#39178,#39179,#39180,#39181,#39182,#39183,#39184,#39185,#39186,
#39187,#39188,#39189,#39190,#39191,#39192,#39193,#39194,#39195,#39196,#39197,
#39198,#39199,#39200,#39201,#39202,#39203,#39204,#39205,#39206,#39207,#39208,
#39209,#39210,#39211,#39212,#39213,#39214,#39215,#39216,#39217,#39218,#39219,
#39220,#39221,#39222,#39223,#39224,#39225,#39226,#39227,#39228,#39229,#39230,
#39231,#39232,#39233,#39234,#39235,#39236,#39237,#39238,#39239,#39240,#39241,
#39242,#39243,#39244,#39245,#39246,#39247,#39248,#39249,#39250,#39251,#39252,
#39253,#39254,#39255,#39256,#39257,#39258,#39259,#39260,#39261,#39262,#39263,
#39264,#39265,#39266,#39267,#39268,#39269,#39270,#39271,#39272,#39273,#39274,
#39275,#39276,#39277,#39278,#39279,#39280,#39281,#39282,#39283,#39284,#39285,
#39286,#39287,#39288,#39289,#39290,#39291,#39292,#39293,#39294,#39295,#39296,
#39297,#39298,#39299,#39300,#39301,#39302,#39303,#39304,#39305,#39306,#39307,
#39308,#39309,#39310,#39311,#39312,#39313,#39314,#39315,#39316,#39317,#39318,
#39319,#39320,#39321,#39322,#39323,#39324,#39325,#39326,#39327,#39328,#39329,
#39330,#39331,#39332,#39333,#39334,#39335,#39336,#39337,#39338,#39339,#39340,
#39341,#39342,#39343,#39344,#39345,#39346,#39347,#39348,#39349,#39350,#39351,
#39352,#39353,#39354,#39355,#39356,#39357,#39358,#39359,#39360,#39361,#39362,
#39363,#39364,#39365,#39366,#39367,#39368,#39369,#39370,#39371,#39372,#39373,
#39374,#39375,#39376,#39377,#39378,#39379,#39380,#39381,#39382,#39383,#39384,
#39385,#39386,#39387,#39388,#39389,#39390,#39391,#39392,#39393,#39394,#39395,
#39396,#39397,#39398,#39399,#39400,#39401,#39402,#39403,#39404,#39405,#39406,
#39407,#39408,#39409,#39410,#39411,#39412,#39413,#39414,#39415,#39416,#39417,
#39418,#39419,#39420,#39421)),.UNSPECIFIED.,.F.,.F.,.F.)
B_SPLINE_SURFACE_WITH_KNOTS((2,2),(3,2,2,2,2,2,2,2,2,2,2,2,2,2,2,2,2,2,
2,2,2,2,2,2,2,2,2,2,2,2,2,2,2,2,2,2,2,2,2,2,2,2,2,2,2,2,2,2,2,2,2,2,2,2,
2,2,2,2,2,2,2,2,2,2,2,2,2,2,2,2,2,2,2,2,2,2,2,2,2,2,2,2,2,2,2,2,2,2,2,2,
2,2,2,2,2,2,2,2,2,2,2,2,2,2,2,2,2,2,2,2,2,2,2,2,2,2,2,2,2,2,2,2,2,2,2,2,
2,2,2,2,2,2,2,2,2,2,2,2,2,2,2,2,2,2,2,2,2,2,2,2,2,2,2,2,2,2,2,2,2,2,2,2,
2,2,2,2,2,2,2,2,2,2,2,2,2,2,2,2,2,2,2,2,2,2,2,2,2,2,2,2,2,2,2,2,2,2,2,2,
2,2,2,2,2,2,2,2,2,2,2,2,2,2,2,2,2,2,2,2,2,2,2,2,2,2,2,2,2,2,2,2,2,2,2,2,
2,2,2,2,2,2,2,2,2,2,2,2,2,2,2,2,2,2,2,2,2,2,2,2,2,2,2,2,2,2,2,2,2,2,2,2,
2,2,2,2,2,2,2,2,2,2,2,2,2,2,2,2,2,2,2,2,2,2,2,2,2,2,2,2,2,2,2,2,2,2,2,2,
2,2,2,2,2,2,2,2,2,2,2,2,2,2,2,2,2,2,2,2,2,2,2,2,2,2,2,2,2,2,2,2,2,2,2,2,
2,2,2,2,2,2,2,2,2,2,2,2,2,2,2,2,2,2,2,2,2,2,2,2,2,2,2,2,2,2,2,2,2,2,2,2,
2,2,2,2,2,2,2,2,2,2,2,2,2,2,2,2,2,2,2,2,2,2,2,2,2,2,2,2,2,2,2,2,2,2,2,2,
2,2,2,2,2,2,2,2,2,2,2,2,2,2,2,2,2,2,2,2,2,2,2,2,2,2,2,2,2,2,2,2,2,2,2,2,
2,2,2,2,2,2,2,2,2,2,2,2,2,2,2,2,2,2,2,2,2,2,2,2,2,2,2,2,2,2,2,2,2,2,2,2,
3),(0.,1.),(0.,0.00205761316872428,0.00411522633744856,0.00617283950617284,
0.00823045267489712,0.0102880658436214,0.0123456790123457,0.01440329218107,
0.0164609053497942,0.0185185185185185,0.0205761316872428,0.0226337448559671,
0.0246913580246914,0.0267489711934156,0.0288065843621399,0.0308641975308642,
0.0329218106995885,0.0349794238683128,0.037037037037037,0.0390946502057613,
0.0411522633744856,0.0432098765432099,0.0452674897119342,0.0473251028806584,
0.0493827160493827,0.051440329218107,0.0534979423868313,0.0555555555555556,
0.0576131687242798,0.0596707818930041,0.0617283950617284,0.0637860082304527,
0.065843621399177,0.0679012345679012,0.0699588477366255,0.0720164609053498,
0.0740740740740741,0.0761316872427984,0.0781893004115226,0.0802469135802469,
0.0823045267489712,0.0843621399176955,0.0864197530864197,0.088477366255144,
0.0905349794238683,0.0925925925925926,0.0946502057613169,0.0967078189300412,
0.0987654320987654,0.10082304526749,0.102880658436214,0.104938271604938,
0.106995884773663,0.109053497942387,0.111111111111111,0.113168724279835,
0.11522633744856,0.117283950617284,0.119341563786008,0.121399176954733,
0.123456790123457,0.125514403292181,0.127572016460905,0.12962962962963,
0.131687242798354,0.133744855967078,0.135802469135802,0.137860082304527,
0.139917695473251,0.141975308641975,0.1440329218107,0.146090534979424,0.148148148148148,
0.150205761316872,0.152263374485597,0.154320987654321,0.156378600823045,
0.15843621399177,0.160493827160494,0.162551440329218,0.164609053497942,
0.166666666666667,0.168724279835391,0.170781893004115,0.172839506172839,
0.174897119341564,0.176954732510288,0.179012345679012,0.181069958847737,
0.183127572016461,0.185185185185185,0.187242798353909,0.189300411522634,
0.191358024691358,0.193415637860082,0.195473251028807,0.197530864197531,
0.199588477366255,0.201646090534979,0.203703703703704,0.205761316872428,
0.207818930041152,0.209876543209877,0.211934156378601,0.213991769547325,
0.216049382716049,0.218106995884774,0.220164609053498,0.222222222222222,
0.224279835390947,0.226337448559671,0.228395061728395,0.230452674897119,
0.232510288065844,0.234567901234568,0.236625514403292,0.238683127572016,
0.240740740740741,0.242798353909465,0.244855967078189,0.246913580246914,
0.248971193415638,0.251028806584362,0.253086419753086,0.255144032921811,
0.257201646090535,0.259259259259259,0.261316872427984,0.263374485596708,
0.265432098765432,0.267489711934156,0.269547325102881,0.271604938271605,
0.273662551440329,0.275720164609054,0.277777777777778,0.279835390946502,
0.281893004115226,0.283950617283951,0.286008230452675,0.288065843621399,
0.290123456790123,0.292181069958848,0.294238683127572,0.296296296296296,
0.298353909465021,0.300411522633745,0.302469135802469,0.304526748971193,
0.306584362139918,0.308641975308642,0.310699588477366,0.312757201646091,
0.314814814814815,0.316872427983539,0.318930041152263,0.320987654320988,
0.323045267489712,0.325102880658436,0.327160493827161,0.329218106995885,
0.331275720164609,0.333333333333333,0.335390946502058,0.337448559670782,
0.339506172839506,0.34156378600823,0.343621399176955,0.345679012345679,
0.347736625514403,0.349794238683128,0.351851851851852,0.353909465020576,
0.3559670781893,0.358024691358025,0.360082304526749,0.362139917695473,0.364197530864198,
0.366255144032922,0.368312757201646,0.37037037037037,0.372427983539095,
0.374485596707819,0.376543209876543,0.378600823045267,0.380658436213992,
0.382716049382716,0.38477366255144,0.386831275720165,0.388888888888889,
0.390946502057613,0.393004115226337,0.395061728395062,0.397119341563786,
0.39917695473251,0.401234567901235,0.403292181069959,0.405349794238683,
0.407407407407407,0.409465020576132,0.411522633744856,0.41358024691358,
0.415637860082305,0.417695473251029,0.419753086419753,0.421810699588477,
0.423868312757202,0.425925925925926,0.42798353909465,0.430041152263374,
0.432098765432099,0.434156378600823,0.436213991769547,0.438271604938272,
0.440329218106996,0.44238683127572,0.444444444444444,0.446502057613169,
0.448559670781893,0.450617283950617,0.452674897119342,0.454732510288066,
0.45679012345679,0.458847736625514,0.460905349794239,0.462962962962963,
0.465020576131687,0.467078189300412,0.469135802469136,0.47119341563786,
0.473251028806584,0.475308641975309,0.477366255144033,0.479423868312757,
0.481481481481481,0.483539094650206,0.48559670781893,0.487654320987654,
0.489711934156379,0.491769547325103,0.493827160493827,0.495884773662551,
0.497942386831276,0.5,0.502057613168724,0.504115226337449,0.506172839506173,
0.508230452674897,0.510288065843621,0.512345679012346,0.51440329218107,
0.516460905349794,0.518518518518518,0.520576131687243,0.522633744855967,
0.524691358024691,0.526748971193416,0.52880658436214,0.530864197530864,
0.532921810699588,0.534979423868313,0.537037037037037,0.539094650205761,
0.541152263374486,0.54320987654321,0.545267489711934,0.547325102880658,
0.549382716049383,0.551440329218107,0.553497942386831,0.555555555555556,
0.55761316872428,0.559670781893004,0.561728395061728,0.563786008230453,
0.565843621399177,0.567901234567901,0.569958847736626,0.57201646090535,
0.574074074074074,0.576131687242798,0.578189300411523,0.580246913580247,
0.582304526748971,0.584362139917695,0.58641975308642,0.588477366255144,
0.590534979423868,0.592592592592593,0.594650205761317,0.596707818930041,
0.598765432098765,0.60082304526749,0.602880658436214,0.604938271604938,
0.606995884773663,0.609053497942387,0.611111111111111,0.613168724279835,
0.61522633744856,0.617283950617284,0.619341563786008,0.621399176954732,
0.623456790123457,0.625514403292181,0.627572016460905,0.62962962962963,
0.631687242798354,0.633744855967078,0.635802469135803,0.637860082304527,
0.639917695473251,0.641975308641975,0.6440329218107,0.646090534979424,0.648148148148148,
0.650205761316872,0.652263374485597,0.654320987654321,0.656378600823045,
0.65843621399177,0.660493827160494,0.662551440329218,0.664609053497942,
0.666666666666667,0.668724279835391,0.670781893004115,0.672839506172839,
0.674897119341564,0.676954732510288,0.679012345679012,0.681069958847737,
0.683127572016461,0.685185185185185,0.687242798353909,0.689300411522634,
0.691358024691358,0.693415637860082,0.695473251028807,0.697530864197531,
0.699588477366255,0.701646090534979,0.703703703703704,0.705761316872428,
0.707818930041152,0.709876543209877,0.711934156378601,0.713991769547325,
0.716049382716049,0.718106995884774,0.720164609053498,0.722222222222222,
0.724279835390947,0.726337448559671,0.728395061728395,0.730452674897119,
0.732510288065844,0.734567901234568,0.736625514403292,0.738683127572016,
0.740740740740741,0.742798353909465,0.744855967078189,0.746913580246914,
0.748971193415638,0.751028806584362,0.753086419753086,0.755144032921811,
0.757201646090535,0.759259259259259,0.761316872427984,0.763374485596708,
0.765432098765432,0.767489711934156,0.769547325102881,0.771604938271605,
0.773662551440329,0.775720164609053,0.777777777777778,0.779835390946502,
0.781893004115226,0.783950617283951,0.786008230452675,0.788065843621399,
0.790123456790123,0.792181069958848,0.794238683127572,0.796296296296296,
0.798353909465021,0.800411522633745,0.802469135802469,0.804526748971193,
0.806584362139918,0.808641975308642,0.810699588477366,0.812757201646091,
0.814814814814815,0.816872427983539,0.818930041152263,0.820987654320988,
0.823045267489712,0.825102880658436,0.827160493827161,0.829218106995885,
0.831275720164609,0.833333333333333,0.835390946502058,0.837448559670782,
0.839506172839506,0.84156378600823,0.843621399176955,0.845679012345679,
0.847736625514403,0.849794238683128,0.851851851851852,0.853909465020576,
0.8559670781893,0.858024691358025,0.860082304526749,0.862139917695473,0.864197530864197,
0.866255144032922,0.868312757201646,0.87037037037037,0.872427983539095,
0.874485596707819,0.876543209876543,0.878600823045268,0.880658436213992,
0.882716049382716,0.88477366255144,0.886831275720165,0.888888888888889,
0.890946502057613,0.893004115226337,0.895061728395062,0.897119341563786,
0.89917695473251,0.901234567901235,0.903292181069959,0.905349794238683,
0.907407407407407,0.909465020576132,0.911522633744856,0.91358024691358,
0.915637860082305,0.917695473251029,0.919753086419753,0.921810699588477,
0.923868312757202,0.925925925925926,0.92798353909465,0.930041152263374,
0.932098765432099,0.934156378600823,0.936213991769547,0.938271604938272,
0.940329218106996,0.94238683127572,0.944444444444444,0.946502057613169,
0.948559670781893,0.950617283950617,0.952674897119342,0.954732510288066,
0.95679012345679,0.958847736625514,0.960905349794239,0.962962962962963,
0.965020576131687,0.967078189300412,0.969135802469136,0.97119341563786,
0.973251028806584,0.975308641975309,0.977366255144033,0.979423868312757,
0.981481481481482,0.983539094650206,0.98559670781893,0.987654320987654,
0.989711934156379,0.991769547325103,0.993827160493827,0.995884773662551,
0.997942386831276,1.),.UNSPECIFIED.)
GEOMETRIC_REPRESENTATION_ITEM()
RATIONAL_B_SPLINE_SURFACE(((1.,0.866025403784439,1.,0.866025403784439,1.,
0.866025403784439,1.,0.866025403784439,1.,0.866025403784439,1.,0.866025403784439,
1.,0.866025403784439,1.,0.866025403784439,1.,0.866025403784439,1.,0.866025403784439,
1.,0.866025403784439,1.,0.866025403784439,1.,0.866025403784439,1.,0.866025403784439,
1.,0.866025403784439,1.,0.866025403784439,1.,0.866025403784439,1.,0.866025403784439,
1.,0.866025403784439,1.,0.866025403784439,1.,0.866025403784439,1.,0.866025403784439,
1.,0.866025403784439,1.,0.866025403784439,1.,0.866025403784439,1.,0.866025403784439,
1.,0.866025403784439,1.,0.866025403784439,1.,0.866025403784439,1.,0.866025403784439,
1.,0.866025403784439,1.,0.866025403784439,1.,0.866025403784439,1.,0.866025403784439,
1.,0.866025403784439,1.,0.866025403784439,1.,0.866025403784439,1.,0.866025403784439,
1.,0.866025403784439,1.,0.866025403784439,1.,0.866025403784439,1.,0.866025403784439,
1.,0.866025403784439,1.,0.866025403784439,1.,0.866025403784439,1.,0.866025403784439,
1.,0.866025403784439,1.,0.866025403784439,1.,0.866025403784439,1.,0.866025403784439,
1.,0.866025403784439,1.,0.866025403784439,1.,0.866025403784439,1.,0.866025403784439,
1.,0.866025403784439,1.,0.866025403784439,1.,0.866025403784439,1.,0.866025403784439,
1.,0.866025403784439,1.,0.866025403784439,1.,0.866025403784439,1.,0.866025403784439,
1.,0.866025403784439,1.,0.866025403784439,1.,0.866025403784439,1.,0.866025403784439,
1.,0.866025403784439,1.,0.866025403784439,1.,0.866025403784439,1.,0.866025403784439,
1.,0.866025403784439,1.,0.866025403784439,1.,0.866025403784439,1.,0.866025403784439,
1.,0.866025403784439,1.,0.866025403784439,1.,0.866025403784439,1.,0.866025403784439,
1.,0.866025403784439,1.,0.866025403784439,1.,0.866025403784439,1.,0.866025403784439,
1.,0.866025403784439,1.,0.866025403784439,1.,0.866025403784439,1.,0.866025403784439,
1.,0.866025403784439,1.,0.866025403784439,1.,0.866025403784439,1.,0.866025403784439,
1.,0.866025403784439,1.,0.866025403784439,1.,0.866025403784439,1.,0.866025403784439,
1.,0.866025403784439,1.,0.866025403784439,1.,0.866025403784439,1.,0.866025403784439,
1.,0.866025403784439,1.,0.866025403784439,1.,0.866025403784439,1.,0.866025403784439,
1.,0.866025403784439,1.,0.866025403784439,1.,0.866025403784439,1.,0.866025403784439,
1.,0.866025403784439,1.,0.866025403784439,1.,0.866025403784439,1.,0.866025403784439,
1.,0.866025403784439,1.,0.866025403784439,1.,0.866025403784439,1.,0.866025403784439,
1.,0.866025403784439,1.,0.866025403784439,1.,0.866025403784439,1.,0.866025403784439,
1.,0.866025403784439,1.,0.866025403784439,1.,0.866025403784439,1.,0.866025403784439,
1.,0.866025403784439,1.,0.866025403784439,1.,0.866025403784439,1.,0.866025403784439,
1.,0.866025403784439,1.,0.866025403784439,1.,0.866025403784439,1.,0.866025403784439,
1.,0.866025403784439,1.,0.866025403784439,1.,0.866025403784439,1.,0.866025403784439,
1.,0.866025403784439,1.,0.866025403784439,1.,0.866025403784439,1.,0.866025403784439,
1.,0.866025403784439,1.,0.866025403784439,1.,0.866025403784439,1.,0.866025403784439,
1.,0.866025403784439,1.,0.866025403784439,1.,0.866025403784439,1.,0.866025403784439,
1.,0.866025403784439,1.,0.866025403784439,1.,0.866025403784439,1.,0.866025403784439,
1.,0.866025403784439,1.,0.866025403784439,1.,0.866025403784439,1.,0.866025403784439,
1.,0.866025403784439,1.,0.866025403784439,1.,0.866025403784439,1.,0.866025403784439,
1.,0.866025403784439,1.,0.866025403784439,1.,0.866025403784439,1.,0.866025403784439,
1.,0.866025403784439,1.,0.866025403784439,1.,0.866025403784439,1.,0.866025403784439,
1.,0.866025403784439,1.,0.866025403784439,1.,0.866025403784439,1.,0.866025403784439,
1.,0.866025403784439,1.,0.866025403784439,1.,0.866025403784439,1.,0.866025403784439,
1.,0.866025403784439,1.,0.866025403784439,1.,0.866025403784439,1.,0.866025403784439,
1.,0.866025403784439,1.,0.866025403784439,1.,0.866025403784439,1.,0.866025403784439,
1.,0.866025403784439,1.,0.866025403784439,1.,0.866025403784439,1.,0.866025403784439,
1.,0.866025403784439,1.,0.866025403784439,1.,0.866025403784439,1.,0.866025403784439,
1.,0.866025403784439,1.,0.866025403784439,1.,0.866025403784439,1.,0.866025403784439,
1.,0.866025403784439,1.,0.866025403784439,1.,0.866025403784439,1.,0.866025403784439,
1.,0.866025403784439,1.,0.866025403784439,1.,0.866025403784439,1.,0.866025403784439,
1.,0.866025403784439,1.,0.866025403784439,1.,0.866025403784439,1.,0.866025403784439,
1.,0.866025403784439,1.,0.866025403784439,1.,0.866025403784439,1.,0.866025403784439,
1.,0.866025403784439,1.,0.866025403784439,1.,0.866025403784439,1.,0.866025403784439,
1.,0.866025403784439,1.,0.866025403784439,1.,0.866025403784439,1.,0.866025403784439,
1.,0.866025403784439,1.,0.866025403784439,1.,0.866025403784439,1.,0.866025403784439,
1.,0.866025403784439,1.,0.866025403784439,1.,0.866025403784439,1.,0.866025403784439,
1.,0.866025403784439,1.,0.866025403784439,1.,0.866025403784439,1.,0.866025403784439,
1.,0.866025403784439,1.,0.866025403784439,1.,0.866025403784439,1.,0.866025403784439,
1.,0.866025403784439,1.,0.866025403784439,1.,0.866025403784439,1.,0.866025403784439,
1.,0.866025403784439,1.,0.866025403784439,1.,0.866025403784439,1.,0.866025403784439,
1.,0.866025403784439,1.,0.866025403784439,1.,0.866025403784439,1.,0.866025403784439,
1.,0.866025403784439,1.,0.866025403784439,1.,0.866025403784439,1.,0.866025403784439,
1.,0.866025403784439,1.,0.866025403784439,1.,0.866025403784439,1.,0.866025403784439,
1.,0.866025403784439,1.,0.866025403784439,1.,0.866025403784439,1.,0.866025403784439,
1.,0.866025403784439,1.,0.866025403784439,1.,0.866025403784439,1.,0.866025403784439,
1.,0.866025403784439,1.,0.866025403784439,1.,0.866025403784439,1.,0.866025403784439,
1.,0.866025403784439,1.,0.866025403784439,1.,0.866025403784439,1.,0.866025403784439,
1.,0.866025403784439,1.,0.866025403784439,1.,0.866025403784439,1.,0.866025403784439,
1.,0.866025403784439,1.,0.866025403784439,1.,0.866025403784439,1.,0.866025403784439,
1.,0.866025403784439,1.,0.866025403784439,1.,0.866025403784439,1.,0.866025403784439,
1.,0.866025403784439,1.,0.866025403784439,1.,0.866025403784439,1.,0.866025403784439,
1.,0.866025403784439,1.,0.866025403784439,1.,0.866025403784439,1.,0.866025403784439,
1.,0.866025403784439,1.,0.866025403784439,1.,0.866025403784439,1.,0.866025403784439,
1.,0.866025403784439,1.,0.866025403784439,1.,0.866025403784439,1.,0.866025403784439,
1.,0.866025403784439,1.,0.866025403784439,1.,0.866025403784439,1.,0.866025403784439,
1.,0.866025403784439,1.,0.866025403784439,1.,0.866025403784439,1.,0.866025403784439,
1.,0.866025403784439,1.,0.866025403784439,1.,0.866025403784439,1.,0.866025403784439,
1.,0.866025403784439,1.,0.866025403784439,1.,0.866025403784439,1.,0.866025403784439,
1.,0.866025403784439,1.,0.866025403784439,1.,0.866025403784439,1.,0.866025403784439,
1.,0.866025403784439,1.,0.866025403784439,1.,0.866025403784439,1.,0.866025403784439,
1.,0.866025403784439,1.,0.866025403784439,1.,0.866025403784439,1.,0.866025403784439,
1.,0.866025403784439,1.,0.866025403784439,1.,0.866025403784439,1.,0.866025403784439,
1.,0.866025403784439,1.,0.866025403784439,1.,0.866025403784439,1.,0.866025403784439,
1.,0.866025403784439,1.,0.866025403784439,1.,0.866025403784439,1.,0.866025403784439,
1.,0.866025403784439,1.,0.866025403784439,1.,0.866025403784439,1.,0.866025403784439,
1.,0.866025403784439,1.,0.866025403784439,1.,0.866025403784439,1.,0.866025403784439,
1.,0.866025403784439,1.,0.866025403784439,1.,0.866025403784439,1.,0.866025403784439,
1.,0.866025403784439,1.,0.866025403784439,1.,0.866025403784439,1.,0.866025403784439,
1.,0.866025403784439,1.,0.866025403784439,1.,0.866025403784439,1.,0.866025403784439,
1.,0.866025403784439,1.,0.866025403784439,1.,0.866025403784439,1.,0.866025403784439,
1.,0.866025403784439,1.,0.866025403784439,1.,0.866025403784439,1.,0.866025403784439,
1.,0.866025403784439,1.,0.866025403784439,1.,0.866025403784439,1.,0.866025403784439,
1.,0.866025403784439,1.,0.866025403784439,1.,0.866025403784439,1.,0.866025403784439,
1.,0.866025403784439,1.,0.866025403784439,1.,0.866025403784439,1.,0.866025403784439,
1.,0.866025403784439,1.,0.866025403784439,1.,0.866025403784439,1.,0.866025403784439,
1.,0.866025403784439,1.,0.866025403784439,1.,0.866025403784439,1.,0.866025403784439,
1.,0.866025403784439,1.,0.866025403784439,1.,0.866025403784439,1.,0.866025403784439,
1.,0.866025403784439,1.,0.866025403784439,1.,0.866025403784439,1.,0.866025403784439,
1.,0.866025403784439,1.,0.866025403784439,1.,0.866025403784439,1.,0.866025403784439,
1.,0.866025403784439,1.,0.866025403784439,1.,0.866025403784439,1.,0.866025403784439,
1.,0.866025403784439,1.,0.866025403784439,1.,0.866025403784439,1.,0.866025403784439,
1.,0.866025403784439,1.,0.866025403784439,1.,0.866025403784439,1.,0.866025403784439,
1.,0.866025403784439,1.,0.866025403784439,1.,0.866025403784439,1.,0.866025403784439,
1.,0.866025403784439,1.,0.866025403784439,1.,0.866025403784439,1.,0.866025403784439,
1.,0.866025403784439,1.,0.866025403784439,1.,0.866025403784439,1.,0.866025403784439,
1.,0.866025403784439,1.,0.866025403784439,1.,0.866025403784439,1.,0.866025403784439,
1.,0.866025403784439,1.,0.866025403784439,1.,0.866025403784439,1.,0.866025403784439,
1.,0.866025403784439,1.,0.866025403784439,1.,0.866025403784439,1.,0.866025403784439,
1.,0.866025403784439,1.,0.866025403784439,1.,0.866025403784439,1.,0.866025403784439,
1.,0.866025403784439,1.,0.866025403784439,1.,0.866025403784439,1.,0.866025403784439,
1.,0.866025403784439,1.,0.866025403784439,1.,0.866025403784439,1.,0.866025403784439,
1.,0.866025403784439,1.,0.866025403784439,1.,0.866025403784439,1.,0.866025403784439,
1.,0.866025403784439,1.,0.866025403784439,1.,0.866025403784439,1.,0.866025403784439,
1.,0.866025403784439,1.,0.866025403784439,1.,0.866025403784439,1.,0.866025403784439,
1.,0.866025403784439,1.,0.866025403784439,1.,0.866025403784439,1.,0.866025403784439,
1.,0.866025403784439,1.,0.866025403784439,1.,0.866025403784439,1.,0.866025403784439,
1.,0.866025403784439,1.,0.866025403784439,1.,0.866025403784439,1.,0.866025403784439,
1.,0.866025403784439,1.,0.866025403784439,1.,0.866025403784439,1.,0.866025403784439,
1.,0.866025403784439,1.,0.866025403784439,1.,0.866025403784439,1.,0.866025403784439,
1.,0.866025403784439,1.,0.866025403784439,1.,0.866025403784439,1.,0.866025403784439,
1.,0.866025403784439,1.,0.866025403784439,1.,0.866025403784439,1.,0.866025403784439,
1.),(1.,0.866025403784439,1.,0.866025403784439,1.,0.866025403784439,1.,
0.866025403784439,1.,0.866025403784439,1.,0.866025403784439,1.,0.866025403784439,
1.,0.866025403784439,1.,0.866025403784439,1.,0.866025403784439,1.,0.866025403784439,
1.,0.866025403784439,1.,0.866025403784439,1.,0.866025403784439,1.,0.866025403784439,
1.,0.866025403784439,1.,0.866025403784439,1.,0.866025403784439,1.,0.866025403784439,
1.,0.866025403784439,1.,0.866025403784439,1.,0.866025403784439,1.,0.866025403784439,
1.,0.866025403784439,1.,0.866025403784439,1.,0.866025403784439,1.,0.866025403784439,
1.,0.866025403784439,1.,0.866025403784439,1.,0.866025403784439,1.,0.866025403784439,
1.,0.866025403784439,1.,0.866025403784439,1.,0.866025403784439,1.,0.866025403784439,
1.,0.866025403784439,1.,0.866025403784439,1.,0.866025403784439,1.,0.866025403784439,
1.,0.866025403784439,1.,0.866025403784439,1.,0.866025403784439,1.,0.866025403784439,
1.,0.866025403784439,1.,0.866025403784439,1.,0.866025403784439,1.,0.866025403784439,
1.,0.866025403784439,1.,0.866025403784439,1.,0.866025403784439,1.,0.866025403784439,
1.,0.866025403784439,1.,0.866025403784439,1.,0.866025403784439,1.,0.866025403784439,
1.,0.866025403784439,1.,0.866025403784439,1.,0.866025403784439,1.,0.866025403784439,
1.,0.866025403784439,1.,0.866025403784439,1.,0.866025403784439,1.,0.866025403784439,
1.,0.866025403784439,1.,0.866025403784439,1.,0.866025403784439,1.,0.866025403784439,
1.,0.866025403784439,1.,0.866025403784439,1.,0.866025403784439,1.,0.866025403784439,
1.,0.866025403784439,1.,0.866025403784439,1.,0.866025403784439,1.,0.866025403784439,
1.,0.866025403784439,1.,0.866025403784439,1.,0.866025403784439,1.,0.866025403784439,
1.,0.866025403784439,1.,0.866025403784439,1.,0.866025403784439,1.,0.866025403784439,
1.,0.866025403784439,1.,0.866025403784439,1.,0.866025403784439,1.,0.866025403784439,
1.,0.866025403784439,1.,0.866025403784439,1.,0.866025403784439,1.,0.866025403784439,
1.,0.866025403784439,1.,0.866025403784439,1.,0.866025403784439,1.,0.866025403784439,
1.,0.866025403784439,1.,0.866025403784439,1.,0.866025403784439,1.,0.866025403784439,
1.,0.866025403784439,1.,0.866025403784439,1.,0.866025403784439,1.,0.866025403784439,
1.,0.866025403784439,1.,0.866025403784439,1.,0.866025403784439,1.,0.866025403784439,
1.,0.866025403784439,1.,0.866025403784439,1.,0.866025403784439,1.,0.866025403784439,
1.,0.866025403784439,1.,0.866025403784439,1.,0.866025403784439,1.,0.866025403784439,
1.,0.866025403784439,1.,0.866025403784439,1.,0.866025403784439,1.,0.866025403784439,
1.,0.866025403784439,1.,0.866025403784439,1.,0.866025403784439,1.,0.866025403784439,
1.,0.866025403784439,1.,0.866025403784439,1.,0.866025403784439,1.,0.866025403784439,
1.,0.866025403784439,1.,0.866025403784439,1.,0.866025403784439,1.,0.866025403784439,
1.,0.866025403784439,1.,0.866025403784439,1.,0.866025403784439,1.,0.866025403784439,
1.,0.866025403784439,1.,0.866025403784439,1.,0.866025403784439,1.,0.866025403784439,
1.,0.866025403784439,1.,0.866025403784439,1.,0.866025403784439,1.,0.866025403784439,
1.,0.866025403784439,1.,0.866025403784439,1.,0.866025403784439,1.,0.866025403784439,
1.,0.866025403784439,1.,0.866025403784439,1.,0.866025403784439,1.,0.866025403784439,
1.,0.866025403784439,1.,0.866025403784439,1.,0.866025403784439,1.,0.866025403784439,
1.,0.866025403784439,1.,0.866025403784439,1.,0.866025403784439,1.,0.866025403784439,
1.,0.866025403784439,1.,0.866025403784439,1.,0.866025403784439,1.,0.866025403784439,
1.,0.866025403784439,1.,0.866025403784439,1.,0.866025403784439,1.,0.866025403784439,
1.,0.866025403784439,1.,0.866025403784439,1.,0.866025403784439,1.,0.866025403784439,
1.,0.866025403784439,1.,0.866025403784439,1.,0.866025403784439,1.,0.866025403784439,
1.,0.866025403784439,1.,0.866025403784439,1.,0.866025403784439,1.,0.866025403784439,
1.,0.866025403784439,1.,0.866025403784439,1.,0.866025403784439,1.,0.866025403784439,
1.,0.866025403784439,1.,0.866025403784439,1.,0.866025403784439,1.,0.866025403784439,
1.,0.866025403784439,1.,0.866025403784439,1.,0.866025403784439,1.,0.866025403784439,
1.,0.866025403784439,1.,0.866025403784439,1.,0.866025403784439,1.,0.866025403784439,
1.,0.866025403784439,1.,0.866025403784439,1.,0.866025403784439,1.,0.866025403784439,
1.,0.866025403784439,1.,0.866025403784439,1.,0.866025403784439,1.,0.866025403784439,
1.,0.866025403784439,1.,0.866025403784439,1.,0.866025403784439,1.,0.866025403784439,
1.,0.866025403784439,1.,0.866025403784439,1.,0.866025403784439,1.,0.866025403784439,
1.,0.866025403784439,1.,0.866025403784439,1.,0.866025403784439,1.,0.866025403784439,
1.,0.866025403784439,1.,0.866025403784439,1.,0.866025403784439,1.,0.866025403784439,
1.,0.866025403784439,1.,0.866025403784439,1.,0.866025403784439,1.,0.866025403784439,
1.,0.866025403784439,1.,0.866025403784439,1.,0.866025403784439,1.,0.866025403784439,
1.,0.866025403784439,1.,0.866025403784439,1.,0.866025403784439,1.,0.866025403784439,
1.,0.866025403784439,1.,0.866025403784439,1.,0.866025403784439,1.,0.866025403784439,
1.,0.866025403784439,1.,0.866025403784439,1.,0.866025403784439,1.,0.866025403784439,
1.,0.866025403784439,1.,0.866025403784439,1.,0.866025403784439,1.,0.866025403784439,
1.,0.866025403784439,1.,0.866025403784439,1.,0.866025403784439,1.,0.866025403784439,
1.,0.866025403784439,1.,0.866025403784439,1.,0.866025403784439,1.,0.866025403784439,
1.,0.866025403784439,1.,0.866025403784439,1.,0.866025403784439,1.,0.866025403784439,
1.,0.866025403784439,1.,0.866025403784439,1.,0.866025403784439,1.,0.866025403784439,
1.,0.866025403784439,1.,0.866025403784439,1.,0.866025403784439,1.,0.866025403784439,
1.,0.866025403784439,1.,0.866025403784439,1.,0.866025403784439,1.,0.866025403784439,
1.,0.866025403784439,1.,0.866025403784439,1.,0.866025403784439,1.,0.866025403784439,
1.,0.866025403784439,1.,0.866025403784439,1.,0.866025403784439,1.,0.866025403784439,
1.,0.866025403784439,1.,0.866025403784439,1.,0.866025403784439,1.,0.866025403784439,
1.,0.866025403784439,1.,0.866025403784439,1.,0.866025403784439,1.,0.866025403784439,
1.,0.866025403784439,1.,0.866025403784439,1.,0.866025403784439,1.,0.866025403784439,
1.,0.866025403784439,1.,0.866025403784439,1.,0.866025403784439,1.,0.866025403784439,
1.,0.866025403784439,1.,0.866025403784439,1.,0.866025403784439,1.,0.866025403784439,
1.,0.866025403784439,1.,0.866025403784439,1.,0.866025403784439,1.,0.866025403784439,
1.,0.866025403784439,1.,0.866025403784439,1.,0.866025403784439,1.,0.866025403784439,
1.,0.866025403784439,1.,0.866025403784439,1.,0.866025403784439,1.,0.866025403784439,
1.,0.866025403784439,1.,0.866025403784439,1.,0.866025403784439,1.,0.866025403784439,
1.,0.866025403784439,1.,0.866025403784439,1.,0.866025403784439,1.,0.866025403784439,
1.,0.866025403784439,1.,0.866025403784439,1.,0.866025403784439,1.,0.866025403784439,
1.,0.866025403784439,1.,0.866025403784439,1.,0.866025403784439,1.,0.866025403784439,
1.,0.866025403784439,1.,0.866025403784439,1.,0.866025403784439,1.,0.866025403784439,
1.,0.866025403784439,1.,0.866025403784439,1.,0.866025403784439,1.,0.866025403784439,
1.,0.866025403784439,1.,0.866025403784439,1.,0.866025403784439,1.,0.866025403784439,
1.,0.866025403784439,1.,0.866025403784439,1.,0.866025403784439,1.,0.866025403784439,
1.,0.866025403784439,1.,0.866025403784439,1.,0.866025403784439,1.,0.866025403784439,
1.,0.866025403784439,1.,0.866025403784439,1.,0.866025403784439,1.,0.866025403784439,
1.,0.866025403784439,1.,0.866025403784439,1.,0.866025403784439,1.,0.866025403784439,
1.,0.866025403784439,1.,0.866025403784439,1.,0.866025403784439,1.,0.866025403784439,
1.,0.866025403784439,1.,0.866025403784439,1.,0.866025403784439,1.,0.866025403784439,
1.,0.866025403784439,1.,0.866025403784439,1.,0.866025403784439,1.,0.866025403784439,
1.,0.866025403784439,1.,0.866025403784439,1.,0.866025403784439,1.,0.866025403784439,
1.,0.866025403784439,1.,0.866025403784439,1.,0.866025403784439,1.,0.866025403784439,
1.,0.866025403784439,1.,0.866025403784439,1.,0.866025403784439,1.,0.866025403784439,
1.,0.866025403784439,1.,0.866025403784439,1.,0.866025403784439,1.,0.866025403784439,
1.,0.866025403784439,1.,0.866025403784439,1.,0.866025403784439,1.,0.866025403784439,
1.,0.866025403784439,1.,0.866025403784439,1.,0.866025403784439,1.,0.866025403784439,
1.,0.866025403784439,1.,0.866025403784439,1.,0.866025403784439,1.,0.866025403784439,
1.,0.866025403784439,1.,0.866025403784439,1.,0.866025403784439,1.,0.866025403784439,
1.,0.866025403784439,1.,0.866025403784439,1.,0.866025403784439,1.,0.866025403784439,
1.,0.866025403784439,1.,0.866025403784439,1.,0.866025403784439,1.,0.866025403784439,
1.,0.866025403784439,1.,0.866025403784439,1.,0.866025403784439,1.,0.866025403784439,
1.,0.866025403784439,1.,0.866025403784439,1.,0.866025403784439,1.,0.866025403784439,
1.,0.866025403784439,1.,0.866025403784439,1.,0.866025403784439,1.,0.866025403784439,
1.,0.866025403784439,1.,0.866025403784439,1.,0.866025403784439,1.,0.866025403784439,
1.,0.866025403784439,1.,0.866025403784439,1.,0.866025403784439,1.,0.866025403784439,
1.,0.866025403784439,1.,0.866025403784439,1.,0.866025403784439,1.,0.866025403784439,
1.,0.866025403784439,1.,0.866025403784439,1.,0.866025403784439,1.,0.866025403784439,
1.,0.866025403784439,1.,0.866025403784439,1.,0.866025403784439,1.,0.866025403784439,
1.,0.866025403784439,1.,0.866025403784439,1.,0.866025403784439,1.,0.866025403784439,
1.,0.866025403784439,1.,0.866025403784439,1.,0.866025403784439,1.,0.866025403784439,
1.,0.866025403784439,1.,0.866025403784439,1.,0.866025403784439,1.,0.866025403784439,
1.,0.866025403784439,1.,0.866025403784439,1.,0.866025403784439,1.,0.866025403784439,
1.,0.866025403784439,1.,0.866025403784439,1.,0.866025403784439,1.,0.866025403784439,
1.,0.866025403784439,1.,0.866025403784439,1.,0.866025403784439,1.,0.866025403784439,
1.,0.866025403784439,1.,0.866025403784439,1.,0.866025403784439,1.,0.866025403784439,
1.,0.866025403784439,1.,0.866025403784439,1.,0.866025403784439,1.,0.866025403784439,
1.,0.866025403784439,1.,0.866025403784439,1.,0.866025403784439,1.,0.866025403784439,
1.,0.866025403784439,1.,0.866025403784439,1.,0.866025403784439,1.,0.866025403784439,
1.,0.866025403784439,1.,0.866025403784439,1.,0.866025403784439,1.,0.866025403784439,
1.,0.866025403784439,1.,0.866025403784439,1.,0.866025403784439,1.,0.866025403784439,
1.,0.866025403784439,1.,0.866025403784439,1.,0.866025403784439,1.)))
REPRESENTATION_ITEM('')
SURFACE()
);
#181=(
BOUNDED_SURFACE()
B_SPLINE_SURFACE(3,2,((#39526,#39527,#39528),(#39529,#39530,#39531),(#39532,
#39533,#39534),(#39535,#39536,#39537),(#39538,#39539,#39540),(#39541,#39542,
#39543),(#39544,#39545,#39546),(#39547,#39548,#39549),(#39550,#39551,#39552),
(#39553,#39554,#39555),(#39556,#39557,#39558),(#39559,#39560,#39561),(#39562,
#39563,#39564),(#39565,#39566,#39567),(#39568,#39569,#39570),(#39571,#39572,
#39573),(#39574,#39575,#39576),(#39577,#39578,#39579),(#39580,#39581,#39582),
(#39583,#39584,#39585),(#39586,#39587,#39588),(#39589,#39590,#39591),(#39592,
#39593,#39594),(#39595,#39596,#39597),(#39598,#39599,#39600),(#39601,#39602,
#39603),(#39604,#39605,#39606),(#39607,#39608,#39609),(#39610,#39611,#39612),
(#39613,#39614,#39615),(#39616,#39617,#39618),(#39619,#39620,#39621),(#39622,
#39623,#39624),(#39625,#39626,#39627),(#39628,#39629,#39630),(#39631,#39632,
#39633),(#39634,#39635,#39636),(#39637,#39638,#39639),(#39640,#39641,#39642),
(#39643,#39644,#39645),(#39646,#39647,#39648),(#39649,#39650,#39651)),
 .UNSPECIFIED.,.F.,.F.,.F.)
B_SPLINE_SURFACE_WITH_KNOTS((4,2,2,2,2,2,2,2,2,2,2,2,2,2,2,2,2,2,2,2,4),
(3,3),(0.0174298903432871,0.0185192584897425,0.019608626636198,0.0206979947826534,
0.0217873629291089,0.0223320470023366,0.0228767310755643,0.0239660992220198,
0.0250554673684752,0.025600151441703,0.0261448355149307,0.0272342036613861,
0.0277788877346139,0.0283235718078416,0.029412939954297,0.0305023081007525,
0.0315916762472079,0.0326810443936634,0.0332257284668911,0.0337704125401188,
0.0348597806865743),(0.,1.),.UNSPECIFIED.)
GEOMETRIC_REPRESENTATION_ITEM()
RATIONAL_B_SPLINE_SURFACE(((1.,0.706866009891761,1.),(1.,0.707709971120244,
1.),(1.,0.706378287598767,1.),(1.,0.699609550425451,1.),(1.,0.694251408628478,
1.),(1.,0.680153613237048,1.),(1.,0.671289168508122,1.),(1.,0.651466158778394,
1.),(1.,0.64048617306175,1.),(1.,0.623110795499309,1.),(1.,0.617152560263192,
1.),(1.,0.605316890643934,1.),(1.,0.599412164382846,1.),(1.,0.581980631318285,
1.),(1.,0.570694981696628,1.),(1.,0.550546690048529,1.),(1.,0.542015457727399,
1.),(1.,0.532586496259878,1.),(1.,0.530005387777312,1.),(1.,0.526142825846638,
1.),(1.,0.524867626920824,1.),(1.,0.523238184105568,1.),(1.,0.525025712186939,
1.),(1.,0.531687007265021,1.),(1.,0.534590177846375,1.),(1.,0.541481193611421,
1.),(1.,0.545459204735857,1.),(1.,0.558669094849934,1.),(1.,0.569250982154013,
1.),(1.,0.591912604715541,1.),(1.,0.603810048297302,1.),(1.,0.627370297955306,
1.),(1.,0.639116797025499,1.),(1.,0.660432022552727,1.),(1.,0.670115428840362,
1.),(1.,0.682559312106454,1.),(1.,0.686375173907005,1.),(1.,0.693053327636874,
1.),(1.,0.695935943959762,1.),(1.,0.703157954701394,1.),(1.,0.706075946662903,
1.),(1.,0.706882331541542,1.)))
REPRESENTATION_ITEM('')
SURFACE()
);
#182=(
BOUNDED_SURFACE()
B_SPLINE_SURFACE(3,2,((#39652,#39653,#39654),(#39655,#39656,#39657),(#39658,
#39659,#39660),(#39661,#39662,#39663),(#39664,#39665,#39666),(#39667,#39668,
#39669),(#39670,#39671,#39672),(#39673,#39674,#39675),(#39676,#39677,#39678),
(#39679,#39680,#39681),(#39682,#39683,#39684),(#39685,#39686,#39687),(#39688,
#39689,#39690),(#39691,#39692,#39693),(#39694,#39695,#39696),(#39697,#39698,
#39699),(#39700,#39701,#39702),(#39703,#39704,#39705),(#39706,#39707,#39708),
(#39709,#39710,#39711),(#39712,#39713,#39714),(#39715,#39716,#39717),(#39718,
#39719,#39720),(#39721,#39722,#39723),(#39724,#39725,#39726),(#39727,#39728,
#39729),(#39730,#39731,#39732),(#39733,#39734,#39735),(#39736,#39737,#39738),
(#39739,#39740,#39741),(#39742,#39743,#39744),(#39745,#39746,#39747),(#39748,
#39749,#39750),(#39751,#39752,#39753),(#39754,#39755,#39756),(#39757,#39758,
#39759),(#39760,#39761,#39762),(#39763,#39764,#39765),(#39766,#39767,#39768),
(#39769,#39770,#39771),(#39772,#39773,#39774),(#39775,#39776,#39777),(#39778,
#39779,#39780),(#39781,#39782,#39783)),.UNSPECIFIED.,.F.,.F.,.F.)
B_SPLINE_SURFACE_WITH_KNOTS((4,2,2,2,2,2,2,2,2,2,2,2,2,2,2,2,2,2,2,2,2,
4),(3,3),(0.0174355915143997,0.0185253159840497,0.0196150404536998,0.0207047649233498,
0.0217944893929999,0.0223393516278249,0.0228842138626499,0.0239739383323,
0.02506366280195,0.0256085250367751,0.0261533872716001,0.0272431117412501,
0.0277879739760752,0.0283328362109002,0.0288776984457252,0.0294225606805503,
0.0305122851502003,0.0316020096198504,0.0326917340895004,0.0332365963243254,
0.0337814585591505,0.0348711830288005),(0.,1.),.UNSPECIFIED.)
GEOMETRIC_REPRESENTATION_ITEM()
RATIONAL_B_SPLINE_SURFACE(((1.,0.524035202708704,1.),(1.,0.52369296431929,
1.),(1.,0.526394142477004,1.),(1.,0.536829948771709,1.),(1.,0.544467574436789,
1.),(1.,0.563002631288668,1.),(1.,0.574012202433206,1.),(1.,0.596893654025968,
1.),(1.,0.608827575768556,1.),(1.,0.626487538313077,1.),(1.,0.632339905306929,
1.),(1.,0.643592429688047,1.),(1.,0.649024086836218,1.),(1.,0.664570352465133,
1.),(1.,0.673967207524643,1.),(1.,0.689780774219124,1.),(1.,0.695966905675102,
1.),(1.,0.702388249318966,1.),(1.,0.704051452628861,1.),(1.,0.706358678483347,
1.),(1.,0.706995125392999,1.),(1.,0.707289148463133,1.),(1.,0.705381051410457,
1.),(1.,0.699485171860676,1.),(1.,0.696993043119987,1.),(1.,0.69112912697355,
1.),(1.,0.687757727348698,1.),(1.,0.680223099202971,1.),(1.,0.676059589951543,
1.),(1.,0.667018043806083,1.),(1.,0.662112134338359,1.),(1.,0.646674940339596,
1.),(1.,0.635448505441412,1.),(1.,0.612137111297426,1.),(1.,0.599953887245996,
1.),(1.,0.576916856514265,1.),(1.,0.565959879293194,1.),(1.,0.551559273150467,
1.),(1.,0.547084490609781,1.),(1.,0.539237982614899,1.),(1.,0.53584249288952,
1.),(1.,0.527460168857136,1.),(1.,0.524283085212896,1.),(1.,0.524030615668023,
1.)))
REPRESENTATION_ITEM('')
SURFACE()
);
#198=(
BOUNDED_CURVE()
B_SPLINE_CURVE(2,(#28081,#28082,#28083),.UNSPECIFIED.,.F.,.F.)
B_SPLINE_CURVE_WITH_KNOTS((3,3),(-2.2693844624543,-1.90898280074518),
 .UNSPECIFIED.)
CURVE()
GEOMETRIC_REPRESENTATION_ITEM()
RATIONAL_B_SPLINE_CURVE((1.7477494971405,1.72129587968328,1.68438569901946))
REPRESENTATION_ITEM('')
);
#199=(
BOUNDED_CURVE()
B_SPLINE_CURVE(2,(#28084,#28085,#28086),.UNSPECIFIED.,.F.,.F.)
B_SPLINE_CURVE_WITH_KNOTS((3,3),(1.90898280074519,2.2693844624543),
 .UNSPECIFIED.)
CURVE()
GEOMETRIC_REPRESENTATION_ITEM()
RATIONAL_B_SPLINE_CURVE((1.68438569901946,1.72129587968328,1.7477494971405))
REPRESENTATION_ITEM('')
);
#200=(
BOUNDED_CURVE()
B_SPLINE_CURVE(2,(#30719,#30720,#30721,#30722,#30723,#30724,#30725,#30726,
#30727,#30728,#30729,#30730,#30731,#30732,#30733,#30734,#30735,#30736,#30737,
#30738,#30739,#30740,#30741,#30742,#30743,#30744,#30745,#30746,#30747,#30748,
#30749,#30750,#30751,#30752,#30753,#30754,#30755,#30756,#30757,#30758,#30759,
#30760,#30761,#30762,#30763,#30764,#30765,#30766,#30767,#30768,#30769,#30770,
#30771,#30772,#30773,#30774,#30775,#30776,#30777,#30778,#30779,#30780,#30781,
#30782,#30783,#30784,#30785,#30786,#30787,#30788,#30789,#30790,#30791,#30792,
#30793,#30794,#30795,#30796,#30797,#30798,#30799,#30800,#30801,#30802,#30803,
#30804,#30805,#30806,#30807,#30808,#30809,#30810,#30811,#30812,#30813,#30814,
#30815,#30816,#30817,#30818,#30819,#30820,#30821,#30822,#30823,#30824,#30825,
#30826,#30827,#30828,#30829,#30830,#30831,#30832,#30833,#30834,#30835,#30836,
#30837,#30838,#30839,#30840,#30841,#30842,#30843,#30844,#30845,#30846,#30847,
#30848,#30849,#30850,#30851,#30852,#30853,#30854,#30855,#30856,#30857,#30858,
#30859,#30860,#30861,#30862,#30863,#30864,#30865,#30866,#30867,#30868,#30869,
#30870,#30871,#30872,#30873,#30874,#30875,#30876,#30877,#30878,#30879,#30880,
#30881,#30882,#30883,#30884,#30885,#30886,#30887,#30888,#30889,#30890,#30891,
#30892,#30893,#30894,#30895,#30896,#30897,#30898,#30899,#30900,#30901,#30902,
#30903,#30904,#30905,#30906,#30907,#30908,#30909,#30910,#30911,#30912,#30913,
#30914,#30915,#30916,#30917,#30918,#30919,#30920,#30921,#30922,#30923,#30924,
#30925,#30926,#30927,#30928,#30929,#30930,#30931,#30932,#30933,#30934,#30935,
#30936,#30937,#30938,#30939,#30940,#30941,#30942,#30943,#30944,#30945,#30946,
#30947,#30948,#30949,#30950,#30951,#30952,#30953,#30954,#30955,#30956,#30957,
#30958,#30959,#30960,#30961,#30962,#30963,#30964,#30965,#30966,#30967,#30968,
#30969,#30970,#30971,#30972,#30973,#30974,#30975,#30976,#30977,#30978,#30979,
#30980,#30981,#30982,#30983,#30984,#30985,#30986,#30987,#30988,#30989,#30990,
#30991,#30992,#30993,#30994,#30995,#30996,#30997,#30998,#30999,#31000,#31001,
#31002,#31003,#31004,#31005,#31006,#31007,#31008,#31009,#31010,#31011,#31012,
#31013,#31014,#31015,#31016,#31017,#31018,#31019,#31020,#31021,#31022,#31023,
#31024,#31025,#31026,#31027,#31028,#31029,#31030,#31031,#31032,#31033,#31034,
#31035,#31036,#31037,#31038,#31039,#31040,#31041,#31042,#31043,#31044,#31045,
#31046,#31047,#31048,#31049,#31050,#31051,#31052,#31053,#31054,#31055,#31056,
#31057,#31058,#31059,#31060,#31061,#31062,#31063,#31064,#31065,#31066,#31067,
#31068,#31069,#31070,#31071,#31072,#31073,#31074,#31075,#31076,#31077,#31078,
#31079,#31080,#31081,#31082,#31083,#31084,#31085,#31086,#31087,#31088,#31089,
#31090,#31091,#31092,#31093,#31094,#31095,#31096,#31097,#31098,#31099,#31100,
#31101,#31102,#31103,#31104,#31105,#31106,#31107,#31108,#31109,#31110,#31111,
#31112,#31113,#31114,#31115,#31116,#31117,#31118,#31119,#31120,#31121,#31122,
#31123,#31124,#31125,#31126,#31127,#31128,#31129,#31130,#31131,#31132,#31133,
#31134,#31135,#31136,#31137,#31138,#31139,#31140,#31141,#31142,#31143,#31144,
#31145,#31146,#31147,#31148,#31149,#31150,#31151,#31152,#31153,#31154,#31155,
#31156,#31157,#31158,#31159,#31160,#31161,#31162,#31163,#31164,#31165,#31166,
#31167,#31168,#31169,#31170,#31171,#31172,#31173,#31174,#31175,#31176,#31177,
#31178,#31179,#31180,#31181,#31182,#31183,#31184,#31185,#31186,#31187,#31188,
#31189,#31190,#31191,#31192,#31193,#31194,#31195,#31196,#31197,#31198,#31199,
#31200,#31201,#31202,#31203,#31204,#31205,#31206,#31207,#31208,#31209,#31210,
#31211,#31212,#31213,#31214,#31215,#31216,#31217,#31218,#31219,#31220,#31221,
#31222,#31223,#31224,#31225,#31226,#31227,#31228,#31229,#31230,#31231,#31232,
#31233,#31234,#31235,#31236,#31237,#31238,#31239,#31240,#31241,#31242,#31243,
#31244,#31245,#31246,#31247,#31248,#31249,#31250,#31251,#31252,#31253,#31254,
#31255,#31256,#31257,#31258,#31259,#31260,#31261,#31262,#31263,#31264,#31265,
#31266,#31267,#31268,#31269,#31270,#31271,#31272,#31273,#31274,#31275,#31276,
#31277,#31278,#31279,#31280,#31281,#31282,#31283,#31284,#31285,#31286,#31287,
#31288,#31289,#31290,#31291,#31292,#31293,#31294,#31295,#31296,#31297,#31298,
#31299,#31300,#31301,#31302,#31303,#31304,#31305,#31306,#31307,#31308,#31309,
#31310,#31311,#31312,#31313,#31314,#31315,#31316,#31317,#31318,#31319,#31320,
#31321,#31322,#31323,#31324,#31325,#31326,#31327,#31328,#31329,#31330,#31331,
#31332,#31333,#31334,#31335,#31336,#31337,#31338,#31339,#31340,#31341,#31342,
#31343,#31344,#31345,#31346,#31347,#31348,#31349,#31350,#31351,#31352,#31353,
#31354,#31355,#31356,#31357,#31358,#31359,#31360,#31361,#31362,#31363,#31364,
#31365,#31366,#31367,#31368,#31369,#31370,#31371,#31372,#31373,#31374,#31375,
#31376,#31377,#31378,#31379,#31380,#31381,#31382,#31383,#31384,#31385,#31386,
#31387,#31388,#31389,#31390,#31391,#31392,#31393,#31394,#31395,#31396,#31397,
#31398,#31399,#31400,#31401,#31402,#31403,#31404,#31405,#31406,#31407,#31408,
#31409,#31410,#31411,#31412,#31413,#31414,#31415,#31416,#31417,#31418,#31419,
#31420,#31421,#31422,#31423,#31424,#31425,#31426,#31427,#31428,#31429,#31430,
#31431,#31432,#31433,#31434,#31435,#31436,#31437,#31438,#31439,#31440,#31441,
#31442,#31443,#31444,#31445,#31446,#31447,#31448,#31449,#31450,#31451,#31452,
#31453,#31454,#31455,#31456,#31457,#31458,#31459,#31460,#31461,#31462,#31463,
#31464,#31465,#31466,#31467,#31468,#31469,#31470,#31471,#31472,#31473,#31474,
#31475,#31476,#31477,#31478,#31479,#31480,#31481,#31482,#31483,#31484,#31485,
#31486,#31487,#31488,#31489,#31490,#31491,#31492,#31493,#31494,#31495,#31496,
#31497,#31498,#31499,#31500,#31501,#31502,#31503,#31504,#31505,#31506,#31507,
#31508,#31509,#31510,#31511,#31512,#31513,#31514,#31515,#31516,#31517,#31518,
#31519,#31520,#31521,#31522,#31523,#31524,#31525,#31526,#31527,#31528,#31529,
#31530,#31531,#31532,#31533,#31534,#31535,#31536,#31537,#31538,#31539,#31540,
#31541,#31542,#31543,#31544,#31545,#31546,#31547,#31548,#31549,#31550,#31551,
#31552,#31553,#31554,#31555,#31556,#31557,#31558,#31559,#31560,#31561,#31562,
#31563,#31564,#31565,#31566,#31567,#31568,#31569,#31570,#31571,#31572,#31573,
#31574,#31575,#31576,#31577,#31578,#31579,#31580,#31581,#31582,#31583,#31584,
#31585,#31586,#31587,#31588,#31589,#31590,#31591,#31592,#31593,#31594,#31595,
#31596,#31597,#31598,#31599,#31600,#31601,#31602,#31603,#31604,#31605,#31606,
#31607,#31608,#31609,#31610,#31611,#31612,#31613,#31614,#31615,#31616,#31617,
#31618,#31619,#31620,#31621,#31622,#31623,#31624,#31625,#31626,#31627,#31628,
#31629,#31630,#31631,#31632,#31633,#31634,#31635,#31636,#31637,#31638,#31639,
#31640,#31641,#31642,#31643,#31644,#31645,#31646,#31647,#31648,#31649,#31650,
#31651,#31652,#31653,#31654,#31655,#31656,#31657,#31658,#31659,#31660,#31661,
#31662,#31663,#31664,#31665),.UNSPECIFIED.,.F.,.F.)
B_SPLINE_CURVE_WITH_KNOTS((3,2,2,2,2,2,2,2,2,2,2,2,2,2,2,2,2,2,2,2,2,2,
2,2,2,2,2,2,2,2,2,2,2,2,2,2,2,2,2,2,2,2,2,2,2,2,2,2,2,2,2,2,2,2,2,2,2,2,
2,2,2,2,2,2,2,2,2,2,2,2,2,2,2,2,2,2,2,2,2,2,2,2,2,2,2,2,2,2,2,2,2,2,2,2,
2,2,2,2,2,2,2,2,2,2,2,2,2,2,2,2,2,2,2,2,2,2,2,2,2,2,2,2,2,2,2,2,2,2,2,2,
2,2,2,2,2,2,2,2,2,2,2,2,2,2,2,2,2,2,2,2,2,2,2,2,2,2,2,2,2,2,2,2,2,2,2,2,
2,2,2,2,2,2,2,2,2,2,2,2,2,2,2,2,2,2,2,2,2,2,2,2,2,2,2,2,2,2,2,2,2,2,2,2,
2,2,2,2,2,2,2,2,2,2,2,2,2,2,2,2,2,2,2,2,2,2,2,2,2,2,2,2,2,2,2,2,2,2,2,2,
2,2,2,2,2,2,2,2,2,2,2,2,2,2,2,2,2,2,2,2,2,2,2,2,2,2,2,2,2,2,2,2,2,2,2,2,
2,2,2,2,2,2,2,2,2,2,2,2,2,2,2,2,2,2,2,2,2,2,2,2,2,2,2,2,2,2,2,2,2,2,2,2,
2,2,2,2,2,2,2,2,2,2,2,2,2,2,2,2,2,2,2,2,2,2,2,2,2,2,2,2,2,2,2,2,2,2,2,2,
2,2,2,2,2,2,2,2,2,2,2,2,2,2,2,2,2,2,2,2,2,2,2,2,2,2,2,2,2,2,2,2,2,2,2,2,
2,2,2,2,2,2,2,2,2,2,2,2,2,2,2,2,2,2,2,2,2,2,2,2,2,2,2,2,2,2,2,2,2,2,2,2,
2,2,2,2,2,2,2,2,2,2,2,2,2,2,2,2,2,2,2,2,2,2,2,2,2,2,2,2,2,2,2,2,2,2,2,2,
2,2,2,2,2,2,2,2,2,2,2,2,2,2,2,2,2,2,2,3),(0.00769788512143581,0.00823045267489712,
0.0102880658436214,0.0123456790123457,0.01440329218107,0.0164609053497942,
0.0185185185185185,0.0205761316872428,0.0226337448559671,0.0246913580246914,
0.0267489711934156,0.0288065843621399,0.0308641975308642,0.0329218106995885,
0.0349794238683128,0.037037037037037,0.0390946502057613,0.0411522633744856,
0.0432098765432099,0.0452674897119342,0.0473251028806584,0.0493827160493827,
0.051440329218107,0.0534979423868313,0.0555555555555556,0.0576131687242798,
0.0596707818930041,0.0617283950617284,0.0637860082304527,0.065843621399177,
0.0679012345679012,0.0699588477366255,0.0720164609053498,0.0740740740740741,
0.0761316872427984,0.0781893004115226,0.0802469135802469,0.0823045267489712,
0.0843621399176955,0.0864197530864197,0.088477366255144,0.0905349794238683,
0.0925925925925926,0.0946502057613169,0.0967078189300412,0.0987654320987654,
0.10082304526749,0.102880658436214,0.104938271604938,0.106995884773663,
0.109053497942387,0.111111111111111,0.113168724279835,0.11522633744856,
0.117283950617284,0.119341563786008,0.121399176954733,0.123456790123457,
0.125514403292181,0.127572016460905,0.12962962962963,0.131687242798354,
0.133744855967078,0.135802469135802,0.137860082304527,0.139917695473251,
0.141975308641975,0.1440329218107,0.146090534979424,0.148148148148148,0.150205761316872,
0.152263374485597,0.154320987654321,0.156378600823045,0.15843621399177,
0.160493827160494,0.162551440329218,0.164609053497942,0.166666666666667,
0.168724279835391,0.170781893004115,0.172839506172839,0.174897119341564,
0.176954732510288,0.179012345679012,0.181069958847737,0.183127572016461,
0.185185185185185,0.18724279835391,0.189300411522634,0.191358024691358,
0.193415637860082,0.195473251028807,0.197530864197531,0.199588477366255,
0.201646090534979,0.203703703703704,0.205761316872428,0.207818930041152,
0.209876543209877,0.211934156378601,0.213991769547325,0.216049382716049,
0.218106995884774,0.220164609053498,0.222222222222222,0.224279835390947,
0.226337448559671,0.228395061728395,0.230452674897119,0.232510288065844,
0.234567901234568,0.236625514403292,0.238683127572016,0.240740740740741,
0.242798353909465,0.244855967078189,0.246913580246914,0.248971193415638,
0.251028806584362,0.253086419753086,0.255144032921811,0.257201646090535,
0.259259259259259,0.261316872427984,0.263374485596708,0.265432098765432,
0.267489711934156,0.269547325102881,0.271604938271605,0.273662551440329,
0.275720164609054,0.277777777777778,0.279835390946502,0.281893004115226,
0.283950617283951,0.286008230452675,0.288065843621399,0.290123456790123,
0.292181069958848,0.294238683127572,0.296296296296296,0.298353909465021,
0.300411522633745,0.302469135802469,0.304526748971193,0.306584362139918,
0.308641975308642,0.310699588477366,0.312757201646091,0.314814814814815,
0.316872427983539,0.318930041152263,0.320987654320988,0.323045267489712,
0.325102880658436,0.327160493827161,0.329218106995885,0.331275720164609,
0.333333333333333,0.335390946502058,0.337448559670782,0.339506172839506,
0.34156378600823,0.343621399176955,0.345679012345679,0.347736625514403,
0.349794238683128,0.351851851851852,0.353909465020576,0.3559670781893,0.358024691358025,
0.360082304526749,0.362139917695473,0.364197530864198,0.366255144032922,
0.368312757201646,0.37037037037037,0.372427983539095,0.374485596707819,
0.376543209876543,0.378600823045267,0.380658436213992,0.382716049382716,
0.38477366255144,0.386831275720165,0.388888888888889,0.390946502057613,
0.393004115226337,0.395061728395062,0.397119341563786,0.39917695473251,
0.401234567901235,0.403292181069959,0.405349794238683,0.407407407407407,
0.409465020576132,0.411522633744856,0.41358024691358,0.415637860082305,
0.417695473251029,0.419753086419753,0.421810699588477,0.423868312757202,
0.425925925925926,0.42798353909465,0.430041152263374,0.432098765432099,
0.434156378600823,0.436213991769547,0.438271604938272,0.440329218106996,
0.44238683127572,0.444444444444444,0.446502057613169,0.448559670781893,
0.450617283950617,0.452674897119342,0.454732510288066,0.45679012345679,
0.458847736625514,0.460905349794239,0.462962962962963,0.465020576131687,
0.467078189300412,0.469135802469136,0.47119341563786,0.473251028806584,
0.475308641975309,0.477366255144033,0.479423868312757,0.481481481481481,
0.483539094650206,0.48559670781893,0.487654320987654,0.489711934156379,
0.491769547325103,0.493827160493827,0.495884773662551,0.497942386831276,
0.5,0.502057613168724,0.504115226337449,0.506172839506173,0.508230452674897,
0.510288065843621,0.512345679012346,0.51440329218107,0.516460905349794,
0.518518518518518,0.520576131687243,0.522633744855967,0.524691358024691,
0.526748971193416,0.52880658436214,0.530864197530864,0.532921810699588,
0.534979423868313,0.537037037037037,0.539094650205761,0.541152263374486,
0.54320987654321,0.545267489711934,0.547325102880658,0.549382716049383,
0.551440329218107,0.553497942386831,0.555555555555556,0.55761316872428,
0.559670781893004,0.561728395061728,0.563786008230453,0.565843621399177,
0.567901234567901,0.569958847736626,0.57201646090535,0.574074074074074,
0.576131687242798,0.578189300411523,0.580246913580247,0.582304526748971,
0.584362139917695,0.58641975308642,0.588477366255144,0.590534979423868,
0.592592592592593,0.594650205761317,0.596707818930041,0.598765432098765,
0.60082304526749,0.602880658436214,0.604938271604938,0.606995884773663,
0.609053497942387,0.611111111111111,0.613168724279835,0.61522633744856,
0.617283950617284,0.619341563786008,0.621399176954732,0.623456790123457,
0.625514403292181,0.627572016460905,0.62962962962963,0.631687242798354,
0.633744855967078,0.635802469135803,0.637860082304527,0.639917695473251,
0.641975308641975,0.6440329218107,0.646090534979424,0.648148148148148,0.650205761316872,
0.652263374485597,0.654320987654321,0.656378600823045,0.65843621399177,
0.660493827160494,0.662551440329218,0.664609053497942,0.666666666666667,
0.668724279835391,0.670781893004115,0.672839506172839,0.674897119341564,
0.676954732510288,0.679012345679012,0.681069958847737,0.683127572016461,
0.685185185185185,0.687242798353909,0.689300411522634,0.691358024691358,
0.693415637860082,0.695473251028807,0.697530864197531,0.699588477366255,
0.70164609053498,0.703703703703704,0.705761316872428,0.707818930041152,
0.709876543209877,0.711934156378601,0.713991769547325,0.716049382716049,
0.718106995884774,0.720164609053498,0.722222222222222,0.724279835390947,
0.726337448559671,0.728395061728395,0.730452674897119,0.732510288065844,
0.734567901234568,0.736625514403292,0.738683127572016,0.740740740740741,
0.742798353909465,0.744855967078189,0.746913580246914,0.748971193415638,
0.751028806584362,0.753086419753086,0.755144032921811,0.757201646090535,
0.759259259259259,0.761316872427984,0.763374485596708,0.765432098765432,
0.767489711934156,0.769547325102881,0.771604938271605,0.773662551440329,
0.775720164609053,0.777777777777778,0.779835390946502,0.781893004115226,
0.783950617283951,0.786008230452675,0.788065843621399,0.790123456790123,
0.792181069958848,0.794238683127572,0.796296296296296,0.798353909465021,
0.800411522633745,0.802469135802469,0.804526748971193,0.806584362139918,
0.808641975308642,0.810699588477366,0.812757201646091,0.814814814814815,
0.816872427983539,0.818930041152263,0.820987654320988,0.823045267489712,
0.825102880658436,0.827160493827161,0.829218106995885,0.831275720164609,
0.833333333333333,0.835390946502058,0.837448559670782,0.839506172839506,
0.84156378600823,0.843621399176955,0.845679012345679,0.847736625514403,
0.849794238683128,0.851851851851852,0.853909465020576,0.8559670781893,0.858024691358025,
0.860082304526749,0.862139917695473,0.864197530864197,0.866255144032922,
0.868312757201646,0.87037037037037,0.872427983539095,0.874485596707819,
0.876543209876543,0.878600823045268,0.880658436213992,0.882716049382716,
0.88477366255144,0.886831275720165,0.888888888888889,0.890946502057613,
0.893004115226337,0.895061728395062,0.897119341563786,0.89917695473251,
0.901234567901235,0.903292181069959,0.905349794238683,0.907407407407407,
0.909465020576132,0.911522633744856,0.91358024691358,0.915637860082305,
0.917695473251029,0.919753086419753,0.921810699588477,0.923868312757202,
0.925925925925926,0.92798353909465,0.930041152263374,0.932098765432099,
0.934156378600823,0.936213991769547,0.938271604938272,0.940329218106996,
0.94238683127572,0.944444444444444,0.946502057613169,0.948559670781893,
0.950617283950617,0.952674897119342,0.954732510288066,0.95679012345679,
0.958847736625514,0.960905349794239,0.962962962962963,0.965020576131687,
0.967078189300412,0.969135802469136,0.97119341563786,0.973251028806584,
0.975308641975309,0.977366255144033,0.977769992664587),.UNSPECIFIED.)
CURVE()
GEOMETRIC_REPRESENTATION_ITEM()
RATIONAL_B_SPLINE_CURVE((0.948597702769161,0.96532364585481,1.,0.866025403784439,
1.,0.866025403784439,1.,0.866025403784439,1.,0.866025403784439,1.,0.866025403784439,
1.,0.866025403784439,1.,0.866025403784439,1.,0.866025403784439,1.,0.866025403784439,
1.,0.866025403784439,1.,0.866025403784439,1.,0.866025403784439,1.,0.866025403784439,
1.,0.866025403784439,1.,0.866025403784439,1.,0.866025403784439,1.,0.866025403784439,
1.,0.866025403784439,1.,0.866025403784439,1.,0.866025403784439,1.,0.866025403784439,
1.,0.866025403784439,1.,0.866025403784439,1.,0.866025403784439,1.,0.866025403784439,
1.,0.866025403784439,1.,0.866025403784439,1.,0.866025403784439,1.,0.866025403784439,
1.,0.866025403784439,1.,0.866025403784439,1.,0.866025403784439,1.,0.866025403784439,
1.,0.866025403784439,1.,0.866025403784439,1.,0.866025403784439,1.,0.866025403784439,
1.,0.866025403784439,1.,0.866025403784439,1.,0.866025403784439,1.,0.866025403784439,
1.,0.866025403784439,1.,0.866025403784439,1.,0.866025403784439,1.,0.866025403784439,
1.,0.866025403784439,1.,0.866025403784439,1.,0.866025403784439,1.,0.866025403784439,
1.,0.866025403784439,1.,0.866025403784439,1.,0.866025403784439,1.,0.866025403784439,
1.,0.866025403784439,1.,0.866025403784439,1.,0.866025403784439,1.,0.866025403784439,
1.,0.866025403784439,1.,0.866025403784439,1.,0.866025403784439,1.,0.866025403784439,
1.,0.866025403784439,1.,0.866025403784439,1.,0.866025403784439,1.,0.866025403784439,
1.,0.866025403784439,1.,0.866025403784439,1.,0.866025403784439,1.,0.866025403784439,
1.,0.866025403784439,1.,0.866025403784439,1.,0.866025403784439,1.,0.866025403784439,
1.,0.866025403784439,1.,0.866025403784439,1.,0.866025403784439,1.,0.866025403784439,
1.,0.866025403784439,1.,0.866025403784439,1.,0.866025403784439,1.,0.866025403784439,
1.,0.866025403784439,1.,0.866025403784439,1.,0.866025403784439,1.,0.866025403784439,
1.,0.866025403784439,1.,0.866025403784439,1.,0.866025403784439,1.,0.866025403784439,
1.,0.866025403784439,1.,0.866025403784439,1.,0.866025403784439,1.,0.866025403784439,
1.,0.866025403784439,1.,0.866025403784439,1.,0.866025403784439,1.,0.866025403784439,
1.,0.866025403784439,1.,0.866025403784439,1.,0.866025403784439,1.,0.866025403784439,
1.,0.866025403784439,1.,0.866025403784439,1.,0.866025403784439,1.,0.866025403784439,
1.,0.866025403784439,1.,0.866025403784439,1.,0.866025403784439,1.,0.866025403784439,
1.,0.866025403784439,1.,0.866025403784439,1.,0.866025403784439,1.,0.866025403784439,
1.,0.866025403784439,1.,0.866025403784439,1.,0.866025403784439,1.,0.866025403784439,
1.,0.866025403784439,1.,0.866025403784439,1.,0.866025403784439,1.,0.866025403784439,
1.,0.866025403784439,1.,0.866025403784439,1.,0.866025403784439,1.,0.866025403784439,
1.,0.866025403784439,1.,0.866025403784439,1.,0.866025403784439,1.,0.866025403784439,
1.,0.866025403784439,1.,0.866025403784439,1.,0.866025403784439,1.,0.866025403784439,
1.,0.866025403784439,1.,0.866025403784439,1.,0.866025403784439,1.,0.866025403784439,
1.,0.866025403784439,1.,0.866025403784439,1.,0.866025403784439,1.,0.866025403784439,
1.,0.866025403784439,1.,0.866025403784439,1.,0.866025403784439,1.,0.866025403784439,
1.,0.866025403784439,1.,0.866025403784439,1.,0.866025403784439,1.,0.866025403784439,
1.,0.866025403784439,1.,0.866025403784439,1.,0.866025403784439,1.,0.866025403784439,
1.,0.866025403784439,1.,0.866025403784439,1.,0.866025403784439,1.,0.866025403784439,
1.,0.866025403784439,1.,0.866025403784439,1.,0.866025403784439,1.,0.866025403784439,
1.,0.866025403784439,1.,0.866025403784439,1.,0.866025403784439,1.,0.866025403784439,
1.,0.866025403784439,1.,0.866025403784439,1.,0.866025403784439,1.,0.866025403784439,
1.,0.866025403784439,1.,0.866025403784439,1.,0.866025403784439,1.,0.866025403784439,
1.,0.866025403784439,1.,0.866025403784439,1.,0.866025403784439,1.,0.866025403784439,
1.,0.866025403784439,1.,0.866025403784439,1.,0.866025403784439,1.,0.866025403784439,
1.,0.866025403784439,1.,0.866025403784439,1.,0.866025403784439,1.,0.866025403784439,
1.,0.866025403784439,1.,0.866025403784439,1.,0.866025403784439,1.,0.866025403784439,
1.,0.866025403784439,1.,0.866025403784439,1.,0.866025403784439,1.,0.866025403784439,
1.,0.866025403784439,1.,0.866025403784439,1.,0.866025403784439,1.,0.866025403784439,
1.,0.866025403784439,1.,0.866025403784439,1.,0.866025403784439,1.,0.866025403784439,
1.,0.866025403784439,1.,0.866025403784439,1.,0.866025403784439,1.,0.866025403784439,
1.,0.866025403784439,1.,0.866025403784439,1.,0.866025403784439,1.,0.866025403784439,
1.,0.866025403784439,1.,0.866025403784439,1.,0.866025403784439,1.,0.866025403784439,
1.,0.866025403784439,1.,0.866025403784439,1.,0.866025403784439,1.,0.866025403784439,
1.,0.866025403784439,1.,0.866025403784439,1.,0.866025403784439,1.,0.866025403784439,
1.,0.866025403784439,1.,0.866025403784439,1.,0.866025403784439,1.,0.866025403784439,
1.,0.866025403784439,1.,0.866025403784439,1.,0.866025403784439,1.,0.866025403784439,
1.,0.866025403784439,1.,0.866025403784439,1.,0.866025403784439,1.,0.866025403784439,
1.,0.866025403784439,1.,0.866025403784439,1.,0.866025403784439,1.,0.866025403784439,
1.,0.866025403784439,1.,0.866025403784439,1.,0.866025403784439,1.,0.866025403784439,
1.,0.866025403784439,1.,0.866025403784439,1.,0.866025403784439,1.,0.866025403784439,
1.,0.866025403784439,1.,0.866025403784439,1.,0.866025403784439,1.,0.866025403784439,
1.,0.866025403784439,1.,0.866025403784439,1.,0.866025403784439,1.,0.866025403784439,
1.,0.866025403784439,1.,0.866025403784439,1.,0.866025403784439,1.,0.866025403784439,
1.,0.866025403784439,1.,0.866025403784439,1.,0.866025403784439,1.,0.866025403784439,
1.,0.866025403784439,1.,0.866025403784439,1.,0.866025403784439,1.,0.866025403784439,
1.,0.866025403784439,1.,0.866025403784439,1.,0.866025403784439,1.,0.866025403784439,
1.,0.866025403784439,1.,0.866025403784439,1.,0.866025403784439,1.,0.866025403784439,
1.,0.866025403784439,1.,0.866025403784439,1.,0.866025403784439,1.,0.866025403784439,
1.,0.866025403784439,1.,0.866025403784439,1.,0.866025403784439,1.,0.866025403784439,
1.,0.866025403784439,1.,0.866025403784439,1.,0.866025403784439,1.,0.866025403784439,
1.,0.866025403784439,1.,0.866025403784439,1.,0.866025403784439,1.,0.866025403784439,
1.,0.866025403784439,1.,0.866025403784439,1.,0.866025403784439,1.,0.866025403784439,
1.,0.866025403784439,1.,0.866025403784439,1.,0.866025403784439,1.,0.866025403784439,
1.,0.866025403784439,1.,0.866025403784439,1.,0.866025403784439,1.,0.866025403784439,
1.,0.866025403784439,1.,0.866025403784439,1.,0.866025403784439,1.,0.866025403784439,
1.,0.866025403784439,1.,0.866025403784439,1.,0.866025403784439,1.,0.866025403784439,
1.,0.866025403784439,1.,0.866025403784439,1.,0.866025403784439,1.,0.866025403784439,
1.,0.866025403784439,1.,0.866025403784439,1.,0.866025403784439,1.,0.866025403784439,
1.,0.866025403784439,1.,0.866025403784439,1.,0.866025403784439,1.,0.866025403784439,
1.,0.866025403784439,1.,0.866025403784439,1.,0.866025403784439,1.,0.866025403784439,
1.,0.866025403784439,1.,0.866025403784439,1.,0.866025403784439,1.,0.866025403784439,
1.,0.866025403784439,1.,0.866025403784439,1.,0.866025403784439,1.,0.866025403784439,
1.,0.866025403784439,1.,0.866025403784439,1.,0.866025403784439,1.,0.866025403784439,
1.,0.866025403784439,1.,0.866025403784439,1.,0.866025403784439,1.,0.866025403784439,
1.,0.866025403784439,1.,0.866025403784439,1.,0.866025403784439,1.,0.866025403784439,
1.,0.866025403784439,1.,0.866025403784439,1.,0.866025403784439,1.,0.866025403784439,
1.,0.866025403784439,1.,0.866025403784439,1.,0.866025403784439,1.,0.866025403784439,
1.,0.866025403784439,1.,0.866025403784439,1.,0.866025403784439,1.,0.866025403784439,
1.,0.866025403784439,1.,0.866025403784439,1.,0.866025403784439,1.,0.866025403784439,
1.,0.866025403784439,1.,0.866025403784439,1.,0.866025403784439,1.,0.866025403784439,
1.,0.866025403784439,1.,0.866025403784439,1.,0.866025403784439,1.,0.866025403784439,
1.,0.866025403784439,1.,0.866025403784439,1.,0.866025403784439,1.,0.866025403784439,
1.,0.866025403784439,1.,0.866025403784439,1.,0.866025403784439,1.,0.866025403784439,
1.,0.866025403784439,1.,0.866025403784439,1.,0.866025403784439,1.,0.866025403784439,
1.,0.866025403784439,1.,0.866025403784439,1.,0.866025403784439,1.,0.866025403784439,
1.,0.866025403784439,1.,0.866025403784439,1.,0.866025403784439,1.,0.866025403784439,
1.,0.866025403784439,1.,0.866025403784439,1.,0.866025403784439,1.,0.866025403784439,
1.,0.866025403784439,1.,0.866025403784439,1.,0.866025403784439,1.,0.866025403784439,
1.,0.866025403784439,1.,0.866025403784439,1.,0.866025403784439,1.,0.866025403784439,
1.,0.866025403784439,1.,0.866025403784439,1.,0.866025403784439,1.,0.866025403784439,
1.,0.866025403784439,1.,0.866025403784439,1.,0.866025403784439,1.,0.866025403784439,
1.,0.866025403784439,1.,0.866025403784439,1.,0.866025403784439,1.,0.866025403784439,
1.,0.866025403784439,1.,0.866025403784439,1.,0.866025403784439,1.,0.866025403784439,
1.,0.866025403784439,1.,0.866025403784439,1.,0.866025403784439,1.,0.866025403784439,
1.,0.866025403784439,1.,0.866025403784439,1.,0.866025403784439,1.,0.866025403784439,
1.,0.866025403784439,1.,0.866025403784439,1.,0.866025403784439,1.,0.866025403784439,
1.,0.866025403784439,1.,0.866025403784439,1.,0.866025403784439,1.,0.866025403784439,
1.,0.866025403784439,1.,0.866025403784439,1.,0.866025403784439,1.,0.866025403784439,
1.,0.866025403784439,1.,0.866025403784439,1.,0.866025403784439,1.,0.866025403784439,
1.,0.866025403784439,1.,0.866025403784439,1.,0.866025403784439,1.,0.866025403784439,
1.,0.866025403784439,1.,0.866025403784439,1.,0.866025403784439,1.,0.866025403784439,
1.,0.866025403784439,1.,0.866025403784439,1.,0.866025403784439,1.,0.866025403784439,
1.,0.866025403784439,1.,0.866025403784439,1.,0.866025403784439,1.,0.866025403784439,
1.,0.866025403784439,1.,0.866025403784439,1.,0.866025403784439,1.,0.866025403784439,
1.,0.866025403784439,1.,0.866025403784439,1.,0.866025403784439,1.,0.866025403784439,
1.,0.866025403784439,1.,0.866025403784439,1.,0.866025403784439,1.,0.866025403784439,
1.,0.866025403784439,1.,0.866025403784439,1.,0.973711982351429,0.957740246914744))
REPRESENTATION_ITEM('')
);
#201=(
BOUNDED_CURVE()
B_SPLINE_CURVE(2,(#31683,#31684,#31685,#31686,#31687,#31688,#31689,#31690,
#31691,#31692,#31693,#31694,#31695,#31696,#31697,#31698,#31699,#31700,#31701,
#31702,#31703,#31704,#31705,#31706,#31707,#31708,#31709,#31710,#31711,#31712,
#31713,#31714,#31715,#31716,#31717,#31718,#31719,#31720,#31721,#31722,#31723,
#31724,#31725,#31726,#31727,#31728,#31729,#31730,#31731,#31732,#31733,#31734,
#31735,#31736,#31737,#31738,#31739,#31740,#31741,#31742,#31743,#31744,#31745,
#31746,#31747,#31748,#31749,#31750,#31751,#31752,#31753,#31754,#31755,#31756,
#31757,#31758,#31759,#31760,#31761,#31762,#31763,#31764,#31765,#31766,#31767,
#31768,#31769,#31770,#31771,#31772,#31773,#31774,#31775,#31776,#31777,#31778,
#31779,#31780,#31781,#31782,#31783,#31784,#31785,#31786,#31787,#31788,#31789,
#31790,#31791,#31792,#31793,#31794,#31795,#31796,#31797,#31798,#31799,#31800,
#31801,#31802,#31803,#31804,#31805,#31806,#31807,#31808,#31809,#31810,#31811,
#31812,#31813,#31814,#31815,#31816,#31817,#31818,#31819,#31820,#31821,#31822,
#31823,#31824,#31825,#31826,#31827,#31828,#31829,#31830,#31831,#31832,#31833,
#31834,#31835,#31836,#31837,#31838,#31839,#31840,#31841,#31842,#31843,#31844,
#31845,#31846,#31847,#31848,#31849,#31850,#31851,#31852,#31853,#31854,#31855,
#31856,#31857,#31858,#31859,#31860,#31861,#31862,#31863,#31864,#31865,#31866,
#31867,#31868,#31869,#31870,#31871,#31872,#31873,#31874,#31875,#31876,#31877,
#31878,#31879,#31880,#31881,#31882,#31883,#31884,#31885,#31886,#31887,#31888,
#31889,#31890,#31891,#31892,#31893,#31894,#31895,#31896,#31897,#31898,#31899,
#31900,#31901,#31902,#31903,#31904,#31905,#31906,#31907,#31908,#31909,#31910,
#31911,#31912,#31913,#31914,#31915,#31916,#31917,#31918,#31919,#31920,#31921,
#31922,#31923,#31924,#31925,#31926,#31927,#31928,#31929,#31930,#31931,#31932,
#31933,#31934,#31935,#31936,#31937,#31938,#31939,#31940,#31941,#31942,#31943,
#31944,#31945,#31946,#31947,#31948,#31949,#31950,#31951,#31952,#31953,#31954,
#31955,#31956,#31957,#31958,#31959,#31960,#31961,#31962,#31963,#31964,#31965,
#31966,#31967,#31968,#31969,#31970,#31971,#31972,#31973,#31974,#31975,#31976,
#31977,#31978,#31979,#31980,#31981,#31982,#31983,#31984,#31985,#31986,#31987,
#31988,#31989,#31990,#31991,#31992,#31993,#31994,#31995,#31996,#31997,#31998,
#31999,#32000,#32001,#32002,#32003,#32004,#32005,#32006,#32007,#32008,#32009,
#32010,#32011,#32012,#32013,#32014,#32015,#32016,#32017,#32018,#32019,#32020,
#32021,#32022,#32023,#32024,#32025,#32026,#32027,#32028,#32029,#32030,#32031,
#32032,#32033,#32034,#32035,#32036,#32037,#32038,#32039,#32040,#32041,#32042,
#32043,#32044,#32045,#32046,#32047,#32048,#32049,#32050,#32051,#32052,#32053,
#32054,#32055,#32056,#32057,#32058,#32059,#32060,#32061,#32062,#32063,#32064,
#32065,#32066,#32067,#32068,#32069,#32070,#32071,#32072,#32073,#32074,#32075,
#32076,#32077,#32078,#32079,#32080,#32081,#32082,#32083,#32084,#32085,#32086,
#32087,#32088,#32089,#32090,#32091,#32092,#32093,#32094,#32095,#32096,#32097,
#32098,#32099,#32100,#32101,#32102,#32103,#32104,#32105,#32106,#32107,#32108,
#32109,#32110,#32111,#32112,#32113,#32114,#32115,#32116,#32117,#32118,#32119,
#32120,#32121,#32122,#32123,#32124,#32125,#32126,#32127,#32128,#32129,#32130,
#32131,#32132,#32133,#32134,#32135,#32136,#32137,#32138,#32139,#32140,#32141,
#32142,#32143,#32144,#32145,#32146,#32147,#32148,#32149,#32150,#32151,#32152,
#32153,#32154,#32155,#32156,#32157,#32158,#32159,#32160,#32161,#32162,#32163,
#32164,#32165,#32166,#32167,#32168,#32169,#32170,#32171,#32172,#32173,#32174,
#32175,#32176,#32177,#32178,#32179,#32180,#32181,#32182,#32183,#32184,#32185,
#32186,#32187,#32188,#32189,#32190,#32191,#32192,#32193,#32194,#32195,#32196,
#32197,#32198,#32199,#32200,#32201,#32202,#32203,#32204,#32205,#32206,#32207,
#32208,#32209,#32210,#32211,#32212,#32213,#32214,#32215,#32216,#32217,#32218,
#32219,#32220,#32221,#32222,#32223,#32224,#32225,#32226,#32227,#32228,#32229,
#32230,#32231,#32232,#32233,#32234,#32235,#32236,#32237,#32238,#32239,#32240,
#32241,#32242,#32243,#32244,#32245,#32246,#32247,#32248,#32249,#32250,#32251,
#32252,#32253,#32254,#32255,#32256,#32257,#32258,#32259,#32260,#32261,#32262,
#32263,#32264,#32265,#32266,#32267,#32268,#32269,#32270,#32271,#32272,#32273,
#32274,#32275,#32276,#32277,#32278,#32279,#32280,#32281,#32282,#32283,#32284,
#32285,#32286,#32287,#32288,#32289,#32290,#32291,#32292,#32293,#32294,#32295,
#32296,#32297,#32298,#32299,#32300,#32301,#32302,#32303,#32304,#32305,#32306,
#32307,#32308,#32309,#32310,#32311,#32312,#32313,#32314,#32315,#32316,#32317,
#32318,#32319,#32320,#32321,#32322,#32323,#32324,#32325,#32326,#32327,#32328,
#32329,#32330,#32331,#32332,#32333,#32334,#32335,#32336,#32337,#32338,#32339,
#32340,#32341,#32342,#32343,#32344,#32345,#32346,#32347,#32348,#32349,#32350,
#32351,#32352,#32353,#32354,#32355,#32356,#32357,#32358,#32359,#32360,#32361,
#32362,#32363,#32364,#32365,#32366,#32367,#32368,#32369,#32370,#32371,#32372,
#32373,#32374,#32375,#32376,#32377,#32378,#32379,#32380,#32381,#32382,#32383,
#32384,#32385,#32386,#32387,#32388,#32389,#32390,#32391,#32392,#32393,#32394,
#32395,#32396,#32397,#32398,#32399,#32400,#32401,#32402,#32403,#32404,#32405,
#32406,#32407,#32408,#32409,#32410,#32411,#32412,#32413,#32414,#32415,#32416,
#32417,#32418,#32419,#32420,#32421,#32422,#32423,#32424,#32425,#32426,#32427,
#32428,#32429,#32430,#32431,#32432,#32433,#32434,#32435,#32436,#32437,#32438,
#32439,#32440,#32441,#32442,#32443,#32444,#32445,#32446,#32447,#32448,#32449,
#32450,#32451,#32452,#32453,#32454,#32455,#32456,#32457,#32458,#32459,#32460,
#32461,#32462,#32463,#32464,#32465,#32466,#32467,#32468,#32469,#32470,#32471,
#32472,#32473,#32474,#32475,#32476,#32477,#32478,#32479,#32480,#32481,#32482,
#32483,#32484,#32485,#32486,#32487,#32488,#32489,#32490,#32491,#32492,#32493,
#32494,#32495,#32496,#32497,#32498,#32499,#32500,#32501,#32502,#32503,#32504,
#32505,#32506,#32507,#32508,#32509,#32510,#32511,#32512,#32513,#32514,#32515,
#32516,#32517,#32518,#32519,#32520,#32521,#32522,#32523,#32524,#32525,#32526,
#32527,#32528,#32529,#32530,#32531,#32532,#32533,#32534,#32535,#32536,#32537,
#32538,#32539,#32540,#32541,#32542,#32543,#32544,#32545,#32546,#32547,#32548,
#32549,#32550,#32551,#32552,#32553,#32554,#32555,#32556,#32557,#32558,#32559,
#32560,#32561,#32562,#32563,#32564,#32565,#32566,#32567,#32568,#32569,#32570,
#32571,#32572,#32573,#32574,#32575,#32576,#32577,#32578,#32579,#32580,#32581,
#32582,#32583,#32584,#32585,#32586,#32587,#32588,#32589,#32590,#32591,#32592,
#32593,#32594,#32595,#32596,#32597,#32598,#32599,#32600,#32601,#32602,#32603,
#32604,#32605,#32606,#32607,#32608,#32609,#32610,#32611,#32612,#32613,#32614,
#32615,#32616,#32617,#32618,#32619,#32620,#32621,#32622,#32623,#32624,#32625,
#32626,#32627),.UNSPECIFIED.,.F.,.F.)
B_SPLINE_CURVE_WITH_KNOTS((3,2,2,2,2,2,2,2,2,2,2,2,2,2,2,2,2,2,2,2,2,2,
2,2,2,2,2,2,2,2,2,2,2,2,2,2,2,2,2,2,2,2,2,2,2,2,2,2,2,2,2,2,2,2,2,2,2,2,
2,2,2,2,2,2,2,2,2,2,2,2,2,2,2,2,2,2,2,2,2,2,2,2,2,2,2,2,2,2,2,2,2,2,2,2,
2,2,2,2,2,2,2,2,2,2,2,2,2,2,2,2,2,2,2,2,2,2,2,2,2,2,2,2,2,2,2,2,2,2,2,2,
2,2,2,2,2,2,2,2,2,2,2,2,2,2,2,2,2,2,2,2,2,2,2,2,2,2,2,2,2,2,2,2,2,2,2,2,
2,2,2,2,2,2,2,2,2,2,2,2,2,2,2,2,2,2,2,2,2,2,2,2,2,2,2,2,2,2,2,2,2,2,2,2,
2,2,2,2,2,2,2,2,2,2,2,2,2,2,2,2,2,2,2,2,2,2,2,2,2,2,2,2,2,2,2,2,2,2,2,2,
2,2,2,2,2,2,2,2,2,2,2,2,2,2,2,2,2,2,2,2,2,2,2,2,2,2,2,2,2,2,2,2,2,2,2,2,
2,2,2,2,2,2,2,2,2,2,2,2,2,2,2,2,2,2,2,2,2,2,2,2,2,2,2,2,2,2,2,2,2,2,2,2,
2,2,2,2,2,2,2,2,2,2,2,2,2,2,2,2,2,2,2,2,2,2,2,2,2,2,2,2,2,2,2,2,2,2,2,2,
2,2,2,2,2,2,2,2,2,2,2,2,2,2,2,2,2,2,2,2,2,2,2,2,2,2,2,2,2,2,2,2,2,2,2,2,
2,2,2,2,2,2,2,2,2,2,2,2,2,2,2,2,2,2,2,2,2,2,2,2,2,2,2,2,2,2,2,2,2,2,2,2,
2,2,2,2,2,2,2,2,2,2,2,2,2,2,2,2,2,2,2,2,2,2,2,2,2,2,2,2,2,2,2,2,2,2,2,2,
2,2,2,2,2,2,2,2,2,2,2,2,2,2,2,2,2,2,3),(4.54089542788183E-5,0.00205761316872428,
0.00411522633744856,0.00617283950617284,0.00823045267489712,0.0102880658436214,
0.0123456790123457,0.01440329218107,0.0164609053497942,0.0185185185185185,
0.0205761316872428,0.0226337448559671,0.0246913580246914,0.0267489711934156,
0.0288065843621399,0.0308641975308642,0.0329218106995885,0.0349794238683128,
0.037037037037037,0.0390946502057613,0.0411522633744856,0.0432098765432099,
0.0452674897119342,0.0473251028806584,0.0493827160493827,0.051440329218107,
0.0534979423868313,0.0555555555555556,0.0576131687242798,0.0596707818930041,
0.0617283950617284,0.0637860082304527,0.065843621399177,0.0679012345679012,
0.0699588477366255,0.0720164609053498,0.0740740740740741,0.0761316872427984,
0.0781893004115226,0.0802469135802469,0.0823045267489712,0.0843621399176955,
0.0864197530864197,0.088477366255144,0.0905349794238683,0.0925925925925926,
0.0946502057613169,0.0967078189300412,0.0987654320987654,0.10082304526749,
0.102880658436214,0.104938271604938,0.106995884773663,0.109053497942387,
0.111111111111111,0.113168724279835,0.11522633744856,0.117283950617284,
0.119341563786008,0.121399176954733,0.123456790123457,0.125514403292181,
0.127572016460905,0.12962962962963,0.131687242798354,0.133744855967078,
0.135802469135802,0.137860082304527,0.139917695473251,0.141975308641975,
0.1440329218107,0.146090534979424,0.148148148148148,0.150205761316872,0.152263374485597,
0.154320987654321,0.156378600823045,0.15843621399177,0.160493827160494,
0.162551440329218,0.164609053497942,0.166666666666667,0.168724279835391,
0.170781893004115,0.172839506172839,0.174897119341564,0.176954732510288,
0.179012345679012,0.181069958847737,0.183127572016461,0.185185185185185,
0.187242798353909,0.189300411522634,0.191358024691358,0.193415637860082,
0.195473251028807,0.197530864197531,0.199588477366255,0.201646090534979,
0.203703703703704,0.205761316872428,0.207818930041152,0.209876543209877,
0.211934156378601,0.213991769547325,0.216049382716049,0.218106995884774,
0.220164609053498,0.222222222222222,0.224279835390947,0.226337448559671,
0.228395061728395,0.230452674897119,0.232510288065844,0.234567901234568,
0.236625514403292,0.238683127572016,0.240740740740741,0.242798353909465,
0.244855967078189,0.246913580246914,0.248971193415638,0.251028806584362,
0.253086419753086,0.255144032921811,0.257201646090535,0.259259259259259,
0.261316872427984,0.263374485596708,0.265432098765432,0.267489711934156,
0.269547325102881,0.271604938271605,0.273662551440329,0.275720164609054,
0.277777777777778,0.279835390946502,0.281893004115226,0.283950617283951,
0.286008230452675,0.288065843621399,0.290123456790123,0.292181069958848,
0.294238683127572,0.296296296296296,0.298353909465021,0.300411522633745,
0.302469135802469,0.304526748971193,0.306584362139918,0.308641975308642,
0.310699588477366,0.312757201646091,0.314814814814815,0.316872427983539,
0.318930041152263,0.320987654320988,0.323045267489712,0.325102880658436,
0.327160493827161,0.329218106995885,0.331275720164609,0.333333333333333,
0.335390946502058,0.337448559670782,0.339506172839506,0.34156378600823,
0.343621399176955,0.345679012345679,0.347736625514403,0.349794238683128,
0.351851851851852,0.353909465020576,0.3559670781893,0.358024691358025,0.360082304526749,
0.362139917695473,0.364197530864198,0.366255144032922,0.368312757201646,
0.37037037037037,0.372427983539095,0.374485596707819,0.376543209876543,
0.378600823045267,0.380658436213992,0.382716049382716,0.38477366255144,
0.386831275720165,0.388888888888889,0.390946502057613,0.393004115226337,
0.395061728395062,0.397119341563786,0.39917695473251,0.401234567901235,
0.403292181069959,0.405349794238683,0.407407407407407,0.409465020576132,
0.411522633744856,0.41358024691358,0.415637860082305,0.417695473251029,
0.419753086419753,0.421810699588477,0.423868312757202,0.425925925925926,
0.42798353909465,0.430041152263374,0.432098765432099,0.434156378600823,
0.436213991769547,0.438271604938272,0.440329218106996,0.44238683127572,
0.444444444444444,0.446502057613169,0.448559670781893,0.450617283950617,
0.452674897119342,0.454732510288066,0.45679012345679,0.458847736625514,
0.460905349794239,0.462962962962963,0.465020576131687,0.467078189300412,
0.469135802469136,0.47119341563786,0.473251028806584,0.475308641975309,
0.477366255144033,0.479423868312757,0.481481481481482,0.483539094650206,
0.48559670781893,0.487654320987654,0.489711934156379,0.491769547325103,
0.493827160493827,0.495884773662551,0.497942386831276,0.5,0.502057613168724,
0.504115226337449,0.506172839506173,0.508230452674897,0.510288065843621,
0.512345679012346,0.51440329218107,0.516460905349794,0.518518518518519,
0.520576131687243,0.522633744855967,0.524691358024691,0.526748971193416,
0.52880658436214,0.530864197530864,0.532921810699588,0.534979423868313,
0.537037037037037,0.539094650205761,0.541152263374486,0.54320987654321,
0.545267489711934,0.547325102880658,0.549382716049383,0.551440329218107,
0.553497942386831,0.555555555555556,0.55761316872428,0.559670781893004,
0.561728395061728,0.563786008230453,0.565843621399177,0.567901234567901,
0.569958847736626,0.57201646090535,0.574074074074074,0.576131687242798,
0.578189300411523,0.580246913580247,0.582304526748971,0.584362139917695,
0.58641975308642,0.588477366255144,0.590534979423868,0.592592592592593,
0.594650205761317,0.596707818930041,0.598765432098765,0.60082304526749,
0.602880658436214,0.604938271604938,0.606995884773663,0.609053497942387,
0.611111111111111,0.613168724279835,0.61522633744856,0.617283950617284,
0.619341563786008,0.621399176954732,0.623456790123457,0.625514403292181,
0.627572016460905,0.62962962962963,0.631687242798354,0.633744855967078,
0.635802469135803,0.637860082304527,0.639917695473251,0.641975308641975,
0.6440329218107,0.646090534979424,0.648148148148148,0.650205761316872,0.652263374485597,
0.654320987654321,0.656378600823045,0.65843621399177,0.660493827160494,
0.662551440329218,0.664609053497942,0.666666666666667,0.668724279835391,
0.670781893004115,0.672839506172839,0.674897119341564,0.676954732510288,
0.679012345679012,0.681069958847737,0.683127572016461,0.685185185185185,
0.687242798353909,0.689300411522634,0.691358024691358,0.693415637860082,
0.695473251028807,0.697530864197531,0.699588477366255,0.701646090534979,
0.703703703703704,0.705761316872428,0.707818930041152,0.709876543209877,
0.711934156378601,0.713991769547325,0.716049382716049,0.718106995884774,
0.720164609053498,0.722222222222222,0.724279835390947,0.726337448559671,
0.728395061728395,0.730452674897119,0.732510288065844,0.734567901234568,
0.736625514403292,0.738683127572016,0.740740740740741,0.742798353909465,
0.744855967078189,0.746913580246914,0.748971193415638,0.751028806584362,
0.753086419753086,0.755144032921811,0.757201646090535,0.759259259259259,
0.761316872427984,0.763374485596708,0.765432098765432,0.767489711934156,
0.769547325102881,0.771604938271605,0.773662551440329,0.775720164609053,
0.777777777777778,0.779835390946502,0.781893004115226,0.783950617283951,
0.786008230452675,0.788065843621399,0.790123456790123,0.792181069958848,
0.794238683127572,0.796296296296296,0.798353909465021,0.800411522633745,
0.802469135802469,0.804526748971193,0.806584362139918,0.808641975308642,
0.810699588477366,0.812757201646091,0.814814814814815,0.816872427983539,
0.818930041152263,0.820987654320988,0.823045267489712,0.825102880658436,
0.827160493827161,0.829218106995885,0.831275720164609,0.833333333333333,
0.835390946502058,0.837448559670782,0.839506172839506,0.84156378600823,
0.843621399176955,0.845679012345679,0.847736625514403,0.849794238683128,
0.851851851851852,0.853909465020576,0.8559670781893,0.858024691358025,0.860082304526749,
0.862139917695473,0.864197530864197,0.866255144032922,0.868312757201646,
0.87037037037037,0.872427983539095,0.874485596707819,0.876543209876543,
0.878600823045268,0.880658436213992,0.882716049382716,0.88477366255144,
0.886831275720165,0.888888888888889,0.890946502057613,0.893004115226337,
0.895061728395062,0.897119341563786,0.89917695473251,0.901234567901235,
0.903292181069959,0.905349794238683,0.907407407407407,0.909465020576132,
0.911522633744856,0.91358024691358,0.915637860082305,0.917695473251029,
0.919753086419753,0.921810699588477,0.923868312757202,0.925925925925926,
0.92798353909465,0.930041152263374,0.932098765432099,0.934156378600823,
0.936213991769547,0.938271604938272,0.940329218106996,0.94238683127572,
0.944444444444444,0.946502057613169,0.948559670781893,0.950617283950617,
0.952674897119342,0.954732510288066,0.95679012345679,0.958847736625514,
0.960905349794239,0.962962962962963,0.965020576131687,0.967078189300412,
0.969135802469136,0.970064444260615),.UNSPECIFIED.)
CURVE()
GEOMETRIC_REPRESENTATION_ITEM()
RATIONAL_B_SPLINE_CURVE((0.994217195025686,0.868982055893079,1.,0.866025403784439,
1.,0.866025403784439,1.,0.866025403784439,1.,0.866025403784439,1.,0.866025403784439,
1.,0.866025403784439,1.,0.866025403784439,1.,0.866025403784439,1.,0.866025403784439,
1.,0.866025403784439,1.,0.866025403784439,1.,0.866025403784439,1.,0.866025403784439,
1.,0.866025403784439,1.,0.866025403784439,1.,0.866025403784439,1.,0.866025403784439,
1.,0.866025403784439,1.,0.866025403784439,1.,0.866025403784439,1.,0.866025403784439,
1.,0.866025403784439,1.,0.866025403784439,1.,0.866025403784439,1.,0.866025403784439,
1.,0.866025403784439,1.,0.866025403784439,1.,0.866025403784439,1.,0.866025403784439,
1.,0.866025403784439,1.,0.866025403784439,1.,0.866025403784439,1.,0.866025403784439,
1.,0.866025403784439,1.,0.866025403784439,1.,0.866025403784439,1.,0.866025403784439,
1.,0.866025403784439,1.,0.866025403784439,1.,0.866025403784439,1.,0.866025403784439,
1.,0.866025403784439,1.,0.866025403784439,1.,0.866025403784439,1.,0.866025403784439,
1.,0.866025403784439,1.,0.866025403784439,1.,0.866025403784439,1.,0.866025403784439,
1.,0.866025403784439,1.,0.866025403784439,1.,0.866025403784439,1.,0.866025403784439,
1.,0.866025403784439,1.,0.866025403784439,1.,0.866025403784439,1.,0.866025403784439,
1.,0.866025403784439,1.,0.866025403784439,1.,0.866025403784439,1.,0.866025403784439,
1.,0.866025403784439,1.,0.866025403784439,1.,0.866025403784439,1.,0.866025403784439,
1.,0.866025403784439,1.,0.866025403784439,1.,0.866025403784439,1.,0.866025403784439,
1.,0.866025403784439,1.,0.866025403784439,1.,0.866025403784439,1.,0.866025403784439,
1.,0.866025403784439,1.,0.866025403784439,1.,0.866025403784439,1.,0.866025403784439,
1.,0.866025403784439,1.,0.866025403784439,1.,0.866025403784439,1.,0.866025403784439,
1.,0.866025403784439,1.,0.866025403784439,1.,0.866025403784439,1.,0.866025403784439,
1.,0.866025403784439,1.,0.866025403784439,1.,0.866025403784439,1.,0.866025403784439,
1.,0.866025403784439,1.,0.866025403784439,1.,0.866025403784439,1.,0.866025403784439,
1.,0.866025403784439,1.,0.866025403784439,1.,0.866025403784439,1.,0.866025403784439,
1.,0.866025403784439,1.,0.866025403784439,1.,0.866025403784439,1.,0.866025403784439,
1.,0.866025403784439,1.,0.866025403784439,1.,0.866025403784439,1.,0.866025403784439,
1.,0.866025403784439,1.,0.866025403784439,1.,0.866025403784439,1.,0.866025403784439,
1.,0.866025403784439,1.,0.866025403784439,1.,0.866025403784439,1.,0.866025403784439,
1.,0.866025403784439,1.,0.866025403784439,1.,0.866025403784439,1.,0.866025403784439,
1.,0.866025403784439,1.,0.866025403784439,1.,0.866025403784439,1.,0.866025403784439,
1.,0.866025403784439,1.,0.866025403784439,1.,0.866025403784439,1.,0.866025403784439,
1.,0.866025403784439,1.,0.866025403784439,1.,0.866025403784439,1.,0.866025403784439,
1.,0.866025403784439,1.,0.866025403784439,1.,0.866025403784439,1.,0.866025403784439,
1.,0.866025403784439,1.,0.866025403784439,1.,0.866025403784439,1.,0.866025403784439,
1.,0.866025403784439,1.,0.866025403784439,1.,0.866025403784439,1.,0.866025403784439,
1.,0.866025403784439,1.,0.866025403784439,1.,0.866025403784439,1.,0.866025403784439,
1.,0.866025403784439,1.,0.866025403784439,1.,0.866025403784439,1.,0.866025403784439,
1.,0.866025403784439,1.,0.866025403784439,1.,0.866025403784439,1.,0.866025403784439,
1.,0.866025403784439,1.,0.866025403784439,1.,0.866025403784439,1.,0.866025403784439,
1.,0.866025403784439,1.,0.866025403784439,1.,0.866025403784439,1.,0.866025403784439,
1.,0.866025403784439,1.,0.866025403784439,1.,0.866025403784439,1.,0.866025403784439,
1.,0.866025403784439,1.,0.866025403784439,1.,0.866025403784439,1.,0.866025403784439,
1.,0.866025403784439,1.,0.866025403784439,1.,0.866025403784439,1.,0.866025403784439,
1.,0.866025403784439,1.,0.866025403784439,1.,0.866025403784439,1.,0.866025403784439,
1.,0.866025403784439,1.,0.866025403784439,1.,0.866025403784439,1.,0.866025403784439,
1.,0.866025403784439,1.,0.866025403784439,1.,0.866025403784439,1.,0.866025403784439,
1.,0.866025403784439,1.,0.866025403784439,1.,0.866025403784439,1.,0.866025403784439,
1.,0.866025403784439,1.,0.866025403784439,1.,0.866025403784439,1.,0.866025403784439,
1.,0.866025403784439,1.,0.866025403784439,1.,0.866025403784439,1.,0.866025403784439,
1.,0.866025403784439,1.,0.866025403784439,1.,0.866025403784439,1.,0.866025403784439,
1.,0.866025403784439,1.,0.866025403784439,1.,0.866025403784439,1.,0.866025403784439,
1.,0.866025403784439,1.,0.866025403784439,1.,0.866025403784439,1.,0.866025403784439,
1.,0.866025403784439,1.,0.866025403784439,1.,0.866025403784439,1.,0.866025403784439,
1.,0.866025403784439,1.,0.866025403784439,1.,0.866025403784439,1.,0.866025403784439,
1.,0.866025403784439,1.,0.866025403784439,1.,0.866025403784439,1.,0.866025403784439,
1.,0.866025403784439,1.,0.866025403784439,1.,0.866025403784439,1.,0.866025403784439,
1.,0.866025403784439,1.,0.866025403784439,1.,0.866025403784439,1.,0.866025403784439,
1.,0.866025403784439,1.,0.866025403784439,1.,0.866025403784439,1.,0.866025403784439,
1.,0.866025403784439,1.,0.866025403784439,1.,0.866025403784439,1.,0.866025403784439,
1.,0.866025403784439,1.,0.866025403784439,1.,0.866025403784439,1.,0.866025403784439,
1.,0.866025403784439,1.,0.866025403784439,1.,0.866025403784439,1.,0.866025403784439,
1.,0.866025403784439,1.,0.866025403784439,1.,0.866025403784439,1.,0.866025403784439,
1.,0.866025403784439,1.,0.866025403784439,1.,0.866025403784439,1.,0.866025403784439,
1.,0.866025403784439,1.,0.866025403784439,1.,0.866025403784439,1.,0.866025403784439,
1.,0.866025403784439,1.,0.866025403784439,1.,0.866025403784439,1.,0.866025403784439,
1.,0.866025403784439,1.,0.866025403784439,1.,0.866025403784439,1.,0.866025403784439,
1.,0.866025403784439,1.,0.866025403784439,1.,0.866025403784439,1.,0.866025403784439,
1.,0.866025403784439,1.,0.866025403784439,1.,0.866025403784439,1.,0.866025403784439,
1.,0.866025403784439,1.,0.866025403784439,1.,0.866025403784439,1.,0.866025403784439,
1.,0.866025403784439,1.,0.866025403784439,1.,0.866025403784439,1.,0.866025403784439,
1.,0.866025403784439,1.,0.866025403784439,1.,0.866025403784439,1.,0.866025403784439,
1.,0.866025403784439,1.,0.866025403784439,1.,0.866025403784439,1.,0.866025403784439,
1.,0.866025403784439,1.,0.866025403784439,1.,0.866025403784439,1.,0.866025403784439,
1.,0.866025403784439,1.,0.866025403784439,1.,0.866025403784439,1.,0.866025403784439,
1.,0.866025403784439,1.,0.866025403784439,1.,0.866025403784439,1.,0.866025403784439,
1.,0.866025403784439,1.,0.866025403784439,1.,0.866025403784439,1.,0.866025403784439,
1.,0.866025403784439,1.,0.866025403784439,1.,0.866025403784439,1.,0.866025403784439,
1.,0.866025403784439,1.,0.866025403784439,1.,0.866025403784439,1.,0.866025403784439,
1.,0.866025403784439,1.,0.866025403784439,1.,0.866025403784439,1.,0.866025403784439,
1.,0.866025403784439,1.,0.866025403784439,1.,0.866025403784439,1.,0.866025403784439,
1.,0.866025403784439,1.,0.866025403784439,1.,0.866025403784439,1.,0.866025403784439,
1.,0.866025403784439,1.,0.866025403784439,1.,0.866025403784439,1.,0.866025403784439,
1.,0.866025403784439,1.,0.866025403784439,1.,0.866025403784439,1.,0.866025403784439,
1.,0.866025403784439,1.,0.866025403784439,1.,0.866025403784439,1.,0.866025403784439,
1.,0.866025403784439,1.,0.866025403784439,1.,0.866025403784439,1.,0.866025403784439,
1.,0.866025403784439,1.,0.866025403784439,1.,0.866025403784439,1.,0.866025403784439,
1.,0.866025403784439,1.,0.866025403784439,1.,0.866025403784439,1.,0.866025403784439,
1.,0.866025403784439,1.,0.866025403784439,1.,0.866025403784439,1.,0.866025403784439,
1.,0.866025403784439,1.,0.866025403784439,1.,0.866025403784439,1.,0.866025403784439,
1.,0.866025403784439,1.,0.866025403784439,1.,0.866025403784439,1.,0.866025403784439,
1.,0.866025403784439,1.,0.866025403784439,1.,0.866025403784439,1.,0.866025403784439,
1.,0.866025403784439,1.,0.866025403784439,1.,0.866025403784439,1.,0.866025403784439,
1.,0.866025403784439,1.,0.866025403784439,1.,0.866025403784439,1.,0.866025403784439,
1.,0.866025403784439,1.,0.866025403784439,1.,0.866025403784439,1.,0.866025403784439,
1.,0.866025403784439,1.,0.866025403784439,1.,0.866025403784439,1.,0.866025403784439,
1.,0.866025403784439,1.,0.866025403784439,1.,0.866025403784439,1.,0.866025403784439,
1.,0.866025403784439,1.,0.866025403784439,1.,0.866025403784439,1.,0.866025403784439,
1.,0.866025403784439,1.,0.866025403784439,1.,0.866025403784439,1.,0.866025403784439,
1.,0.866025403784439,1.,0.866025403784439,1.,0.866025403784439,1.,0.866025403784439,
1.,0.866025403784439,1.,0.866025403784439,1.,0.866025403784439,1.,0.866025403784439,
1.,0.866025403784439,1.,0.866025403784439,1.,0.866025403784439,1.,0.866025403784439,
1.,0.866025403784439,1.,0.866025403784439,1.,0.866025403784439,1.,0.866025403784439,
1.,0.866025403784439,1.,0.866025403784439,1.,0.866025403784439,1.,0.866025403784439,
1.,0.866025403784439,1.,0.866025403784439,1.,0.866025403784439,1.,0.866025403784439,
1.,0.866025403784439,1.,0.866025403784439,1.,0.866025403784439,1.,0.866025403784439,
1.,0.866025403784439,1.,0.866025403784439,1.,0.866025403784439,1.,0.866025403784439,
1.,0.866025403784439,1.,0.866025403784439,1.,0.866025403784439,1.,0.866025403784439,
1.,0.866025403784439,1.,0.866025403784439,1.,0.866025403784439,1.,0.866025403784439,
1.,0.866025403784439,1.,0.866025403784439,1.,0.866025403784439,1.,0.866025403784439,
1.,0.866025403784439,1.,0.866025403784439,1.,0.866025403784439,1.,0.866025403784439,
1.,0.866025403784439,1.,0.866025403784439,1.,0.866025403784439,1.,0.866025403784439,
1.,0.866025403784439,1.,0.866025403784439,1.,0.866025403784439,1.,0.866025403784439,
1.,0.866025403784439,1.,0.866025403784439,1.,0.866025403784439,1.,0.866025403784439,
1.,0.866025403784439,1.,0.866025403784439,1.,0.866025403784439,1.,0.866025403784439,
1.,0.866025403784439,1.,0.866025403784439,1.,0.866025403784439,1.,0.866025403784439,
1.,0.866025403784439,1.,0.866025403784439,1.,0.866025403784439,1.,0.866025403784439,
1.,0.866025403784439,1.,0.866025403784439,1.,0.866025403784439,1.,0.866025403784439,
1.,0.866025403784439,1.,0.939534597205461,0.933647674785266))
REPRESENTATION_ITEM('')
);
#202=(
BOUNDED_CURVE()
B_SPLINE_CURVE(2,(#36521,#36522,#36523,#36524,#36525,#36526,#36527,#36528,
#36529,#36530,#36531,#36532,#36533,#36534,#36535,#36536,#36537,#36538,#36539,
#36540,#36541,#36542,#36543,#36544,#36545,#36546,#36547,#36548,#36549,#36550,
#36551,#36552,#36553,#36554,#36555,#36556,#36557,#36558,#36559,#36560,#36561,
#36562,#36563,#36564,#36565,#36566,#36567,#36568,#36569,#36570,#36571,#36572,
#36573,#36574,#36575,#36576,#36577,#36578,#36579,#36580,#36581,#36582,#36583,
#36584,#36585,#36586,#36587,#36588,#36589,#36590,#36591,#36592,#36593,#36594,
#36595,#36596,#36597,#36598,#36599,#36600,#36601,#36602,#36603,#36604,#36605,
#36606,#36607,#36608,#36609,#36610,#36611,#36612,#36613,#36614,#36615,#36616,
#36617,#36618,#36619,#36620,#36621,#36622,#36623,#36624,#36625,#36626,#36627,
#36628,#36629,#36630,#36631,#36632,#36633,#36634,#36635,#36636,#36637,#36638,
#36639,#36640,#36641,#36642,#36643,#36644,#36645,#36646,#36647,#36648,#36649,
#36650,#36651,#36652,#36653,#36654,#36655,#36656,#36657,#36658,#36659,#36660,
#36661,#36662,#36663,#36664,#36665,#36666,#36667,#36668,#36669,#36670,#36671,
#36672,#36673,#36674,#36675,#36676,#36677,#36678,#36679,#36680,#36681,#36682,
#36683,#36684,#36685,#36686,#36687,#36688,#36689,#36690,#36691,#36692,#36693,
#36694,#36695,#36696,#36697,#36698,#36699,#36700,#36701,#36702,#36703,#36704,
#36705,#36706,#36707,#36708,#36709,#36710,#36711,#36712,#36713,#36714,#36715,
#36716,#36717,#36718,#36719,#36720,#36721,#36722,#36723,#36724,#36725,#36726,
#36727,#36728,#36729,#36730,#36731,#36732,#36733,#36734,#36735,#36736,#36737,
#36738,#36739,#36740,#36741,#36742,#36743,#36744,#36745,#36746,#36747,#36748,
#36749,#36750,#36751,#36752,#36753,#36754,#36755,#36756,#36757,#36758,#36759,
#36760,#36761,#36762,#36763,#36764,#36765,#36766,#36767,#36768,#36769,#36770,
#36771,#36772,#36773,#36774,#36775,#36776,#36777,#36778,#36779,#36780,#36781,
#36782,#36783,#36784,#36785,#36786,#36787,#36788,#36789,#36790,#36791,#36792,
#36793,#36794,#36795,#36796,#36797,#36798,#36799,#36800,#36801,#36802,#36803,
#36804,#36805,#36806,#36807,#36808,#36809,#36810,#36811,#36812,#36813,#36814,
#36815,#36816,#36817,#36818,#36819,#36820,#36821,#36822,#36823,#36824,#36825,
#36826,#36827,#36828,#36829,#36830,#36831,#36832,#36833,#36834,#36835,#36836,
#36837,#36838,#36839,#36840,#36841,#36842,#36843,#36844,#36845,#36846,#36847,
#36848,#36849,#36850,#36851,#36852,#36853,#36854,#36855,#36856,#36857,#36858,
#36859,#36860,#36861,#36862,#36863,#36864,#36865,#36866,#36867,#36868,#36869,
#36870,#36871,#36872,#36873,#36874,#36875,#36876,#36877,#36878,#36879,#36880,
#36881,#36882,#36883,#36884,#36885,#36886,#36887,#36888,#36889,#36890,#36891,
#36892,#36893,#36894,#36895,#36896,#36897,#36898,#36899,#36900,#36901,#36902,
#36903,#36904,#36905,#36906,#36907,#36908,#36909,#36910,#36911,#36912,#36913,
#36914,#36915,#36916,#36917,#36918,#36919,#36920,#36921,#36922,#36923,#36924,
#36925,#36926,#36927,#36928,#36929,#36930,#36931,#36932,#36933,#36934,#36935,
#36936,#36937,#36938,#36939,#36940,#36941,#36942,#36943,#36944,#36945,#36946,
#36947,#36948,#36949,#36950,#36951,#36952,#36953,#36954,#36955,#36956,#36957,
#36958,#36959,#36960,#36961,#36962,#36963,#36964,#36965,#36966,#36967,#36968,
#36969,#36970,#36971,#36972,#36973,#36974,#36975,#36976,#36977,#36978,#36979,
#36980,#36981,#36982,#36983,#36984,#36985,#36986,#36987,#36988,#36989,#36990,
#36991,#36992,#36993,#36994,#36995,#36996,#36997,#36998,#36999,#37000,#37001,
#37002,#37003,#37004,#37005,#37006,#37007,#37008,#37009,#37010,#37011,#37012,
#37013,#37014,#37015,#37016,#37017,#37018,#37019,#37020,#37021,#37022,#37023,
#37024,#37025,#37026,#37027,#37028,#37029,#37030,#37031,#37032,#37033,#37034,
#37035,#37036,#37037,#37038,#37039,#37040,#37041,#37042,#37043,#37044,#37045,
#37046,#37047,#37048,#37049,#37050,#37051,#37052,#37053,#37054,#37055,#37056,
#37057,#37058,#37059,#37060,#37061,#37062,#37063,#37064,#37065,#37066,#37067,
#37068,#37069,#37070,#37071,#37072,#37073,#37074,#37075,#37076,#37077,#37078,
#37079,#37080,#37081,#37082,#37083,#37084,#37085,#37086,#37087,#37088,#37089,
#37090,#37091,#37092,#37093,#37094,#37095,#37096,#37097,#37098,#37099,#37100,
#37101,#37102,#37103,#37104,#37105,#37106,#37107,#37108,#37109,#37110,#37111,
#37112,#37113,#37114,#37115,#37116,#37117,#37118,#37119,#37120,#37121,#37122,
#37123,#37124,#37125,#37126,#37127,#37128,#37129,#37130,#37131,#37132,#37133,
#37134,#37135,#37136,#37137,#37138,#37139,#37140,#37141,#37142,#37143,#37144,
#37145,#37146,#37147,#37148,#37149,#37150,#37151,#37152,#37153,#37154,#37155,
#37156,#37157,#37158,#37159,#37160,#37161,#37162,#37163,#37164,#37165,#37166,
#37167,#37168,#37169,#37170,#37171,#37172,#37173,#37174,#37175,#37176,#37177,
#37178,#37179,#37180,#37181,#37182,#37183,#37184,#37185,#37186,#37187,#37188,
#37189,#37190,#37191,#37192,#37193,#37194,#37195,#37196,#37197,#37198,#37199,
#37200,#37201,#37202,#37203,#37204,#37205,#37206,#37207,#37208,#37209,#37210,
#37211,#37212,#37213,#37214,#37215,#37216,#37217,#37218,#37219,#37220,#37221,
#37222,#37223,#37224,#37225,#37226,#37227,#37228,#37229,#37230,#37231,#37232,
#37233,#37234,#37235,#37236,#37237,#37238,#37239,#37240,#37241,#37242,#37243,
#37244,#37245,#37246,#37247,#37248,#37249,#37250,#37251,#37252,#37253,#37254,
#37255,#37256,#37257,#37258,#37259,#37260,#37261,#37262,#37263,#37264,#37265,
#37266,#37267,#37268,#37269,#37270,#37271,#37272,#37273,#37274,#37275,#37276,
#37277,#37278,#37279,#37280,#37281,#37282,#37283,#37284,#37285,#37286,#37287,
#37288,#37289,#37290,#37291,#37292,#37293,#37294,#37295,#37296,#37297,#37298,
#37299,#37300,#37301,#37302,#37303,#37304,#37305,#37306,#37307,#37308,#37309,
#37310,#37311,#37312,#37313,#37314,#37315,#37316,#37317,#37318,#37319,#37320,
#37321,#37322,#37323,#37324,#37325,#37326,#37327,#37328,#37329,#37330,#37331,
#37332,#37333,#37334,#37335,#37336,#37337,#37338,#37339,#37340,#37341,#37342,
#37343,#37344,#37345,#37346,#37347,#37348,#37349,#37350,#37351,#37352,#37353,
#37354,#37355,#37356,#37357,#37358,#37359,#37360,#37361,#37362,#37363,#37364,
#37365,#37366,#37367,#37368,#37369,#37370,#37371,#37372,#37373,#37374,#37375,
#37376,#37377,#37378,#37379,#37380,#37381,#37382,#37383,#37384,#37385,#37386,
#37387,#37388,#37389,#37390,#37391,#37392,#37393,#37394,#37395,#37396,#37397,
#37398,#37399,#37400,#37401,#37402,#37403,#37404,#37405,#37406,#37407,#37408,
#37409,#37410,#37411,#37412,#37413,#37414,#37415,#37416,#37417,#37418,#37419,
#37420,#37421,#37422,#37423,#37424,#37425,#37426,#37427,#37428,#37429,#37430,
#37431,#37432,#37433,#37434,#37435,#37436,#37437,#37438,#37439,#37440,#37441,
#37442,#37443,#37444,#37445,#37446,#37447,#37448,#37449,#37450,#37451,#37452,
#37453,#37454,#37455,#37456,#37457,#37458,#37459,#37460,#37461,#37462,#37463,
#37464,#37465),.UNSPECIFIED.,.F.,.F.)
B_SPLINE_CURVE_WITH_KNOTS((3,2,2,2,2,2,2,2,2,2,2,2,2,2,2,2,2,2,2,2,2,2,
2,2,2,2,2,2,2,2,2,2,2,2,2,2,2,2,2,2,2,2,2,2,2,2,2,2,2,2,2,2,2,2,2,2,2,2,
2,2,2,2,2,2,2,2,2,2,2,2,2,2,2,2,2,2,2,2,2,2,2,2,2,2,2,2,2,2,2,2,2,2,2,2,
2,2,2,2,2,2,2,2,2,2,2,2,2,2,2,2,2,2,2,2,2,2,2,2,2,2,2,2,2,2,2,2,2,2,2,2,
2,2,2,2,2,2,2,2,2,2,2,2,2,2,2,2,2,2,2,2,2,2,2,2,2,2,2,2,2,2,2,2,2,2,2,2,
2,2,2,2,2,2,2,2,2,2,2,2,2,2,2,2,2,2,2,2,2,2,2,2,2,2,2,2,2,2,2,2,2,2,2,2,
2,2,2,2,2,2,2,2,2,2,2,2,2,2,2,2,2,2,2,2,2,2,2,2,2,2,2,2,2,2,2,2,2,2,2,2,
2,2,2,2,2,2,2,2,2,2,2,2,2,2,2,2,2,2,2,2,2,2,2,2,2,2,2,2,2,2,2,2,2,2,2,2,
2,2,2,2,2,2,2,2,2,2,2,2,2,2,2,2,2,2,2,2,2,2,2,2,2,2,2,2,2,2,2,2,2,2,2,2,
2,2,2,2,2,2,2,2,2,2,2,2,2,2,2,2,2,2,2,2,2,2,2,2,2,2,2,2,2,2,2,2,2,2,2,2,
2,2,2,2,2,2,2,2,2,2,2,2,2,2,2,2,2,2,2,2,2,2,2,2,2,2,2,2,2,2,2,2,2,2,2,2,
2,2,2,2,2,2,2,2,2,2,2,2,2,2,2,2,2,2,2,2,2,2,2,2,2,2,2,2,2,2,2,2,2,2,2,2,
2,2,2,2,2,2,2,2,2,2,2,2,2,2,2,2,2,2,2,2,2,2,2,2,2,2,2,2,2,2,2,2,2,2,2,2,
2,2,2,2,2,2,2,2,2,2,2,2,2,2,2,2,2,2,3),(0.00472507824212208,0.00617283950617284,
0.00823045267489712,0.0102880658436214,0.0123456790123457,0.01440329218107,
0.0164609053497942,0.0185185185185185,0.0205761316872428,0.0226337448559671,
0.0246913580246914,0.0267489711934156,0.0288065843621399,0.0308641975308642,
0.0329218106995885,0.0349794238683128,0.037037037037037,0.0390946502057613,
0.0411522633744856,0.0432098765432099,0.0452674897119342,0.0473251028806584,
0.0493827160493827,0.051440329218107,0.0534979423868313,0.0555555555555556,
0.0576131687242798,0.0596707818930041,0.0617283950617284,0.0637860082304527,
0.065843621399177,0.0679012345679012,0.0699588477366255,0.0720164609053498,
0.0740740740740741,0.0761316872427984,0.0781893004115226,0.0802469135802469,
0.0823045267489712,0.0843621399176955,0.0864197530864197,0.088477366255144,
0.0905349794238683,0.0925925925925926,0.0946502057613169,0.0967078189300412,
0.0987654320987654,0.10082304526749,0.102880658436214,0.104938271604938,
0.106995884773663,0.109053497942387,0.111111111111111,0.113168724279835,
0.11522633744856,0.117283950617284,0.119341563786008,0.121399176954733,
0.123456790123457,0.125514403292181,0.127572016460905,0.12962962962963,
0.131687242798354,0.133744855967078,0.135802469135802,0.137860082304527,
0.139917695473251,0.141975308641975,0.1440329218107,0.146090534979424,0.148148148148148,
0.150205761316872,0.152263374485597,0.154320987654321,0.156378600823045,
0.15843621399177,0.160493827160494,0.162551440329218,0.164609053497942,
0.166666666666667,0.168724279835391,0.170781893004115,0.172839506172839,
0.174897119341564,0.176954732510288,0.179012345679012,0.181069958847737,
0.183127572016461,0.185185185185185,0.187242798353909,0.189300411522634,
0.191358024691358,0.193415637860082,0.195473251028807,0.197530864197531,
0.199588477366255,0.201646090534979,0.203703703703704,0.205761316872428,
0.207818930041152,0.209876543209877,0.211934156378601,0.213991769547325,
0.216049382716049,0.218106995884774,0.220164609053498,0.222222222222222,
0.224279835390947,0.226337448559671,0.228395061728395,0.230452674897119,
0.232510288065844,0.234567901234568,0.236625514403292,0.238683127572016,
0.240740740740741,0.242798353909465,0.244855967078189,0.246913580246914,
0.248971193415638,0.251028806584362,0.253086419753086,0.255144032921811,
0.257201646090535,0.259259259259259,0.261316872427984,0.263374485596708,
0.265432098765432,0.267489711934156,0.269547325102881,0.271604938271605,
0.273662551440329,0.275720164609054,0.277777777777778,0.279835390946502,
0.281893004115226,0.283950617283951,0.286008230452675,0.288065843621399,
0.290123456790123,0.292181069958848,0.294238683127572,0.296296296296296,
0.298353909465021,0.300411522633745,0.302469135802469,0.304526748971193,
0.306584362139918,0.308641975308642,0.310699588477366,0.312757201646091,
0.314814814814815,0.316872427983539,0.318930041152263,0.320987654320988,
0.323045267489712,0.325102880658436,0.327160493827161,0.329218106995885,
0.331275720164609,0.333333333333333,0.335390946502058,0.337448559670782,
0.339506172839506,0.34156378600823,0.343621399176955,0.345679012345679,
0.347736625514403,0.349794238683128,0.351851851851852,0.353909465020576,
0.3559670781893,0.358024691358025,0.360082304526749,0.362139917695473,0.364197530864198,
0.366255144032922,0.368312757201646,0.37037037037037,0.372427983539095,
0.374485596707819,0.376543209876543,0.378600823045267,0.380658436213992,
0.382716049382716,0.38477366255144,0.386831275720165,0.388888888888889,
0.390946502057613,0.393004115226337,0.395061728395062,0.397119341563786,
0.39917695473251,0.401234567901235,0.403292181069959,0.405349794238683,
0.407407407407407,0.409465020576132,0.411522633744856,0.41358024691358,
0.415637860082305,0.417695473251029,0.419753086419753,0.421810699588477,
0.423868312757202,0.425925925925926,0.42798353909465,0.430041152263374,
0.432098765432099,0.434156378600823,0.436213991769547,0.438271604938272,
0.440329218106996,0.44238683127572,0.444444444444444,0.446502057613169,
0.448559670781893,0.450617283950617,0.452674897119342,0.454732510288066,
0.45679012345679,0.458847736625514,0.460905349794239,0.462962962962963,
0.465020576131687,0.467078189300412,0.469135802469136,0.47119341563786,
0.473251028806584,0.475308641975309,0.477366255144033,0.479423868312757,
0.481481481481481,0.483539094650206,0.48559670781893,0.487654320987654,
0.489711934156379,0.491769547325103,0.493827160493827,0.495884773662551,
0.497942386831276,0.5,0.502057613168724,0.504115226337449,0.506172839506173,
0.508230452674897,0.510288065843621,0.512345679012346,0.51440329218107,
0.516460905349794,0.518518518518518,0.520576131687243,0.522633744855967,
0.524691358024691,0.526748971193416,0.52880658436214,0.530864197530864,
0.532921810699588,0.534979423868313,0.537037037037037,0.539094650205761,
0.541152263374486,0.54320987654321,0.545267489711934,0.547325102880658,
0.549382716049383,0.551440329218107,0.553497942386831,0.555555555555556,
0.55761316872428,0.559670781893004,0.561728395061728,0.563786008230453,
0.565843621399177,0.567901234567901,0.569958847736626,0.57201646090535,
0.574074074074074,0.576131687242798,0.578189300411523,0.580246913580247,
0.582304526748971,0.584362139917695,0.58641975308642,0.588477366255144,
0.590534979423868,0.592592592592593,0.594650205761317,0.596707818930041,
0.598765432098765,0.60082304526749,0.602880658436214,0.604938271604938,
0.606995884773663,0.609053497942387,0.611111111111111,0.613168724279835,
0.61522633744856,0.617283950617284,0.619341563786008,0.621399176954732,
0.623456790123457,0.625514403292181,0.627572016460905,0.62962962962963,
0.631687242798354,0.633744855967078,0.635802469135803,0.637860082304527,
0.639917695473251,0.641975308641975,0.6440329218107,0.646090534979424,0.648148148148148,
0.650205761316872,0.652263374485597,0.654320987654321,0.656378600823045,
0.65843621399177,0.660493827160494,0.662551440329218,0.664609053497942,
0.666666666666667,0.668724279835391,0.670781893004115,0.672839506172839,
0.674897119341564,0.676954732510288,0.679012345679012,0.681069958847737,
0.683127572016461,0.685185185185185,0.687242798353909,0.689300411522634,
0.691358024691358,0.693415637860082,0.695473251028807,0.697530864197531,
0.699588477366255,0.701646090534979,0.703703703703704,0.705761316872428,
0.707818930041152,0.709876543209877,0.711934156378601,0.713991769547325,
0.716049382716049,0.718106995884774,0.720164609053498,0.722222222222222,
0.724279835390947,0.726337448559671,0.728395061728395,0.730452674897119,
0.732510288065844,0.734567901234568,0.736625514403292,0.738683127572016,
0.740740740740741,0.742798353909465,0.744855967078189,0.746913580246914,
0.748971193415638,0.751028806584362,0.753086419753086,0.755144032921811,
0.757201646090535,0.759259259259259,0.761316872427984,0.763374485596708,
0.765432098765432,0.767489711934156,0.769547325102881,0.771604938271605,
0.773662551440329,0.775720164609053,0.777777777777778,0.779835390946502,
0.781893004115226,0.783950617283951,0.786008230452675,0.788065843621399,
0.790123456790123,0.792181069958848,0.794238683127572,0.796296296296296,
0.798353909465021,0.800411522633745,0.802469135802469,0.804526748971193,
0.806584362139918,0.808641975308642,0.810699588477366,0.812757201646091,
0.814814814814815,0.816872427983539,0.818930041152263,0.820987654320988,
0.823045267489712,0.825102880658436,0.827160493827161,0.829218106995885,
0.831275720164609,0.833333333333333,0.835390946502058,0.837448559670782,
0.839506172839506,0.84156378600823,0.843621399176955,0.845679012345679,
0.847736625514403,0.849794238683128,0.851851851851852,0.853909465020576,
0.8559670781893,0.858024691358025,0.860082304526749,0.862139917695473,0.864197530864197,
0.866255144032922,0.868312757201646,0.87037037037037,0.872427983539095,
0.874485596707819,0.876543209876543,0.878600823045268,0.880658436213992,
0.882716049382716,0.88477366255144,0.886831275720165,0.888888888888889,
0.890946502057613,0.893004115226337,0.895061728395062,0.897119341563786,
0.89917695473251,0.901234567901235,0.903292181069959,0.905349794238683,
0.907407407407407,0.909465020576132,0.911522633744856,0.91358024691358,
0.915637860082305,0.917695473251029,0.919753086419753,0.921810699588477,
0.923868312757202,0.925925925925926,0.92798353909465,0.930041152263374,
0.932098765432099,0.934156378600823,0.936213991769547,0.938271604938272,
0.940329218106996,0.94238683127572,0.944444444444444,0.946502057613169,
0.948559670781893,0.950617283950617,0.952674897119342,0.954732510288066,
0.95679012345679,0.958847736625514,0.960905349794239,0.962962962962963,
0.965020576131687,0.967078189300412,0.969135802469136,0.97119341563786,
0.973251028806584,0.974693312758157),.UNSPECIFIED.)
CURVE()
GEOMETRIC_REPRESENTATION_ITEM()
RATIONAL_B_SPLINE_CURVE((0.944121295592482,0.905733869846882,1.,0.866025403784439,
1.,0.866025403784439,1.,0.866025403784439,1.,0.866025403784439,1.,0.866025403784439,
1.,0.866025403784439,1.,0.866025403784439,1.,0.866025403784439,1.,0.866025403784439,
1.,0.866025403784439,1.,0.866025403784439,1.,0.866025403784439,1.,0.866025403784439,
1.,0.866025403784439,1.,0.866025403784439,1.,0.866025403784439,1.,0.866025403784439,
1.,0.866025403784439,1.,0.866025403784439,1.,0.866025403784439,1.,0.866025403784439,
1.,0.866025403784439,1.,0.866025403784439,1.,0.866025403784439,1.,0.866025403784439,
1.,0.866025403784439,1.,0.866025403784439,1.,0.866025403784439,1.,0.866025403784439,
1.,0.866025403784439,1.,0.866025403784439,1.,0.866025403784439,1.,0.866025403784439,
1.,0.866025403784439,1.,0.866025403784439,1.,0.866025403784439,1.,0.866025403784439,
1.,0.866025403784439,1.,0.866025403784439,1.,0.866025403784439,1.,0.866025403784439,
1.,0.866025403784439,1.,0.866025403784439,1.,0.866025403784439,1.,0.866025403784439,
1.,0.866025403784439,1.,0.866025403784439,1.,0.866025403784439,1.,0.866025403784439,
1.,0.866025403784439,1.,0.866025403784439,1.,0.866025403784439,1.,0.866025403784439,
1.,0.866025403784439,1.,0.866025403784439,1.,0.866025403784439,1.,0.866025403784439,
1.,0.866025403784439,1.,0.866025403784439,1.,0.866025403784439,1.,0.866025403784439,
1.,0.866025403784439,1.,0.866025403784439,1.,0.866025403784439,1.,0.866025403784439,
1.,0.866025403784439,1.,0.866025403784439,1.,0.866025403784439,1.,0.866025403784439,
1.,0.866025403784439,1.,0.866025403784439,1.,0.866025403784439,1.,0.866025403784439,
1.,0.866025403784439,1.,0.866025403784439,1.,0.866025403784439,1.,0.866025403784439,
1.,0.866025403784439,1.,0.866025403784439,1.,0.866025403784439,1.,0.866025403784439,
1.,0.866025403784439,1.,0.866025403784439,1.,0.866025403784439,1.,0.866025403784439,
1.,0.866025403784439,1.,0.866025403784439,1.,0.866025403784439,1.,0.866025403784439,
1.,0.866025403784439,1.,0.866025403784439,1.,0.866025403784439,1.,0.866025403784439,
1.,0.866025403784439,1.,0.866025403784439,1.,0.866025403784439,1.,0.866025403784439,
1.,0.866025403784439,1.,0.866025403784439,1.,0.866025403784439,1.,0.866025403784439,
1.,0.866025403784439,1.,0.866025403784439,1.,0.866025403784439,1.,0.866025403784439,
1.,0.866025403784439,1.,0.866025403784439,1.,0.866025403784439,1.,0.866025403784439,
1.,0.866025403784439,1.,0.866025403784439,1.,0.866025403784439,1.,0.866025403784439,
1.,0.866025403784439,1.,0.866025403784439,1.,0.866025403784439,1.,0.866025403784439,
1.,0.866025403784439,1.,0.866025403784439,1.,0.866025403784439,1.,0.866025403784439,
1.,0.866025403784439,1.,0.866025403784439,1.,0.866025403784439,1.,0.866025403784439,
1.,0.866025403784439,1.,0.866025403784439,1.,0.866025403784439,1.,0.866025403784439,
1.,0.866025403784439,1.,0.866025403784439,1.,0.866025403784439,1.,0.866025403784439,
1.,0.866025403784439,1.,0.866025403784439,1.,0.866025403784439,1.,0.866025403784439,
1.,0.866025403784439,1.,0.866025403784439,1.,0.866025403784439,1.,0.866025403784439,
1.,0.866025403784439,1.,0.866025403784439,1.,0.866025403784439,1.,0.866025403784439,
1.,0.866025403784439,1.,0.866025403784439,1.,0.866025403784439,1.,0.866025403784439,
1.,0.866025403784439,1.,0.866025403784439,1.,0.866025403784439,1.,0.866025403784439,
1.,0.866025403784439,1.,0.866025403784439,1.,0.866025403784439,1.,0.866025403784439,
1.,0.866025403784439,1.,0.866025403784439,1.,0.866025403784439,1.,0.866025403784439,
1.,0.866025403784439,1.,0.866025403784439,1.,0.866025403784439,1.,0.866025403784439,
1.,0.866025403784439,1.,0.866025403784439,1.,0.866025403784439,1.,0.866025403784439,
1.,0.866025403784439,1.,0.866025403784439,1.,0.866025403784439,1.,0.866025403784439,
1.,0.866025403784439,1.,0.866025403784439,1.,0.866025403784439,1.,0.866025403784439,
1.,0.866025403784439,1.,0.866025403784439,1.,0.866025403784439,1.,0.866025403784439,
1.,0.866025403784439,1.,0.866025403784439,1.,0.866025403784439,1.,0.866025403784439,
1.,0.866025403784439,1.,0.866025403784439,1.,0.866025403784439,1.,0.866025403784439,
1.,0.866025403784439,1.,0.866025403784439,1.,0.866025403784439,1.,0.866025403784439,
1.,0.866025403784439,1.,0.866025403784439,1.,0.866025403784439,1.,0.866025403784439,
1.,0.866025403784439,1.,0.866025403784439,1.,0.866025403784439,1.,0.866025403784439,
1.,0.866025403784439,1.,0.866025403784439,1.,0.866025403784439,1.,0.866025403784439,
1.,0.866025403784439,1.,0.866025403784439,1.,0.866025403784439,1.,0.866025403784439,
1.,0.866025403784439,1.,0.866025403784439,1.,0.866025403784439,1.,0.866025403784439,
1.,0.866025403784439,1.,0.866025403784439,1.,0.866025403784439,1.,0.866025403784439,
1.,0.866025403784439,1.,0.866025403784439,1.,0.866025403784439,1.,0.866025403784439,
1.,0.866025403784439,1.,0.866025403784439,1.,0.866025403784439,1.,0.866025403784439,
1.,0.866025403784439,1.,0.866025403784439,1.,0.866025403784439,1.,0.866025403784439,
1.,0.866025403784439,1.,0.866025403784439,1.,0.866025403784439,1.,0.866025403784439,
1.,0.866025403784439,1.,0.866025403784439,1.,0.866025403784439,1.,0.866025403784439,
1.,0.866025403784439,1.,0.866025403784439,1.,0.866025403784439,1.,0.866025403784439,
1.,0.866025403784439,1.,0.866025403784439,1.,0.866025403784439,1.,0.866025403784439,
1.,0.866025403784439,1.,0.866025403784439,1.,0.866025403784439,1.,0.866025403784439,
1.,0.866025403784439,1.,0.866025403784439,1.,0.866025403784439,1.,0.866025403784439,
1.,0.866025403784439,1.,0.866025403784439,1.,0.866025403784439,1.,0.866025403784439,
1.,0.866025403784439,1.,0.866025403784439,1.,0.866025403784439,1.,0.866025403784439,
1.,0.866025403784439,1.,0.866025403784439,1.,0.866025403784439,1.,0.866025403784439,
1.,0.866025403784439,1.,0.866025403784439,1.,0.866025403784439,1.,0.866025403784439,
1.,0.866025403784439,1.,0.866025403784439,1.,0.866025403784439,1.,0.866025403784439,
1.,0.866025403784439,1.,0.866025403784439,1.,0.866025403784439,1.,0.866025403784439,
1.,0.866025403784439,1.,0.866025403784439,1.,0.866025403784439,1.,0.866025403784439,
1.,0.866025403784439,1.,0.866025403784439,1.,0.866025403784439,1.,0.866025403784439,
1.,0.866025403784439,1.,0.866025403784439,1.,0.866025403784439,1.,0.866025403784439,
1.,0.866025403784439,1.,0.866025403784439,1.,0.866025403784439,1.,0.866025403784439,
1.,0.866025403784439,1.,0.866025403784439,1.,0.866025403784439,1.,0.866025403784439,
1.,0.866025403784439,1.,0.866025403784439,1.,0.866025403784439,1.,0.866025403784439,
1.,0.866025403784439,1.,0.866025403784439,1.,0.866025403784439,1.,0.866025403784439,
1.,0.866025403784439,1.,0.866025403784439,1.,0.866025403784439,1.,0.866025403784439,
1.,0.866025403784439,1.,0.866025403784439,1.,0.866025403784439,1.,0.866025403784439,
1.,0.866025403784439,1.,0.866025403784439,1.,0.866025403784439,1.,0.866025403784439,
1.,0.866025403784439,1.,0.866025403784439,1.,0.866025403784439,1.,0.866025403784439,
1.,0.866025403784439,1.,0.866025403784439,1.,0.866025403784439,1.,0.866025403784439,
1.,0.866025403784439,1.,0.866025403784439,1.,0.866025403784439,1.,0.866025403784439,
1.,0.866025403784439,1.,0.866025403784439,1.,0.866025403784439,1.,0.866025403784439,
1.,0.866025403784439,1.,0.866025403784439,1.,0.866025403784439,1.,0.866025403784439,
1.,0.866025403784439,1.,0.866025403784439,1.,0.866025403784439,1.,0.866025403784439,
1.,0.866025403784439,1.,0.866025403784439,1.,0.866025403784439,1.,0.866025403784439,
1.,0.866025403784439,1.,0.866025403784439,1.,0.866025403784439,1.,0.866025403784439,
1.,0.866025403784439,1.,0.866025403784439,1.,0.866025403784439,1.,0.866025403784439,
1.,0.866025403784439,1.,0.866025403784439,1.,0.866025403784439,1.,0.866025403784439,
1.,0.866025403784439,1.,0.866025403784439,1.,0.866025403784439,1.,0.866025403784439,
1.,0.866025403784439,1.,0.866025403784439,1.,0.866025403784439,1.,0.866025403784439,
1.,0.866025403784439,1.,0.866025403784439,1.,0.866025403784439,1.,0.866025403784439,
1.,0.866025403784439,1.,0.866025403784439,1.,0.866025403784439,1.,0.866025403784439,
1.,0.866025403784439,1.,0.866025403784439,1.,0.866025403784439,1.,0.866025403784439,
1.,0.866025403784439,1.,0.866025403784439,1.,0.866025403784439,1.,0.866025403784439,
1.,0.866025403784439,1.,0.866025403784439,1.,0.866025403784439,1.,0.866025403784439,
1.,0.866025403784439,1.,0.866025403784439,1.,0.866025403784439,1.,0.866025403784439,
1.,0.866025403784439,1.,0.866025403784439,1.,0.866025403784439,1.,0.866025403784439,
1.,0.866025403784439,1.,0.866025403784439,1.,0.866025403784439,1.,0.866025403784439,
1.,0.866025403784439,1.,0.866025403784439,1.,0.866025403784439,1.,0.866025403784439,
1.,0.866025403784439,1.,0.866025403784439,1.,0.866025403784439,1.,0.866025403784439,
1.,0.866025403784439,1.,0.866025403784439,1.,0.866025403784439,1.,0.866025403784439,
1.,0.866025403784439,1.,0.866025403784439,1.,0.866025403784439,1.,0.866025403784439,
1.,0.866025403784439,1.,0.866025403784439,1.,0.866025403784439,1.,0.866025403784439,
1.,0.866025403784439,1.,0.866025403784439,1.,0.866025403784439,1.,0.866025403784439,
1.,0.866025403784439,1.,0.866025403784439,1.,0.866025403784439,1.,0.866025403784439,
1.,0.866025403784439,1.,0.866025403784439,1.,0.866025403784439,1.,0.866025403784439,
1.,0.866025403784439,1.,0.866025403784439,1.,0.866025403784439,1.,0.866025403784439,
1.,0.866025403784439,1.,0.866025403784439,1.,0.866025403784439,1.,0.866025403784439,
1.,0.866025403784439,1.,0.866025403784439,1.,0.866025403784439,1.,0.866025403784439,
1.,0.866025403784439,1.,0.866025403784439,1.,0.866025403784439,1.,0.866025403784439,
1.,0.866025403784439,1.,0.866025403784439,1.,0.866025403784439,1.,0.866025403784439,
1.,0.866025403784439,1.,0.866025403784439,1.,0.866025403784439,1.,0.866025403784439,
1.,0.866025403784439,1.,0.866025403784439,1.,0.866025403784439,1.,0.866025403784439,
1.,0.866025403784439,1.,0.866025403784439,1.,0.866025403784439,1.,0.866025403784439,
1.,0.866025403784439,1.,0.866025403784439,1.,0.866025403784439,1.,0.866025403784439,
1.,0.866025403784439,1.,0.866025403784439,1.,0.866025403784439,1.,0.866025403784439,
1.,0.866025403784439,1.,0.906090506720528,0.94383273215671))
REPRESENTATION_ITEM('')
);
#203=(
BOUNDED_CURVE()
B_SPLINE_CURVE(2,(#39448,#39449,#39450),.UNSPECIFIED.,.F.,.F.)
B_SPLINE_CURVE_WITH_KNOTS((3,3),(-2.2693844624543,-1.90898280074519),
 .UNSPECIFIED.)
CURVE()
GEOMETRIC_REPRESENTATION_ITEM()
RATIONAL_B_SPLINE_CURVE((1.7477494971405,1.72129587968328,1.68438569901946))
REPRESENTATION_ITEM('')
);
#204=(
BOUNDED_CURVE()
B_SPLINE_CURVE(2,(#39453,#39454,#39455),.UNSPECIFIED.,.F.,.F.)
B_SPLINE_CURVE_WITH_KNOTS((3,3),(-4.45331599749568,-4.09291433578657),
 .UNSPECIFIED.)
CURVE()
GEOMETRIC_REPRESENTATION_ITEM()
RATIONAL_B_SPLINE_CURVE((1.68438569901946,1.72129587968328,1.7477494971405))
REPRESENTATION_ITEM('')
);
#205=(
BOUNDED_CURVE()
B_SPLINE_CURVE(2,(#39462,#39463,#39464),.UNSPECIFIED.,.F.,.F.)
B_SPLINE_CURVE_WITH_KNOTS((3,3),(-2.2693844624543,-1.90898280074519),
 .UNSPECIFIED.)
CURVE()
GEOMETRIC_REPRESENTATION_ITEM()
RATIONAL_B_SPLINE_CURVE((1.7477494971405,1.72129587968328,1.68438569901946))
REPRESENTATION_ITEM('')
);
#206=(
BOUNDED_CURVE()
B_SPLINE_CURVE(2,(#39467,#39468,#39469),.UNSPECIFIED.,.F.,.F.)
B_SPLINE_CURVE_WITH_KNOTS((3,3),(-4.45331599749568,-4.09291433578656),
 .UNSPECIFIED.)
CURVE()
GEOMETRIC_REPRESENTATION_ITEM()
RATIONAL_B_SPLINE_CURVE((1.68438569901946,1.72129587968328,1.7477494971405))
REPRESENTATION_ITEM('')
);
#207=(
BOUNDED_CURVE()
B_SPLINE_CURVE(2,(#39476,#39477,#39478),.UNSPECIFIED.,.F.,.F.)
B_SPLINE_CURVE_WITH_KNOTS((3,3),(-2.2693844624543,-1.90898280074518),
 .UNSPECIFIED.)
CURVE()
GEOMETRIC_REPRESENTATION_ITEM()
RATIONAL_B_SPLINE_CURVE((1.7477494971405,1.72129587968328,1.68438569901946))
REPRESENTATION_ITEM('')
);
#208=(
BOUNDED_CURVE()
B_SPLINE_CURVE(2,(#39481,#39482,#39483),.UNSPECIFIED.,.F.,.F.)
B_SPLINE_CURVE_WITH_KNOTS((3,3),(-4.45331599749568,-4.09291433578656),
 .UNSPECIFIED.)
CURVE()
GEOMETRIC_REPRESENTATION_ITEM()
RATIONAL_B_SPLINE_CURVE((1.68438569901946,1.72129587968328,1.7477494971405))
REPRESENTATION_ITEM('')
);
#209=(
BOUNDED_CURVE()
B_SPLINE_CURVE(2,(#39490,#39491,#39492),.UNSPECIFIED.,.F.,.F.)
B_SPLINE_CURVE_WITH_KNOTS((3,3),(-2.2693844624543,-1.90898280074518),
 .UNSPECIFIED.)
CURVE()
GEOMETRIC_REPRESENTATION_ITEM()
RATIONAL_B_SPLINE_CURVE((1.7477494971405,1.72129587968328,1.68438569901946))
REPRESENTATION_ITEM('')
);
#210=(
BOUNDED_CURVE()
B_SPLINE_CURVE(2,(#39495,#39496,#39497),.UNSPECIFIED.,.F.,.F.)
B_SPLINE_CURVE_WITH_KNOTS((3,3),(-4.45331599749568,-4.09291433578657),
 .UNSPECIFIED.)
CURVE()
GEOMETRIC_REPRESENTATION_ITEM()
RATIONAL_B_SPLINE_CURVE((1.68438569901946,1.72129587968328,1.7477494971405))
REPRESENTATION_ITEM('')
);
#211=(
BOUNDED_CURVE()
B_SPLINE_CURVE(2,(#39504,#39505,#39506),.UNSPECIFIED.,.F.,.F.)
B_SPLINE_CURVE_WITH_KNOTS((3,3),(-4.45331599749568,-4.09291433578656),
 .UNSPECIFIED.)
CURVE()
GEOMETRIC_REPRESENTATION_ITEM()
RATIONAL_B_SPLINE_CURVE((1.68438569901946,1.72129587968328,1.7477494971405))
REPRESENTATION_ITEM('')
);
#212=(
BOUNDED_CURVE()
B_SPLINE_CURVE(2,(#39510,#39511,#39512),.UNSPECIFIED.,.F.,.F.)
B_SPLINE_CURVE_WITH_KNOTS((3,3),(-2.2693844624543,-1.90898280074519),
 .UNSPECIFIED.)
CURVE()
GEOMETRIC_REPRESENTATION_ITEM()
RATIONAL_B_SPLINE_CURVE((1.7477494971405,1.72129587968328,1.68438569901946))
REPRESENTATION_ITEM('')
);
#277=PLANE('',#6723);
#278=PLANE('',#6724);
#279=PLANE('',#6725);
#280=PLANE('',#6726);
#281=PLANE('',#6727);
#282=PLANE('',#6728);
#283=PLANE('',#6729);
#284=PLANE('',#6730);
#285=PLANE('',#6731);
#286=PLANE('',#6732);
#287=PLANE('',#6743);
#346=FACE_BOUND('',#1077,.T.);
#347=FACE_BOUND('',#1079,.T.);
#348=FACE_BOUND('',#1081,.T.);
#349=FACE_BOUND('',#1086,.T.);
#350=FACE_BOUND('',#1094,.T.);
#377=CONICAL_SURFACE('',#6704,12.7,0.785398163397453);
#378=CONICAL_SURFACE('',#6712,7.4375,0.785398163397444);
#379=CONICAL_SURFACE('',#6713,11.7,0.78539816339744);
#380=CONICAL_SURFACE('',#6733,12.7,0.785398163397453);
#381=CONICAL_SURFACE('',#6735,12.7,0.785398163397453);
#382=CONICAL_SURFACE('',#6737,12.7,0.785398163397453);
#383=CONICAL_SURFACE('',#6739,12.7,0.785398163397453);
#384=CONICAL_SURFACE('',#6741,12.7,0.785398163397453);
#462=ELLIPSE('',#6707,2.36743243982073,1.24520550947174);
#674=FACE_OUTER_BOUND('',#1068,.T.);
#675=FACE_OUTER_BOUND('',#1069,.T.);
#676=FACE_OUTER_BOUND('',#1070,.T.);
#677=FACE_OUTER_BOUND('',#1071,.T.);
#678=FACE_OUTER_BOUND('',#1072,.T.);
#679=FACE_OUTER_BOUND('',#1073,.T.);
#680=FACE_OUTER_BOUND('',#1074,.T.);
#681=FACE_OUTER_BOUND('',#1075,.T.);
#682=FACE_OUTER_BOUND('',#1076,.T.);
#683=FACE_OUTER_BOUND('',#1078,.T.);
#684=FACE_OUTER_BOUND('',#1080,.T.);
#685=FACE_OUTER_BOUND('',#1082,.T.);
#686=FACE_OUTER_BOUND('',#1083,.T.);
#687=FACE_OUTER_BOUND('',#1084,.T.);
#688=FACE_OUTER_BOUND('',#1085,.T.);
#689=FACE_OUTER_BOUND('',#1087,.T.);
#690=FACE_OUTER_BOUND('',#1088,.T.);
#691=FACE_OUTER_BOUND('',#1089,.T.);
#692=FACE_OUTER_BOUND('',#1090,.T.);
#693=FACE_OUTER_BOUND('',#1091,.T.);
#694=FACE_OUTER_BOUND('',#1092,.T.);
#695=FACE_OUTER_BOUND('',#1093,.T.);
#696=FACE_OUTER_BOUND('',#1095,.T.);
#697=FACE_OUTER_BOUND('',#1096,.T.);
#698=FACE_OUTER_BOUND('',#1097,.T.);
#699=FACE_OUTER_BOUND('',#1098,.T.);
#700=FACE_OUTER_BOUND('',#1099,.T.);
#701=FACE_OUTER_BOUND('',#1100,.T.);
#702=FACE_OUTER_BOUND('',#1101,.T.);
#703=FACE_OUTER_BOUND('',#1102,.T.);
#1068=EDGE_LOOP('',(#4758,#4759,#4760,#4761,#4762,#4763));
#1069=EDGE_LOOP('',(#4764,#4765,#4766,#4767,#4768,#4769));
#1070=EDGE_LOOP('',(#4770,#4771,#4772));
#1071=EDGE_LOOP('',(#4773,#4774,#4775,#4776,#4777,#4778,#4779,#4780,#4781,
#4782));
#1072=EDGE_LOOP('',(#4783,#4784,#4785,#4786,#4787));
#1073=EDGE_LOOP('',(#4788,#4789,#4790,#4791));
#1074=EDGE_LOOP('',(#4792,#4793,#4794,#4795,#4796));
#1075=EDGE_LOOP('',(#4797,#4798,#4799,#4800));
#1076=EDGE_LOOP('',(#4801,#4802,#4803,#4804,#4805,#4806,#4807,#4808,#4809,
#4810,#4811));
#1077=EDGE_LOOP('',(#4812,#4813,#4814,#4815));
#1078=EDGE_LOOP('',(#4816));
#1079=EDGE_LOOP('',(#4817));
#1080=EDGE_LOOP('',(#4818,#4819,#4820));
#1081=EDGE_LOOP('',(#4821));
#1082=EDGE_LOOP('',(#4822,#4823,#4824,#4825));
#1083=EDGE_LOOP('',(#4826,#4827,#4828,#4829));
#1084=EDGE_LOOP('',(#4830,#4831,#4832,#4833));
#1085=EDGE_LOOP('',(#4834,#4835,#4836));
#1086=EDGE_LOOP('',(#4837));
#1087=EDGE_LOOP('',(#4838,#4839,#4840,#4841,#4842,#4843));
#1088=EDGE_LOOP('',(#4844,#4845,#4846,#4847,#4848,#4849));
#1089=EDGE_LOOP('',(#4850,#4851,#4852,#4853,#4854,#4855));
#1090=EDGE_LOOP('',(#4856,#4857,#4858,#4859,#4860,#4861));
#1091=EDGE_LOOP('',(#4862,#4863,#4864,#4865,#4866,#4867));
#1092=EDGE_LOOP('',(#4868,#4869,#4870,#4871,#4872,#4873));
#1093=EDGE_LOOP('',(#4874));
#1094=EDGE_LOOP('',(#4875,#4876,#4877,#4878,#4879,#4880));
#1095=EDGE_LOOP('',(#4881,#4882,#4883));
#1096=EDGE_LOOP('',(#4884,#4885,#4886));
#1097=EDGE_LOOP('',(#4887,#4888,#4889));
#1098=EDGE_LOOP('',(#4890,#4891,#4892));
#1099=EDGE_LOOP('',(#4893,#4894,#4895));
#1100=EDGE_LOOP('',(#4896,#4897,#4898,#4899,#4900,#4901,#4902,#4903,#4904,
#4905,#4906,#4907));
#1101=EDGE_LOOP('',(#4908,#4909,#4910,#4911,#4912,#4913));
#1102=EDGE_LOOP('',(#4914,#4915,#4916,#4917,#4918,#4919));
#1447=CIRCLE('',#6699,0.5);
#1448=CIRCLE('',#6700,0.5);
#1449=CIRCLE('',#6701,0.500000000000002);
#1450=CIRCLE('',#6702,5.39635281288848);
#1451=CIRCLE('',#6703,0.499999999999999);
#1452=CIRCLE('',#6705,11.7);
#1453=CIRCLE('',#6709,7.4375);
#1454=CIRCLE('',#6710,7.4375);
#1455=CIRCLE('',#6711,7.4375);
#1456=CIRCLE('',#6714,12.7);
#1457=CIRCLE('',#6715,12.7);
#1458=CIRCLE('',#6716,11.7);
#1459=CIRCLE('',#6718,7.70000000000001);
#1460=CIRCLE('',#6719,7.7);
#1461=CIRCLE('',#6721,12.7);
#1462=CIRCLE('',#6722,5.31464415841409);
#1463=CIRCLE('',#6734,11.7);
#1464=CIRCLE('',#6736,11.7);
#1465=CIRCLE('',#6738,11.7);
#1466=CIRCLE('',#6740,11.7);
#1467=CIRCLE('',#6742,11.7);
#1806=B_SPLINE_CURVE_WITH_KNOTS('',3,(#27294,#27295,#27296,#27297,#27298,
#27299,#27300,#27301,#27302,#27303,#27304,#27305,#27306,#27307,#27308,#27309,
#27310,#27311,#27312,#27313,#27314,#27315,#27316,#27317,#27318,#27319,#27320,
#27321,#27322,#27323,#27324,#27325,#27326,#27327,#27328,#27329,#27330,#27331,
#27332,#27333,#27334,#27335,#27336,#27337,#27338,#27339,#27340,#27341,#27342,
#27343,#27344,#27345,#27346,#27347,#27348,#27349,#27350,#27351,#27352,#27353,
#27354,#27355,#27356,#27357,#27358,#27359,#27360,#27361,#27362,#27363,#27364,
#27365,#27366,#27367,#27368,#27369,#27370,#27371,#27372,#27373,#27374,#27375,
#27376,#27377,#27378,#27379,#27380,#27381,#27382,#27383,#27384,#27385,#27386,
#27387,#27388,#27389,#27390,#27391,#27392,#27393,#27394,#27395,#27396,#27397,
#27398,#27399,#27400,#27401,#27402,#27403,#27404,#27405,#27406,#27407,#27408,
#27409,#27410,#27411,#27412,#27413,#27414,#27415,#27416,#27417,#27418,#27419,
#27420,#27421,#27422,#27423,#27424,#27425,#27426,#27427,#27428,#27429,#27430,
#27431,#27432,#27433,#27434,#27435,#27436,#27437,#27438,#27439,#27440,#27441,
#27442,#27443,#27444,#27445,#27446,#27447,#27448,#27449,#27450,#27451,#27452,
#27453,#27454,#27455,#27456,#27457,#27458,#27459,#27460,#27461,#27462,#27463,
#27464,#27465),.UNSPECIFIED.,.F.,.F.,(4,3,3,3,3,3,3,3,3,3,3,3,3,3,3,3,3,
3,3,3,3,3,3,3,3,3,3,3,3,3,3,3,3,3,3,3,3,3,3,3,3,3,3,3,3,3,3,3,3,3,3,3,3,
3,3,3,3,4),(0.0161972991085284,0.0165394666975099,0.0168809221214402,0.0172044026463048,
0.0176094804041076,0.0180166563712003,0.0182115061840812,0.019004889187358,
0.0192186097218576,0.0195483730729979,0.0198870431663159,0.020225713259634,
0.0205303601960963,0.0208345896758242,0.0211387162338752,0.0212328167974104,
0.0215681677457675,0.0219040440404771,0.0222399203351868,0.0224639690092825,
0.0226878387172806,0.022743472104075,0.0230854328330104,0.0232470238729632,
0.0235831943749047,0.0237505756418514,0.023959762309833,0.0241688808757419,
0.0242541274107396,0.0245936504558835,0.0249356019729133,0.025261230948516,
0.025525825317406,0.0257903817038414,0.026055729922731,0.0262683344862924,
0.0266058569357826,0.0269447878928871,0.0272754380240688,0.0275032853685415,
0.0277312867104389,0.027778989792957,0.0281109815849333,0.0282825415618451,
0.0286824722061837,0.0290770552629352,0.0292896450996216,0.029623506776701,
0.0299601277070495,0.030296748637398,0.0305741027539414,0.0308509225425318,
0.031127629650921,0.0313038521751744,0.0316222885798555,0.0319394577071118,
0.0322532614556433,0.0323109557129508),.UNSPECIFIED.);
#1807=B_SPLINE_CURVE_WITH_KNOTS('',3,(#27469,#27470,#27471,#27472,#27473,
#27474,#27475,#27476,#27477,#27478,#27479,#27480,#27481,#27482,#27483,#27484,
#27485,#27486,#27487,#27488,#27489,#27490,#27491,#27492,#27493,#27494,#27495,
#27496,#27497,#27498,#27499,#27500,#27501,#27502,#27503,#27504,#27505,#27506,
#27507,#27508,#27509,#27510,#27511,#27512,#27513,#27514,#27515,#27516,#27517,
#27518,#27519,#27520,#27521,#27522,#27523,#27524,#27525,#27526,#27527,#27528,
#27529,#27530,#27531,#27532,#27533,#27534,#27535,#27536,#27537,#27538,#27539,
#27540,#27541,#27542,#27543,#27544,#27545,#27546,#27547,#27548,#27549,#27550),
 .UNSPECIFIED.,.F.,.F.,(4,3,3,3,3,3,3,3,3,3,3,3,3,3,3,3,3,3,3,3,3,3,3,3,
3,3,3,4),(0.00890915223960435,0.0094204624297249,0.00946241028514952,0.00998728674902293,
0.0100156683306947,0.0105532850043369,0.0105689263762399,0.0111184026693338,
0.0111221844217851,0.0119717719779961,0.0122287005128754,0.0122437820923162,
0.0128330281524603,0.0133352166039658,0.0133620354339848,0.0140734232108796,
0.0144417326950561,0.0144721766299634,0.0151217140130995,0.0155482487861465,
0.0155745146428516,0.0161015068316917,0.0161230651642655,0.0166190777279675,
0.0166547648772369,0.0166698085595632,0.0173648818539917,0.0177612809683272),
 .UNSPECIFIED.);
#1808=B_SPLINE_CURVE_WITH_KNOTS('',3,(#27552,#27553,#27554,#27555,#27556,
#27557,#27558,#27559,#27560,#27561,#27562,#27563,#27564,#27565,#27566,#27567,
#27568,#27569,#27570,#27571),.UNSPECIFIED.,.F.,.F.,(4,2,2,2,2,2,2,2,2,4),
(0.0355734865786901,0.0366931658727571,0.037812845166824,0.0389325244608909,
0.0400522037549579,0.0406120434019913,0.0411718830490248,0.0422915623430917,
0.0434112416371587,0.0445309209312256),.UNSPECIFIED.);
#1809=B_SPLINE_CURVE_WITH_KNOTS('',3,(#27574,#27575,#27576,#27577),
 .UNSPECIFIED.,.F.,.F.,(4,4),(0.,4.45846292526202E-5),.UNSPECIFIED.);
#1810=B_SPLINE_CURVE_WITH_KNOTS('',3,(#27706,#27707,#27708,#27709,#27710,
#27711,#27712,#27713,#27714,#27715,#27716,#27717,#27718,#27719,#27720,#27721,
#27722,#27723,#27724,#27725,#27726,#27727,#27728,#27729,#27730,#27731,#27732,
#27733,#27734,#27735,#27736,#27737,#27738,#27739,#27740,#27741,#27742,#27743,
#27744,#27745,#27746,#27747,#27748,#27749,#27750,#27751,#27752,#27753,#27754,
#27755,#27756,#27757,#27758,#27759,#27760,#27761,#27762,#27763,#27764,#27765,
#27766,#27767,#27768,#27769,#27770,#27771,#27772,#27773,#27774,#27775,#27776,
#27777,#27778,#27779,#27780,#27781,#27782,#27783,#27784,#27785,#27786,#27787,
#27788,#27789,#27790),.UNSPECIFIED.,.F.,.F.,(4,3,3,3,3,3,3,3,3,3,3,3,3,
3,3,3,3,3,3,3,3,3,3,3,3,3,3,3,4),(0.0163404601436347,0.0173256833684261,
0.0173478922432849,0.0177073599341222,0.0178182949808219,0.0178520374467346,
0.0182545320008027,0.0183109065932176,0.0183567651649381,0.0187303101652621,
0.0191065909074555,0.0192961298180091,0.0193676144802671,0.0197533601995195,
0.0201449367067774,0.0202813530428006,0.0203798282124602,0.021266576267592,
0.0213919424331495,0.0222517994923835,0.0224025672000064,0.0229070517959347,
0.023237022717175,0.0234111125329635,0.0236644536869744,0.0237804896972582,
0.0239146520071729,0.0242030183124513,0.0242222459419665),.UNSPECIFIED.);
#1811=B_SPLINE_CURVE_WITH_KNOTS('',3,(#27794,#27795,#27796,#27797,#27798,
#27799,#27800,#27801,#27802,#27803,#27804,#27805,#27806,#27807,#27808,#27809,
#27810,#27811,#27812,#27813,#27814,#27815,#27816,#27817,#27818,#27819,#27820,
#27821,#27822,#27823,#27824,#27825,#27826,#27827,#27828,#27829,#27830,#27831,
#27832,#27833,#27834,#27835,#27836,#27837,#27838,#27839,#27840,#27841,#27842,
#27843,#27844,#27845,#27846,#27847,#27848,#27849,#27850,#27851,#27852,#27853,
#27854,#27855,#27856,#27857,#27858,#27859,#27860,#27861,#27862,#27863,#27864,
#27865,#27866,#27867,#27868,#27869,#27870,#27871,#27872,#27873,#27874,#27875,
#27876,#27877,#27878,#27879,#27880,#27881,#27882,#27883,#27884,#27885,#27886,
#27887,#27888,#27889,#27890,#27891,#27892,#27893,#27894,#27895,#27896,#27897,
#27898,#27899,#27900,#27901,#27902,#27903,#27904,#27905,#27906,#27907,#27908,
#27909,#27910,#27911,#27912,#27913,#27914,#27915,#27916,#27917,#27918,#27919,
#27920,#27921,#27922,#27923,#27924,#27925,#27926,#27927,#27928,#27929,#27930,
#27931,#27932,#27933,#27934,#27935,#27936,#27937,#27938,#27939,#27940,#27941,
#27942,#27943,#27944,#27945,#27946,#27947,#27948,#27949,#27950,#27951,#27952,
#27953,#27954,#27955,#27956,#27957,#27958,#27959,#27960,#27961,#27962,#27963,
#27964,#27965,#27966,#27967,#27968,#27969,#27970,#27971,#27972,#27973,#27974,
#27975,#27976,#27977,#27978,#27979,#27980,#27981,#27982,#27983,#27984,#27985,
#27986),.UNSPECIFIED.,.F.,.F.,(4,3,3,3,3,3,3,3,3,3,3,3,3,3,3,3,3,3,3,3,
3,3,3,3,3,3,3,3,3,3,3,3,3,3,3,3,3,3,3,3,3,3,3,3,3,3,3,3,3,3,3,3,3,3,3,3,
3,3,3,3,3,3,3,3,4),(0.,0.000476483257676747,0.000920430129810064,0.00110270427003711,
0.0016586651891166,0.00205477723046485,0.00220540854007422,0.00261403414264452,
0.00302622462762113,0.00318437350442038,0.00330811281011133,0.00369591663725892,
0.00408676590346633,0.00430673855116764,0.00441081708014843,0.0048197443595792,
0.00486501447903157,0.00496216921516699,0.00531164477891051,0.00542124469901969,
0.00551352135018555,0.00602068054519799,0.00652783974021042,0.00661622562022266,
0.00701845057040251,0.00743031416521327,0.00762708503273923,0.00771892989025977,
0.00822053759859568,0.00872214530693159,0.00882163416029687,0.00911084512080088,
0.00926867571247231,0.00937298629531544,0.00981572542009721,0.009924338430334,
0.0102952256348079,0.0103637517719452,0.0104756905653526,0.0107825930307397,
0.0109128329030101,0.0110270427003711,0.0118184582616005,0.0120162612334194,
0.0121297469704082,0.012410398075847,0.0126810991054268,0.0130200359460735,
0.0131274071843423,0.0132324512404454,0.0136546231592765,0.0140734930528288,
0.0142469357400738,0.0143351555104825,0.0147312308823071,0.0151293577222552,
0.0153736058156945,0.0154378597805196,0.0158451722172866,0.0159393472249651,
0.0159892119155382,0.0164350035042047,0.0165066770945964,0.0165405640505567,
0.0176432683205938),.UNSPECIFIED.);
#1812=B_SPLINE_CURVE_WITH_KNOTS('',3,(#27991,#27992,#27993,#27994,#27995,
#27996,#27997,#27998,#27999,#28000,#28001,#28002,#28003,#28004,#28005,#28006,
#28007,#28008,#28009,#28010,#28011,#28012,#28013,#28014,#28015,#28016,#28017,
#28018,#28019,#28020,#28021,#28022,#28023,#28024,#28025,#28026,#28027,#28028,
#28029,#28030,#28031,#28032,#28033,#28034,#28035,#28036,#28037,#28038,#28039,
#28040,#28041,#28042,#28043,#28044,#28045,#28046,#28047,#28048,#28049,#28050,
#28051,#28052,#28053,#28054,#28055,#28056,#28057,#28058,#28059,#28060,#28061,
#28062,#28063,#28064,#28065,#28066,#28067,#28068,#28069,#28070,#28071,#28072,
#28073,#28074,#28075),.UNSPECIFIED.,.F.,.F.,(4,3,3,3,3,3,3,3,3,3,3,3,3,
3,3,3,3,3,3,3,3,3,3,3,3,3,3,3,4),(0.0242222459426628,0.0244180431366776,
0.0250670610002247,0.0252558702165362,0.0254257993687501,0.0258101580369982,
0.0261920397107803,0.0262894944911059,0.0264352581025446,0.0268818610381716,
0.0273231187656756,0.0274466088771079,0.0279527924666284,0.0283567430402452,
0.0284590391121063,0.0288583023070336,0.0292494335045575,0.0293903673148149,
0.0294708328719711,0.0298842927152321,0.0302930478895242,0.0304239915893846,
0.0304812062897893,0.0310833961140862,0.0314576158639543,0.0314886932089115,
0.0318206160521525,0.0321559280953382,0.032491240138524),.UNSPECIFIED.);
#1813=B_SPLINE_CURVE_WITH_KNOTS('',3,(#28089,#28090,#28091,#28092,#28093,
#28094,#28095,#28096,#28097,#28098,#28099,#28100,#28101,#28102,#28103,#28104,
#28105,#28106,#28107,#28108,#28109,#28110,#28111,#28112,#28113,#28114,#28115,
#28116,#28117,#28118,#28119,#28120,#28121,#28122,#28123,#28124,#28125,#28126,
#28127,#28128,#28129,#28130,#28131,#28132,#28133,#28134,#28135,#28136,#28137,
#28138,#28139,#28140,#28141,#28142,#28143,#28144,#28145,#28146,#28147,#28148,
#28149,#28150,#28151,#28152,#28153,#28154,#28155,#28156,#28157,#28158,#28159,
#28160,#28161,#28162,#28163,#28164),.UNSPECIFIED.,.F.,.F.,(4,3,3,3,3,3,
3,3,3,3,3,3,3,3,3,3,3,3,3,3,3,3,3,3,3,4),(0.00807103269296787,0.00826343092632988,
0.00876686013716756,0.00910471112411131,0.00927072398918449,0.0101383895554718,
0.0102800255304896,0.0106156018941836,0.010655228771152,0.0110644258204309,
0.0111720679868323,0.0112913127308201,0.0117973861554865,0.0122057464181927,
0.0123035593154063,0.0132394248495532,0.0133153163713804,0.0138374104952791,
0.0142731032809137,0.0143254514319448,0.0148760179492037,0.0153067817122742,
0.0153336346080776,0.0156869818471577,0.0160337318414785,0.0163404601436347),
 .UNSPECIFIED.);
#1814=B_SPLINE_CURVE_WITH_KNOTS('',3,(#28168,#28169,#28170,#28171,#28172,
#28173,#28174,#28175,#28176,#28177,#28178,#28179,#28180,#28181,#28182,#28183,
#28184,#28185,#28186,#28187,#28188,#28189,#28190,#28191,#28192,#28193,#28194,
#28195,#28196,#28197,#28198,#28199,#28200,#28201,#28202,#28203,#28204,#28205,
#28206,#28207,#28208,#28209,#28210,#28211,#28212,#28213,#28214,#28215,#28216,
#28217,#28218,#28219,#28220,#28221,#28222,#28223,#28224,#28225,#28226,#28227,
#28228,#28229,#28230,#28231,#28232,#28233,#28234,#28235,#28236,#28237,#28238,
#28239,#28240,#28241,#28242,#28243,#28244,#28245,#28246,#28247,#28248,#28249,
#28250,#28251,#28252,#28253,#28254,#28255,#28256,#28257,#28258,#28259,#28260,
#28261,#28262,#28263,#28264,#28265,#28266,#28267,#28268,#28269,#28270,#28271,
#28272,#28273,#28274,#28275,#28276,#28277,#28278,#28279,#28280,#28281,#28282,
#28283,#28284,#28285,#28286,#28287,#28288,#28289,#28290,#28291,#28292,#28293,
#28294,#28295,#28296,#28297,#28298,#28299,#28300,#28301,#28302,#28303,#28304,
#28305,#28306,#28307,#28308,#28309,#28310,#28311,#28312,#28313,#28314,#28315,
#28316,#28317,#28318,#28319,#28320,#28321),.UNSPECIFIED.,.F.,.F.,(4,3,3,
3,3,3,3,3,3,3,3,3,3,3,3,3,3,3,3,3,3,3,3,3,3,3,3,3,3,3,3,3,3,3,3,3,3,3,3,
3,3,3,3,3,3,3,3,3,3,3,3,4),(4.45846292526202E-5,0.00105045630092898,0.00105093952698816,
0.0014376794093111,0.00155285871031254,0.00191803247755761,0.00205655415239476,
0.0020572944247237,0.00279642434499595,0.00306364932245924,0.00306768917245999,
0.00383461365631528,0.00407000422019478,0.0040800681747585,0.00507635911793032,
0.00509211131047192,0.0055976346059631,0.00608271401566585,0.00610269177361662,
0.00658589146453362,0.00660721081063723,0.00699582755236498,0.00708906891340139,
0.00711120248307089,0.00772832521421459,0.00809542381113692,0.0081185518555815,
0.00854575157131149,0.00859860126000469,0.00862200314174437,0.00910177870887246,
0.00912580243443331,0.010108133606608,0.0101346994725071,0.0110502314226318,
0.0111144885043435,0.0111454360522996,0.0116514589397514,0.0121208434020791,
0.0121576802258181,0.0129515084587526,0.0131271982998146,0.0131700170813561,
0.013745821675725,0.0141335531975501,0.014181101651953,0.0147833538088824,
0.0151399080952856,0.0151901066138265,0.0155690496395463,0.0159361916298065,
0.0161462629930212),.UNSPECIFIED.);
#1815=B_SPLINE_CURVE_WITH_KNOTS('',3,(#28322,#28323,#28324,#28325,#28326,
#28327,#28328,#28329,#28330,#28331,#28332,#28333,#28334,#28335,#28336,#28337,
#28338,#28339,#28340,#28341,#28342,#28343),.UNSPECIFIED.,.F.,.F.,(4,2,2,
2,2,2,2,2,2,2,4),(0.000187655515302136,0.00117307766248322,0.00166578873607376,
0.00215849980966431,0.0031439219568454,0.00412934410402649,0.00511476625120758,
0.00610018839838867,0.00659289947197922,0.00708561054556976,0.00807103269275084),
 .UNSPECIFIED.);
#1816=B_SPLINE_CURVE_WITH_KNOTS('',3,(#28372,#28373,#28374,#28375,#28376,
#28377,#28378,#28379,#28380,#28381,#28382,#28383,#28384,#28385,#28386,#28387,
#28388,#28389,#28390,#28391,#28392,#28393,#28394,#28395,#28396,#28397,#28398,
#28399,#28400,#28401,#28402,#28403,#28404,#28405,#28406,#28407,#28408,#28409,
#28410,#28411,#28412,#28413,#28414,#28415,#28416,#28417,#28418,#28419,#28420,
#28421,#28422,#28423,#28424,#28425,#28426,#28427,#28428,#28429,#28430,#28431,
#28432,#28433,#28434,#28435,#28436,#28437,#28438,#28439,#28440,#28441,#28442,
#28443,#28444,#28445,#28446,#28447,#28448,#28449,#28450,#28451,#28452,#28453,
#28454,#28455,#28456,#28457,#28458,#28459),.UNSPECIFIED.,.F.,.F.,(4,3,3,
3,3,3,3,3,3,3,3,3,3,3,3,3,3,3,3,3,3,3,3,3,3,3,3,3,3,4),(0.0177612809683272,
0.0179912055960288,0.0182264943827035,0.018320985239376,0.0186309863592005,
0.0188517626649399,0.0188806895104249,0.0195327263331859,0.0199466791231638,
0.0200000980525225,0.0205240586547836,0.02100811078643,0.0210480192570447,
0.0211195065946202,0.0218330559323615,0.0221573969432929,0.0222389151367179,
0.0227150057367735,0.0232746671940726,0.0233583236788155,0.0240758493690848,
0.0243994308669159,0.0244777322209132,0.0254514724876917,0.025529773750765,
0.0255971407630109,0.0260964347561723,0.0261568450340597,0.0266638537201985,
0.0267165493051086),.UNSPECIFIED.);
#1817=B_SPLINE_CURVE_WITH_KNOTS('',3,(#28463,#28464,#28465,#28466,#28467,
#28468,#28469,#28470,#28471,#28472,#28473,#28474,#28475,#28476,#28477,#28478,
#28479,#28480,#28481,#28482,#28483,#28484,#28485,#28486,#28487,#28488,#28489,
#28490,#28491,#28492,#28493,#28494,#28495,#28496,#28497,#28498,#28499,#28500,
#28501,#28502,#28503,#28504,#28505,#28506,#28507,#28508,#28509,#28510,#28511,
#28512,#28513,#28514,#28515,#28516,#28517,#28518,#28519,#28520,#28521,#28522,
#28523,#28524,#28525,#28526,#28527,#28528,#28529,#28530,#28531,#28532,#28533,
#28534,#28535,#28536,#28537,#28538,#28539,#28540,#28541),.UNSPECIFIED.,
 .F.,.F.,(4,3,3,3,3,3,3,3,3,3,3,3,3,3,3,3,3,3,3,3,3,3,3,3,3,3,4),(0.0267165493051086,
0.0273773663586454,0.0277977530222155,0.0278236664643063,0.0283640328899012,
0.0283772250439051,0.0289289794857498,0.028930783623504,0.029492481704934,
0.0300379007827017,0.0300544056967581,0.0308713360248079,0.0311450179418994,
0.0311725469988184,0.0317293956286949,0.0322521351010971,0.0322826877003502,
0.0330325553019409,0.0333592522602948,0.033385001375028,0.0337665202189872,
0.0339128108398936,0.0339332548501144,0.0344663694194925,0.0344806499432494,
0.0353087686546496,0.0355734865786901),.UNSPECIFIED.);
#1818=B_SPLINE_CURVE_WITH_KNOTS('',3,(#28544,#28545,#28546,#28547,#28548,
#28549,#28550,#28551,#28552,#28553,#28554,#28555,#28556,#28557,#28558,#28559,
#28560,#28561,#28562,#28563,#28564,#28565,#28566,#28567,#28568,#28569,#28570,
#28571,#28572,#28573,#28574,#28575,#28576,#28577,#28578,#28579,#28580,#28581,
#28582,#28583,#28584,#28585,#28586,#28587,#28588,#28589,#28590,#28591,#28592,
#28593,#28594,#28595,#28596,#28597,#28598,#28599,#28600,#28601,#28602,#28603,
#28604,#28605,#28606,#28607,#28608,#28609,#28610,#28611,#28612,#28613,#28614,
#28615,#28616,#28617,#28618,#28619,#28620,#28621,#28622,#28623,#28624,#28625,
#28626,#28627,#28628,#28629,#28630,#28631,#28632,#28633,#28634,#28635,#28636,
#28637,#28638,#28639,#28640,#28641,#28642,#28643,#28644,#28645,#28646,#28647,
#28648,#28649,#28650,#28651,#28652,#28653,#28654,#28655,#28656,#28657,#28658,
#28659,#28660,#28661,#28662,#28663,#28664,#28665,#28666,#28667,#28668,#28669,
#28670,#28671,#28672,#28673,#28674,#28675,#28676,#28677,#28678,#28679,#28680,
#28681,#28682,#28683,#28684,#28685,#28686,#28687,#28688,#28689,#28690,#28691,
#28692,#28693,#28694,#28695,#28696,#28697,#28698,#28699,#28700,#28701,#28702,
#28703,#28704,#28705,#28706,#28707,#28708,#28709,#28710,#28711,#28712,#28713,
#28714,#28715,#28716,#28717,#28718,#28719,#28720,#28721,#28722,#28723,#28724),
 .UNSPECIFIED.,.F.,.F.,(4,3,3,3,3,3,3,3,3,3,3,3,3,3,3,3,3,3,3,3,3,3,3,3,
3,3,3,3,3,3,3,3,3,3,3,3,3,3,3,3,3,3,3,3,3,3,3,3,3,3,3,3,3,3,3,3,3,3,3,3,
4),(0.0178660642413966,0.0181417588937503,0.0186938767206654,0.0187811248524612,
0.0189688428508114,0.0194531680236473,0.0199158046998442,0.0200716214602261,
0.0205298348659482,0.0210163068304557,0.0210454834309858,0.0211744000696409,
0.0219594418566194,0.0221678060338532,0.0222771786790556,0.0227260534193597,
0.0232822856052293,0.0233799572884703,0.0238115218795811,0.0239313465931777,
0.0242624070083197,0.0243886629871502,0.0244827358978851,0.0252848636807742,
0.025488188664657,0.0255855145072998,0.0260359693196439,0.0261369038120072,
0.0264718602397466,0.0265826145543591,0.0266882931167146,0.0271831282339348,
0.0276765624138436,0.0277910717261293,0.0280872868681377,0.0282242998156046,
0.0283424610308367,0.0287313424802207,0.0287733642636607,0.028893850335544,
0.0292158645122804,0.0294452396402514,0.0297215320002951,0.0298768660914162,
0.0299966289449587,0.0305825033289074,0.0309879174841298,0.0310994075543735,
0.0316285242822441,0.0321072673250968,0.0322021861637882,0.0327550977994062,
0.03323391559953,0.0333049647732029,0.0336759265167946,0.0338000533258756,
0.0338563540779102,0.0343681678909991,0.0344077433826176,0.0353007819162081,
0.0355105219920323),.UNSPECIFIED.);
#1819=B_SPLINE_CURVE_WITH_KNOTS('',3,(#28729,#28730,#28731,#28732,#28733,
#28734,#28735,#28736,#28737,#28738),.UNSPECIFIED.,.F.,.F.,(4,2,2,2,4),(-0.811230782792507,
-0.589543564549274,-0.405568456785375,-0.225516486965526,0.),
 .UNSPECIFIED.);
#1820=B_SPLINE_CURVE_WITH_KNOTS('',3,(#28740,#28741,#28742,#28743,#28744,
#28745,#28746,#28747,#28748,#28749,#28750,#28751,#28752,#28753,#28754,#28755),
 .UNSPECIFIED.,.F.,.F.,(4,2,2,2,2,2,2,4),(-1.61608002816124,-1.45775061305033,
-1.29955710501412,-1.0636537651015,-0.825767803590715,-0.617872986250325,
-0.355668197463001,0.),.UNSPECIFIED.);
#1821=B_SPLINE_CURVE_WITH_KNOTS('',3,(#28756,#28757,#28758,#28759,#28760,
#28761,#28762,#28763,#28764,#28765,#28766,#28767,#28768,#28769,#28770,#28771),
 .UNSPECIFIED.,.F.,.F.,(4,2,2,2,2,2,2,4),(-2.43104855078003,-1.903494016152,
-1.45644570848914,-1.09062827200157,-0.723808102624913,-0.376722226195001,
-0.186648168518802,0.),.UNSPECIFIED.);
#1822=B_SPLINE_CURVE_WITH_KNOTS('',3,(#31667,#31668,#31669,#31670,#31671,
#31672,#31673,#31674,#31675,#31676,#31677,#31678,#31679,#31680,#31681,#31682),
 .UNSPECIFIED.,.F.,.F.,(4,2,2,2,2,2,2,4),(0.,0.211383895657764,0.374142667531924,
0.583513224887238,0.779876212205008,0.988270595967209,1.21322647326508,
1.38005248901974),.UNSPECIFIED.);
#1823=B_SPLINE_CURVE_WITH_KNOTS('',3,(#37466,#37467,#37468,#37469,#37470,
#37471,#37472,#37473,#37474,#37475),.UNSPECIFIED.,.F.,.F.,(4,2,2,2,4),(0.,
0.220020771446265,0.376089701153298,0.530276196623649,0.752535026745683),
 .UNSPECIFIED.);
#1824=B_SPLINE_CURVE_WITH_KNOTS('',3,(#39422,#39423,#39424,#39425,#39426,
#39427,#39428,#39429,#39430,#39431,#39432,#39433,#39434,#39435,#39436,#39437),
 .UNSPECIFIED.,.F.,.F.,(4,2,2,2,2,2,2,4),(0.,0.371355913148883,0.741064833958748,
1.0486227715232,1.30223077148216,1.57308405581568,1.73972138317415,1.89659917227108),
 .UNSPECIFIED.);
#1958=LINE('',#28166,#2276);
#1959=LINE('',#28350,#2277);
#1960=LINE('',#28354,#2278);
#1961=LINE('',#28361,#2279);
#1962=LINE('',#28367,#2280);
#1963=LINE('',#28370,#2281);
#1964=LINE('',#28461,#2282);
#1965=LINE('',#39442,#2283);
#1966=LINE('',#39444,#2284);
#1967=LINE('',#39446,#2285);
#1968=LINE('',#39452,#2286);
#1969=LINE('',#39458,#2287);
#1970=LINE('',#39460,#2288);
#1971=LINE('',#39466,#2289);
#1972=LINE('',#39472,#2290);
#1973=LINE('',#39474,#2291);
#1974=LINE('',#39480,#2292);
#1975=LINE('',#39486,#2293);
#1976=LINE('',#39488,#2294);
#1977=LINE('',#39494,#2295);
#1978=LINE('',#39500,#2296);
#1979=LINE('',#39501,#2297);
#1980=LINE('',#39503,#2298);
#1981=LINE('',#39508,#2299);
#1982=LINE('',#39513,#2300);
#2276=VECTOR('',#7940,5.);
#2277=VECTOR('',#7949,7.4375);
#2278=VECTOR('',#7954,7.4375);
#2279=VECTOR('',#7961,11.7);
#2280=VECTOR('',#7968,7.70000000000001);
#2281=VECTOR('',#7973,12.7);
#2282=VECTOR('',#7974,12.7);
#2283=VECTOR('',#7987,1000.);
#2284=VECTOR('',#7988,1000.);
#2285=VECTOR('',#7989,1000.);
#2286=VECTOR('',#7990,1000.);
#2287=VECTOR('',#7993,1000.);
#2288=VECTOR('',#7994,1000.);
#2289=VECTOR('',#7995,1000.);
#2290=VECTOR('',#7998,1000.);
#2291=VECTOR('',#7999,1000.);
#2292=VECTOR('',#8000,1000.);
#2293=VECTOR('',#8003,1000.);
#2294=VECTOR('',#8004,1000.);
#2295=VECTOR('',#8005,1000.);
#2296=VECTOR('',#8008,1000.);
#2297=VECTOR('',#8009,1000.);
#2298=VECTOR('',#8010,1000.);
#2299=VECTOR('',#8013,1000.);
#2300=VECTOR('',#8014,1000.);
#2701=VERTEX_POINT('',#27292);
#2702=VERTEX_POINT('',#27293);
#2703=VERTEX_POINT('',#27466);
#2704=VERTEX_POINT('',#27468);
#2705=VERTEX_POINT('',#27551);
#2706=VERTEX_POINT('',#27572);
#2707=VERTEX_POINT('',#27704);
#2708=VERTEX_POINT('',#27705);
#2709=VERTEX_POINT('',#27791);
#2710=VERTEX_POINT('',#27793);
#2711=VERTEX_POINT('',#27987);
#2712=VERTEX_POINT('',#27989);
#2713=VERTEX_POINT('',#28077);
#2714=VERTEX_POINT('',#28078);
#2715=VERTEX_POINT('',#28080);
#2716=VERTEX_POINT('',#28088);
#2717=VERTEX_POINT('',#28165);
#2718=VERTEX_POINT('',#28345);
#2719=VERTEX_POINT('',#28346);
#2720=VERTEX_POINT('',#28349);
#2721=VERTEX_POINT('',#28353);
#2722=VERTEX_POINT('',#28356);
#2723=VERTEX_POINT('',#28357);
#2724=VERTEX_POINT('',#28360);
#2725=VERTEX_POINT('',#28364);
#2726=VERTEX_POINT('',#28366);
#2727=VERTEX_POINT('',#28371);
#2728=VERTEX_POINT('',#28460);
#2729=VERTEX_POINT('',#28542);
#2730=VERTEX_POINT('',#28727);
#2731=VERTEX_POINT('',#28728);
#2732=VERTEX_POINT('',#28739);
#2733=VERTEX_POINT('',#30718);
#2734=VERTEX_POINT('',#31666);
#2735=VERTEX_POINT('',#36520);
#2736=VERTEX_POINT('',#39440);
#2737=VERTEX_POINT('',#39441);
#2738=VERTEX_POINT('',#39443);
#2739=VERTEX_POINT('',#39445);
#2740=VERTEX_POINT('',#39447);
#2741=VERTEX_POINT('',#39451);
#2742=VERTEX_POINT('',#39457);
#2743=VERTEX_POINT('',#39459);
#2744=VERTEX_POINT('',#39461);
#2745=VERTEX_POINT('',#39465);
#2746=VERTEX_POINT('',#39471);
#2747=VERTEX_POINT('',#39473);
#2748=VERTEX_POINT('',#39475);
#2749=VERTEX_POINT('',#39479);
#2750=VERTEX_POINT('',#39485);
#2751=VERTEX_POINT('',#39487);
#2752=VERTEX_POINT('',#39489);
#2753=VERTEX_POINT('',#39493);
#2754=VERTEX_POINT('',#39499);
#2755=VERTEX_POINT('',#39502);
#2756=VERTEX_POINT('',#39509);
#3431=EDGE_CURVE('',#2701,#2702,#1806,.T.);
#3432=EDGE_CURVE('',#2701,#2703,#1447,.T.);
#3433=EDGE_CURVE('',#2704,#2703,#1807,.T.);
#3434=EDGE_CURVE('',#2705,#2704,#1808,.T.);
#3435=EDGE_CURVE('',#2706,#2705,#1448,.T.);
#3436=EDGE_CURVE('',#2702,#2706,#1809,.T.);
#3437=EDGE_CURVE('',#2707,#2708,#1810,.T.);
#3438=EDGE_CURVE('',#2707,#2709,#1449,.T.);
#3439=EDGE_CURVE('',#2710,#2709,#1811,.T.);
#3440=EDGE_CURVE('',#2711,#2710,#1450,.T.);
#3441=EDGE_CURVE('',#2712,#2711,#1451,.T.);
#3442=EDGE_CURVE('',#2708,#2712,#1812,.T.);
#3443=EDGE_CURVE('',#2713,#2714,#1452,.T.);
#3444=EDGE_CURVE('',#2713,#2715,#198,.T.);
#3445=EDGE_CURVE('',#2715,#2714,#199,.T.);
#3446=EDGE_CURVE('',#2716,#2707,#1813,.T.);
#3447=EDGE_CURVE('',#2708,#2717,#1958,.T.);
#3448=EDGE_CURVE('',#2717,#2701,#462,.T.);
#3449=EDGE_CURVE('',#2706,#2717,#1814,.T.);
#3450=EDGE_CURVE('',#2712,#2716,#1815,.T.);
#3451=EDGE_CURVE('',#2718,#2719,#1453,.T.);
#3452=EDGE_CURVE('',#2719,#2718,#1454,.T.);
#3453=EDGE_CURVE('',#2719,#2720,#1959,.T.);
#3454=EDGE_CURVE('',#2720,#2720,#1455,.T.);
#3455=EDGE_CURVE('',#2718,#2721,#1960,.T.);
#3456=EDGE_CURVE('',#2722,#2723,#1456,.T.);
#3457=EDGE_CURVE('',#2723,#2722,#1457,.T.);
#3458=EDGE_CURVE('',#2723,#2724,#1961,.T.);
#3459=EDGE_CURVE('',#2724,#2724,#1458,.T.);
#3460=EDGE_CURVE('',#2725,#2725,#1459,.T.);
#3461=EDGE_CURVE('',#2725,#2726,#1962,.T.);
#3462=EDGE_CURVE('',#2726,#2726,#1460,.T.);
#3463=EDGE_CURVE('',#2722,#2704,#1963,.T.);
#3464=EDGE_CURVE('',#2703,#2727,#1816,.T.);
#3465=EDGE_CURVE('',#2727,#2728,#1964,.T.);
#3466=EDGE_CURVE('',#2728,#2728,#1461,.T.);
#3467=EDGE_CURVE('',#2727,#2705,#1817,.T.);
#3468=EDGE_CURVE('',#2709,#2729,#1462,.T.);
#3469=EDGE_CURVE('',#2729,#2711,#1818,.T.);
#3470=EDGE_CURVE('',#2730,#2731,#1819,.T.);
#3471=EDGE_CURVE('',#2731,#2732,#1820,.T.);
#3472=EDGE_CURVE('',#2732,#2730,#1821,.T.);
#3473=EDGE_CURVE('',#2733,#2731,#200,.T.);
#3474=EDGE_CURVE('',#2733,#2734,#1822,.T.);
#3475=EDGE_CURVE('',#2734,#2732,#201,.T.);
#3476=EDGE_CURVE('',#2735,#2730,#202,.T.);
#3477=EDGE_CURVE('',#2735,#2733,#1823,.T.);
#3478=EDGE_CURVE('',#2734,#2735,#1824,.T.);
#3479=EDGE_CURVE('',#2736,#2737,#1965,.T.);
#3480=EDGE_CURVE('',#2736,#2738,#1966,.T.);
#3481=EDGE_CURVE('',#2738,#2739,#1967,.T.);
#3482=EDGE_CURVE('',#2740,#2739,#203,.T.);
#3483=EDGE_CURVE('',#2741,#2740,#1968,.T.);
#3484=EDGE_CURVE('',#2737,#2741,#204,.T.);
#3485=EDGE_CURVE('',#2738,#2742,#1969,.T.);
#3486=EDGE_CURVE('',#2742,#2743,#1970,.T.);
#3487=EDGE_CURVE('',#2744,#2743,#205,.T.);
#3488=EDGE_CURVE('',#2745,#2744,#1971,.T.);
#3489=EDGE_CURVE('',#2739,#2745,#206,.T.);
#3490=EDGE_CURVE('',#2742,#2746,#1972,.T.);
#3491=EDGE_CURVE('',#2746,#2747,#1973,.T.);
#3492=EDGE_CURVE('',#2748,#2747,#207,.T.);
#3493=EDGE_CURVE('',#2749,#2748,#1974,.T.);
#3494=EDGE_CURVE('',#2743,#2749,#208,.T.);
#3495=EDGE_CURVE('',#2746,#2750,#1975,.T.);
#3496=EDGE_CURVE('',#2750,#2751,#1976,.T.);
#3497=EDGE_CURVE('',#2752,#2751,#209,.T.);
#3498=EDGE_CURVE('',#2753,#2752,#1977,.T.);
#3499=EDGE_CURVE('',#2747,#2753,#210,.T.);
#3500=EDGE_CURVE('',#2750,#2754,#1978,.T.);
#3501=EDGE_CURVE('',#2754,#2715,#1979,.T.);
#3502=EDGE_CURVE('',#2755,#2713,#1980,.T.);
#3503=EDGE_CURVE('',#2751,#2755,#211,.T.);
#3504=EDGE_CURVE('',#2754,#2736,#1981,.T.);
#3505=EDGE_CURVE('',#2756,#2737,#212,.T.);
#3506=EDGE_CURVE('',#2714,#2756,#1982,.T.);
#3507=EDGE_CURVE('',#2756,#2741,#1463,.T.);
#3508=EDGE_CURVE('',#2752,#2755,#1464,.T.);
#3509=EDGE_CURVE('',#2748,#2753,#1465,.T.);
#3510=EDGE_CURVE('',#2744,#2749,#1466,.T.);
#3511=EDGE_CURVE('',#2740,#2745,#1467,.T.);
#4758=ORIENTED_EDGE('',*,*,#3431,.F.);
#4759=ORIENTED_EDGE('',*,*,#3432,.T.);
#4760=ORIENTED_EDGE('',*,*,#3433,.F.);
#4761=ORIENTED_EDGE('',*,*,#3434,.F.);
#4762=ORIENTED_EDGE('',*,*,#3435,.F.);
#4763=ORIENTED_EDGE('',*,*,#3436,.F.);
#4764=ORIENTED_EDGE('',*,*,#3437,.F.);
#4765=ORIENTED_EDGE('',*,*,#3438,.T.);
#4766=ORIENTED_EDGE('',*,*,#3439,.F.);
#4767=ORIENTED_EDGE('',*,*,#3440,.F.);
#4768=ORIENTED_EDGE('',*,*,#3441,.F.);
#4769=ORIENTED_EDGE('',*,*,#3442,.F.);
#4770=ORIENTED_EDGE('',*,*,#3443,.F.);
#4771=ORIENTED_EDGE('',*,*,#3444,.T.);
#4772=ORIENTED_EDGE('',*,*,#3445,.T.);
#4773=ORIENTED_EDGE('',*,*,#3446,.T.);
#4774=ORIENTED_EDGE('',*,*,#3437,.T.);
#4775=ORIENTED_EDGE('',*,*,#3447,.T.);
#4776=ORIENTED_EDGE('',*,*,#3448,.T.);
#4777=ORIENTED_EDGE('',*,*,#3431,.T.);
#4778=ORIENTED_EDGE('',*,*,#3436,.T.);
#4779=ORIENTED_EDGE('',*,*,#3449,.T.);
#4780=ORIENTED_EDGE('',*,*,#3447,.F.);
#4781=ORIENTED_EDGE('',*,*,#3442,.T.);
#4782=ORIENTED_EDGE('',*,*,#3450,.T.);
#4783=ORIENTED_EDGE('',*,*,#3451,.F.);
#4784=ORIENTED_EDGE('',*,*,#3452,.F.);
#4785=ORIENTED_EDGE('',*,*,#3453,.T.);
#4786=ORIENTED_EDGE('',*,*,#3454,.T.);
#4787=ORIENTED_EDGE('',*,*,#3453,.F.);
#4788=ORIENTED_EDGE('',*,*,#3451,.T.);
#4789=ORIENTED_EDGE('',*,*,#3452,.T.);
#4790=ORIENTED_EDGE('',*,*,#3455,.T.);
#4791=ORIENTED_EDGE('',*,*,#3455,.F.);
#4792=ORIENTED_EDGE('',*,*,#3456,.F.);
#4793=ORIENTED_EDGE('',*,*,#3457,.F.);
#4794=ORIENTED_EDGE('',*,*,#3458,.T.);
#4795=ORIENTED_EDGE('',*,*,#3459,.F.);
#4796=ORIENTED_EDGE('',*,*,#3458,.F.);
#4797=ORIENTED_EDGE('',*,*,#3460,.F.);
#4798=ORIENTED_EDGE('',*,*,#3461,.T.);
#4799=ORIENTED_EDGE('',*,*,#3462,.T.);
#4800=ORIENTED_EDGE('',*,*,#3461,.F.);
#4801=ORIENTED_EDGE('',*,*,#3456,.T.);
#4802=ORIENTED_EDGE('',*,*,#3457,.T.);
#4803=ORIENTED_EDGE('',*,*,#3463,.T.);
#4804=ORIENTED_EDGE('',*,*,#3433,.T.);
#4805=ORIENTED_EDGE('',*,*,#3464,.T.);
#4806=ORIENTED_EDGE('',*,*,#3465,.T.);
#4807=ORIENTED_EDGE('',*,*,#3466,.F.);
#4808=ORIENTED_EDGE('',*,*,#3465,.F.);
#4809=ORIENTED_EDGE('',*,*,#3467,.T.);
#4810=ORIENTED_EDGE('',*,*,#3434,.T.);
#4811=ORIENTED_EDGE('',*,*,#3463,.F.);
#4812=ORIENTED_EDGE('',*,*,#3439,.T.);
#4813=ORIENTED_EDGE('',*,*,#3468,.T.);
#4814=ORIENTED_EDGE('',*,*,#3469,.T.);
#4815=ORIENTED_EDGE('',*,*,#3440,.T.);
#4816=ORIENTED_EDGE('',*,*,#3459,.T.);
#4817=ORIENTED_EDGE('',*,*,#3462,.F.);
#4818=ORIENTED_EDGE('',*,*,#3470,.T.);
#4819=ORIENTED_EDGE('',*,*,#3471,.T.);
#4820=ORIENTED_EDGE('',*,*,#3472,.T.);
#4821=ORIENTED_EDGE('',*,*,#3460,.T.);
#4822=ORIENTED_EDGE('',*,*,#3473,.F.);
#4823=ORIENTED_EDGE('',*,*,#3474,.T.);
#4824=ORIENTED_EDGE('',*,*,#3475,.T.);
#4825=ORIENTED_EDGE('',*,*,#3471,.F.);
#4826=ORIENTED_EDGE('',*,*,#3476,.F.);
#4827=ORIENTED_EDGE('',*,*,#3477,.T.);
#4828=ORIENTED_EDGE('',*,*,#3473,.T.);
#4829=ORIENTED_EDGE('',*,*,#3470,.F.);
#4830=ORIENTED_EDGE('',*,*,#3475,.F.);
#4831=ORIENTED_EDGE('',*,*,#3478,.T.);
#4832=ORIENTED_EDGE('',*,*,#3476,.T.);
#4833=ORIENTED_EDGE('',*,*,#3472,.F.);
#4834=ORIENTED_EDGE('',*,*,#3478,.F.);
#4835=ORIENTED_EDGE('',*,*,#3474,.F.);
#4836=ORIENTED_EDGE('',*,*,#3477,.F.);
#4837=ORIENTED_EDGE('',*,*,#3454,.F.);
#4838=ORIENTED_EDGE('',*,*,#3479,.F.);
#4839=ORIENTED_EDGE('',*,*,#3480,.T.);
#4840=ORIENTED_EDGE('',*,*,#3481,.T.);
#4841=ORIENTED_EDGE('',*,*,#3482,.F.);
#4842=ORIENTED_EDGE('',*,*,#3483,.F.);
#4843=ORIENTED_EDGE('',*,*,#3484,.F.);
#4844=ORIENTED_EDGE('',*,*,#3481,.F.);
#4845=ORIENTED_EDGE('',*,*,#3485,.T.);
#4846=ORIENTED_EDGE('',*,*,#3486,.T.);
#4847=ORIENTED_EDGE('',*,*,#3487,.F.);
#4848=ORIENTED_EDGE('',*,*,#3488,.F.);
#4849=ORIENTED_EDGE('',*,*,#3489,.F.);
#4850=ORIENTED_EDGE('',*,*,#3486,.F.);
#4851=ORIENTED_EDGE('',*,*,#3490,.T.);
#4852=ORIENTED_EDGE('',*,*,#3491,.T.);
#4853=ORIENTED_EDGE('',*,*,#3492,.F.);
#4854=ORIENTED_EDGE('',*,*,#3493,.F.);
#4855=ORIENTED_EDGE('',*,*,#3494,.F.);
#4856=ORIENTED_EDGE('',*,*,#3491,.F.);
#4857=ORIENTED_EDGE('',*,*,#3495,.T.);
#4858=ORIENTED_EDGE('',*,*,#3496,.T.);
#4859=ORIENTED_EDGE('',*,*,#3497,.F.);
#4860=ORIENTED_EDGE('',*,*,#3498,.F.);
#4861=ORIENTED_EDGE('',*,*,#3499,.F.);
#4862=ORIENTED_EDGE('',*,*,#3496,.F.);
#4863=ORIENTED_EDGE('',*,*,#3500,.T.);
#4864=ORIENTED_EDGE('',*,*,#3501,.T.);
#4865=ORIENTED_EDGE('',*,*,#3444,.F.);
#4866=ORIENTED_EDGE('',*,*,#3502,.F.);
#4867=ORIENTED_EDGE('',*,*,#3503,.F.);
#4868=ORIENTED_EDGE('',*,*,#3501,.F.);
#4869=ORIENTED_EDGE('',*,*,#3504,.T.);
#4870=ORIENTED_EDGE('',*,*,#3479,.T.);
#4871=ORIENTED_EDGE('',*,*,#3505,.F.);
#4872=ORIENTED_EDGE('',*,*,#3506,.F.);
#4873=ORIENTED_EDGE('',*,*,#3445,.F.);
#4874=ORIENTED_EDGE('',*,*,#3466,.T.);
#4875=ORIENTED_EDGE('',*,*,#3480,.F.);
#4876=ORIENTED_EDGE('',*,*,#3504,.F.);
#4877=ORIENTED_EDGE('',*,*,#3500,.F.);
#4878=ORIENTED_EDGE('',*,*,#3495,.F.);
#4879=ORIENTED_EDGE('',*,*,#3490,.F.);
#4880=ORIENTED_EDGE('',*,*,#3485,.F.);
#4881=ORIENTED_EDGE('',*,*,#3505,.T.);
#4882=ORIENTED_EDGE('',*,*,#3484,.T.);
#4883=ORIENTED_EDGE('',*,*,#3507,.F.);
#4884=ORIENTED_EDGE('',*,*,#3508,.F.);
#4885=ORIENTED_EDGE('',*,*,#3497,.T.);
#4886=ORIENTED_EDGE('',*,*,#3503,.T.);
#4887=ORIENTED_EDGE('',*,*,#3509,.F.);
#4888=ORIENTED_EDGE('',*,*,#3492,.T.);
#4889=ORIENTED_EDGE('',*,*,#3499,.T.);
#4890=ORIENTED_EDGE('',*,*,#3510,.F.);
#4891=ORIENTED_EDGE('',*,*,#3487,.T.);
#4892=ORIENTED_EDGE('',*,*,#3494,.T.);
#4893=ORIENTED_EDGE('',*,*,#3511,.F.);
#4894=ORIENTED_EDGE('',*,*,#3482,.T.);
#4895=ORIENTED_EDGE('',*,*,#3489,.T.);
#4896=ORIENTED_EDGE('',*,*,#3483,.T.);
#4897=ORIENTED_EDGE('',*,*,#3511,.T.);
#4898=ORIENTED_EDGE('',*,*,#3488,.T.);
#4899=ORIENTED_EDGE('',*,*,#3510,.T.);
#4900=ORIENTED_EDGE('',*,*,#3493,.T.);
#4901=ORIENTED_EDGE('',*,*,#3509,.T.);
#4902=ORIENTED_EDGE('',*,*,#3498,.T.);
#4903=ORIENTED_EDGE('',*,*,#3508,.T.);
#4904=ORIENTED_EDGE('',*,*,#3502,.T.);
#4905=ORIENTED_EDGE('',*,*,#3443,.T.);
#4906=ORIENTED_EDGE('',*,*,#3506,.T.);
#4907=ORIENTED_EDGE('',*,*,#3507,.T.);
#4908=ORIENTED_EDGE('',*,*,#3438,.F.);
#4909=ORIENTED_EDGE('',*,*,#3446,.F.);
#4910=ORIENTED_EDGE('',*,*,#3450,.F.);
#4911=ORIENTED_EDGE('',*,*,#3441,.T.);
#4912=ORIENTED_EDGE('',*,*,#3469,.F.);
#4913=ORIENTED_EDGE('',*,*,#3468,.F.);
#4914=ORIENTED_EDGE('',*,*,#3432,.F.);
#4915=ORIENTED_EDGE('',*,*,#3448,.F.);
#4916=ORIENTED_EDGE('',*,*,#3449,.F.);
#4917=ORIENTED_EDGE('',*,*,#3435,.T.);
#4918=ORIENTED_EDGE('',*,*,#3467,.F.);
#4919=ORIENTED_EDGE('',*,*,#3464,.F.);
#5862=CYLINDRICAL_SURFACE('',#6706,5.);
#5863=CYLINDRICAL_SURFACE('',#6708,7.4375);
#5864=CYLINDRICAL_SURFACE('',#6717,7.70000000000001);
#5865=CYLINDRICAL_SURFACE('',#6720,12.7);
#6089=ADVANCED_FACE('',(#674),#176,.T.);
#6090=ADVANCED_FACE('',(#675),#177,.T.);
#6091=ADVANCED_FACE('',(#676),#377,.T.);
#6092=ADVANCED_FACE('',(#677),#5862,.F.);
#6093=ADVANCED_FACE('',(#678),#5863,.T.);
#6094=ADVANCED_FACE('',(#679),#378,.T.);
#6095=ADVANCED_FACE('',(#680),#379,.T.);
#6096=ADVANCED_FACE('',(#681),#5864,.T.);
#6097=ADVANCED_FACE('',(#682,#346),#5865,.T.);
#6098=ADVANCED_FACE('',(#683,#347),#277,.F.);
#6099=ADVANCED_FACE('',(#684,#348),#278,.F.);
#6100=ADVANCED_FACE('',(#685),#178,.F.);
#6101=ADVANCED_FACE('',(#686),#179,.F.);
#6102=ADVANCED_FACE('',(#687),#180,.F.);
#6103=ADVANCED_FACE('',(#688,#349),#279,.F.);
#6104=ADVANCED_FACE('',(#689),#280,.T.);
#6105=ADVANCED_FACE('',(#690),#281,.T.);
#6106=ADVANCED_FACE('',(#691),#282,.T.);
#6107=ADVANCED_FACE('',(#692),#283,.T.);
#6108=ADVANCED_FACE('',(#693),#284,.T.);
#6109=ADVANCED_FACE('',(#694),#285,.T.);
#6110=ADVANCED_FACE('',(#695,#350),#286,.T.);
#6111=ADVANCED_FACE('',(#696),#380,.T.);
#6112=ADVANCED_FACE('',(#697),#381,.T.);
#6113=ADVANCED_FACE('',(#698),#382,.T.);
#6114=ADVANCED_FACE('',(#699),#383,.T.);
#6115=ADVANCED_FACE('',(#700),#384,.T.);
#6116=ADVANCED_FACE('',(#701),#287,.F.);
#6117=ADVANCED_FACE('',(#702),#181,.T.);
#6118=ADVANCED_FACE('',(#703),#182,.T.);
#6299=CLOSED_SHELL('',(#6089,#6090,#6091,#6092,#6093,#6094,#6095,#6096,
#6097,#6098,#6099,#6100,#6101,#6102,#6103,#6104,#6105,#6106,#6107,#6108,
#6109,#6110,#6111,#6112,#6113,#6114,#6115,#6116,#6117,#6118));
#6698=AXIS2_PLACEMENT_3D('',#27165,#7922,#7923);
#6699=AXIS2_PLACEMENT_3D('',#27467,#7924,#7925);
#6700=AXIS2_PLACEMENT_3D('',#27573,#7926,#7927);
#6701=AXIS2_PLACEMENT_3D('',#27792,#7928,#7929);
#6702=AXIS2_PLACEMENT_3D('',#27988,#7930,#7931);
#6703=AXIS2_PLACEMENT_3D('',#27990,#7932,#7933);
#6704=AXIS2_PLACEMENT_3D('',#28076,#7934,#7935);
#6705=AXIS2_PLACEMENT_3D('',#28079,#7936,#7937);
#6706=AXIS2_PLACEMENT_3D('',#28087,#7938,#7939);
#6707=AXIS2_PLACEMENT_3D('',#28167,#7941,#7942);
#6708=AXIS2_PLACEMENT_3D('',#28344,#7943,#7944);
#6709=AXIS2_PLACEMENT_3D('',#28347,#7945,#7946);
#6710=AXIS2_PLACEMENT_3D('',#28348,#7947,#7948);
#6711=AXIS2_PLACEMENT_3D('',#28351,#7950,#7951);
#6712=AXIS2_PLACEMENT_3D('',#28352,#7952,#7953);
#6713=AXIS2_PLACEMENT_3D('',#28355,#7955,#7956);
#6714=AXIS2_PLACEMENT_3D('',#28358,#7957,#7958);
#6715=AXIS2_PLACEMENT_3D('',#28359,#7959,#7960);
#6716=AXIS2_PLACEMENT_3D('',#28362,#7962,#7963);
#6717=AXIS2_PLACEMENT_3D('',#28363,#7964,#7965);
#6718=AXIS2_PLACEMENT_3D('',#28365,#7966,#7967);
#6719=AXIS2_PLACEMENT_3D('',#28368,#7969,#7970);
#6720=AXIS2_PLACEMENT_3D('',#28369,#7971,#7972);
#6721=AXIS2_PLACEMENT_3D('',#28462,#7975,#7976);
#6722=AXIS2_PLACEMENT_3D('',#28543,#7977,#7978);
#6723=AXIS2_PLACEMENT_3D('',#28725,#7979,#7980);
#6724=AXIS2_PLACEMENT_3D('',#28726,#7981,#7982);
#6725=AXIS2_PLACEMENT_3D('',#39438,#7983,#7984);
#6726=AXIS2_PLACEMENT_3D('',#39439,#7985,#7986);
#6727=AXIS2_PLACEMENT_3D('',#39456,#7991,#7992);
#6728=AXIS2_PLACEMENT_3D('',#39470,#7996,#7997);
#6729=AXIS2_PLACEMENT_3D('',#39484,#8001,#8002);
#6730=AXIS2_PLACEMENT_3D('',#39498,#8006,#8007);
#6731=AXIS2_PLACEMENT_3D('',#39507,#8011,#8012);
#6732=AXIS2_PLACEMENT_3D('',#39514,#8015,#8016);
#6733=AXIS2_PLACEMENT_3D('',#39515,#8017,#8018);
#6734=AXIS2_PLACEMENT_3D('',#39516,#8019,#8020);
#6735=AXIS2_PLACEMENT_3D('',#39517,#8021,#8022);
#6736=AXIS2_PLACEMENT_3D('',#39518,#8023,#8024);
#6737=AXIS2_PLACEMENT_3D('',#39519,#8025,#8026);
#6738=AXIS2_PLACEMENT_3D('',#39520,#8027,#8028);
#6739=AXIS2_PLACEMENT_3D('',#39521,#8029,#8030);
#6740=AXIS2_PLACEMENT_3D('',#39522,#8031,#8032);
#6741=AXIS2_PLACEMENT_3D('',#39523,#8033,#8034);
#6742=AXIS2_PLACEMENT_3D('',#39524,#8035,#8036);
#6743=AXIS2_PLACEMENT_3D('',#39525,#8037,#8038);
#7922=DIRECTION('axis',(0.,0.,1.));
#7923=DIRECTION('refdir',(1.,0.,0.));
#7924=DIRECTION('center_axis',(0.010041653963972,-0.999936721719416,0.00507126637988255));
#7925=DIRECTION('ref_axis',(0.999949580025092,0.010041783090799,-1.60007301981504E-17));
#7926=DIRECTION('center_axis',(-0.00891671946192249,0.999950105367358,0.0045032088389469));
#7927=DIRECTION('ref_axis',(-0.999960244460585,-0.00891680987388346,-1.13603182561227E-17));
#7928=DIRECTION('center_axis',(-0.999091404712184,0.0388570551898569,0.0175069783860113));
#7929=DIRECTION('ref_axis',(-0.0388630112918391,-0.999244547822669,2.07434801815803E-18));
#7930=DIRECTION('center_axis',(-1.61571391014197E-6,0.424667837114185,0.90534922992078));
#7931=DIRECTION('ref_axis',(1.42145081289922E-6,0.905349229922022,-0.424667837112231));
#7932=DIRECTION('center_axis',(0.999152984554678,-0.0375175097387351,0.0169041390932047));
#7933=DIRECTION('ref_axis',(0.0375228712004652,0.999295769097855,-1.81623557326339E-18));
#7934=DIRECTION('center_axis',(0.,-1.,0.));
#7935=DIRECTION('ref_axis',(0.,0.,-1.));
#7936=DIRECTION('center_axis',(0.,1.,0.));
#7937=DIRECTION('ref_axis',(0.,0.,-1.));
#7938=DIRECTION('center_axis',(0.,0.,1.));
#7939=DIRECTION('ref_axis',(1.,0.,0.));
#7940=DIRECTION('',(0.,0.,1.));
#7941=DIRECTION('center_axis',(-0.489387119106713,-5.09160744540987E-5,
0.872066651730236));
#7942=DIRECTION('ref_axis',(-0.106617366365419,-0.992494824264684,-0.0598895733589422));
#7943=DIRECTION('center_axis',(0.,-1.,0.));
#7944=DIRECTION('ref_axis',(0.,0.,-1.));
#7945=DIRECTION('center_axis',(0.,-1.,0.));
#7946=DIRECTION('ref_axis',(0.,0.,-1.));
#7947=DIRECTION('center_axis',(0.,-1.,0.));
#7948=DIRECTION('ref_axis',(0.,0.,-1.));
#7949=DIRECTION('',(0.,1.,0.));
#7950=DIRECTION('center_axis',(0.,-1.,0.));
#7951=DIRECTION('ref_axis',(0.,0.,-1.));
#7952=DIRECTION('center_axis',(0.,1.,0.));
#7953=DIRECTION('ref_axis',(0.,0.,1.));
#7954=DIRECTION('',(8.65956056235489E-17,-0.707106781186551,0.707106781186544));
#7955=DIRECTION('center_axis',(0.,1.,0.));
#7956=DIRECTION('ref_axis',(0.,0.,1.));
#7957=DIRECTION('center_axis',(0.,1.,0.));
#7958=DIRECTION('ref_axis',(0.,0.,1.));
#7959=DIRECTION('center_axis',(0.,1.,0.));
#7960=DIRECTION('ref_axis',(0.,0.,1.));
#7961=DIRECTION('',(8.65956056235486E-17,-0.707106781186554,0.707106781186541));
#7962=DIRECTION('center_axis',(0.,-1.,0.));
#7963=DIRECTION('ref_axis',(0.,0.,1.));
#7964=DIRECTION('center_axis',(0.,-1.,0.));
#7965=DIRECTION('ref_axis',(0.,0.,-1.));
#7966=DIRECTION('center_axis',(0.,-1.,0.));
#7967=DIRECTION('ref_axis',(0.,0.,-1.));
#7968=DIRECTION('',(0.,1.,0.));
#7969=DIRECTION('center_axis',(0.,-1.,0.));
#7970=DIRECTION('ref_axis',(0.,0.,-1.));
#7971=DIRECTION('center_axis',(0.,-1.,0.));
#7972=DIRECTION('ref_axis',(0.,0.,-1.));
#7973=DIRECTION('',(0.,1.,0.));
#7974=DIRECTION('',(0.,1.,0.));
#7975=DIRECTION('center_axis',(0.,1.,0.));
#7976=DIRECTION('ref_axis',(0.,0.,1.));
#7977=DIRECTION('center_axis',(-6.90968518692092E-5,-0.425975505302661,
0.904734692662865));
#7978=DIRECTION('ref_axis',(0.000745635165897718,-0.904734465265813,-0.425975341291467));
#7979=DIRECTION('center_axis',(0.,1.,0.));
#7980=DIRECTION('ref_axis',(0.,0.,1.));
#7981=DIRECTION('center_axis',(0.,-1.,0.));
#7982=DIRECTION('ref_axis',(0.,0.,-1.));
#7983=DIRECTION('center_axis',(0.,1.,0.));
#7984=DIRECTION('ref_axis',(0.,0.,1.));
#7985=DIRECTION('center_axis',(-1.,0.,-2.76472863796254E-16));
#7986=DIRECTION('ref_axis',(-2.76472863796254E-16,0.,1.));
#7987=DIRECTION('',(0.,1.,0.));
#7988=DIRECTION('',(-2.76472863796254E-16,0.,1.));
#7989=DIRECTION('',(0.,1.,0.));
#7990=DIRECTION('',(-2.76472863796254E-16,0.,1.));
#7991=DIRECTION('center_axis',(-0.5,0.,0.866025403784438));
#7992=DIRECTION('ref_axis',(0.866025403784438,0.,0.5));
#7993=DIRECTION('',(0.866025403784438,0.,0.5));
#7994=DIRECTION('',(0.,1.,0.));
#7995=DIRECTION('',(0.866025403784438,0.,0.5));
#7996=DIRECTION('center_axis',(0.5,0.,0.866025403784439));
#7997=DIRECTION('ref_axis',(0.866025403784439,0.,-0.5));
#7998=DIRECTION('',(0.866025403784439,0.,-0.5));
#7999=DIRECTION('',(0.,1.,0.));
#8000=DIRECTION('',(0.866025403784439,0.,-0.5));
#8001=DIRECTION('center_axis',(1.,0.,0.));
#8002=DIRECTION('ref_axis',(0.,0.,-1.));
#8003=DIRECTION('',(0.,0.,-1.));
#8004=DIRECTION('',(0.,1.,0.));
#8005=DIRECTION('',(0.,0.,-1.));
#8006=DIRECTION('center_axis',(0.5,0.,-0.866025403784439));
#8007=DIRECTION('ref_axis',(-0.866025403784439,0.,-0.5));
#8008=DIRECTION('',(-0.866025403784438,0.,-0.5));
#8009=DIRECTION('',(0.,1.,0.));
#8010=DIRECTION('',(-0.866025403784438,0.,-0.5));
#8011=DIRECTION('center_axis',(-0.5,0.,-0.866025403784439));
#8012=DIRECTION('ref_axis',(-0.866025403784439,0.,0.5));
#8013=DIRECTION('',(-0.866025403784439,0.,0.5));
#8014=DIRECTION('',(-0.866025403784439,0.,0.5));
#8015=DIRECTION('center_axis',(0.,1.,0.));
#8016=DIRECTION('ref_axis',(0.,0.,1.));
#8017=DIRECTION('center_axis',(0.,-1.,0.));
#8018=DIRECTION('ref_axis',(0.,0.,-1.));
#8019=DIRECTION('center_axis',(0.,1.,0.));
#8020=DIRECTION('ref_axis',(0.,0.,-1.));
#8021=DIRECTION('center_axis',(0.,-1.,0.));
#8022=DIRECTION('ref_axis',(0.,0.,-1.));
#8023=DIRECTION('center_axis',(0.,1.,0.));
#8024=DIRECTION('ref_axis',(7.105427357601E-15,0.,-1.));
#8025=DIRECTION('center_axis',(0.,-1.,0.));
#8026=DIRECTION('ref_axis',(0.,0.,-1.));
#8027=DIRECTION('center_axis',(0.,1.,0.));
#8028=DIRECTION('ref_axis',(3.5527136788005E-15,0.,-1.));
#8029=DIRECTION('center_axis',(0.,-1.,0.));
#8030=DIRECTION('ref_axis',(1.22464679914735E-16,0.,1.));
#8031=DIRECTION('center_axis',(0.,1.,0.));
#8032=DIRECTION('ref_axis',(5.32907051820075E-15,0.,-1.));
#8033=DIRECTION('center_axis',(0.,-1.,0.));
#8034=DIRECTION('ref_axis',(0.,0.,-1.));
#8035=DIRECTION('center_axis',(0.,1.,0.));
#8036=DIRECTION('ref_axis',(-8.88178419700125E-16,0.,-1.));
#8037=DIRECTION('center_axis',(0.,-1.,0.));
#8038=DIRECTION('ref_axis',(0.,0.,-1.));
#27165=CARTESIAN_POINT('',(0.,0.,0.));
#27166=CARTESIAN_POINT('Ctrl Pts',(4.99864419322373,-21.608305818412,10.8906322767302));
#27167=CARTESIAN_POINT('Ctrl Pts',(4.99883364334396,-21.6179081044763,11.7031708025873));
#27168=CARTESIAN_POINT('Ctrl Pts',(5.72391665153499,-21.5966350540385,11.3369690930511));
#27169=CARTESIAN_POINT('Ctrl Pts',(5.00698491717006,-21.9683819493214,10.8859593746152));
#27170=CARTESIAN_POINT('Ctrl Pts',(5.00568014694611,-21.9487593964398,11.700455499203));
#27171=CARTESIAN_POINT('Ctrl Pts',(5.73346753777204,-21.9927228607166,11.3321045753797));
#27172=CARTESIAN_POINT('Ctrl Pts',(4.97681790987538,-22.3214319362742,10.903022409287));
#27173=CARTESIAN_POINT('Ctrl Pts',(4.98154299652122,-22.2686534039265,11.7100742339915));
#27174=CARTESIAN_POINT('Ctrl Pts',(5.69892353458948,-22.3810823369386,11.3498673084045));
#27175=CARTESIAN_POINT('Ctrl Pts',(4.84821686874648,-22.9911597054847,10.9728701997679));
#27176=CARTESIAN_POINT('Ctrl Pts',(4.87172013085809,-22.8940685954447,11.7530513658957));
#27177=CARTESIAN_POINT('Ctrl Pts',(5.55166363360174,-23.1177906197389,11.4225792046101));
#27178=CARTESIAN_POINT('Ctrl Pts',(4.75280187594809,-23.3116970781571,11.0240130526473));
#27179=CARTESIAN_POINT('Ctrl Pts',(4.79059840005532,-23.1963542824898,11.7847242777248));
#27180=CARTESIAN_POINT('Ctrl Pts',(5.44240468437886,-23.4703854977074,11.4758191935635));
#27181=CARTESIAN_POINT('Ctrl Pts',(4.50592320341294,-23.9166636689606,11.1487513379524));
#27182=CARTESIAN_POINT('Ctrl Pts',(4.56891533871215,-23.784060286346,11.868052837188));
#27183=CARTESIAN_POINT('Ctrl Pts',(5.15970603065283,-24.1358555142914,11.605672265421));
#27184=CARTESIAN_POINT('Ctrl Pts',(4.35465771842323,-24.2035260698023,11.2222713469962));
#27185=CARTESIAN_POINT('Ctrl Pts',(4.43153279702055,-24.0685058089498,11.9186637657369));
#27186=CARTESIAN_POINT('Ctrl Pts',(4.98649309301282,-24.4514073295638,11.6822068961658));
#27187=CARTESIAN_POINT('Ctrl Pts',(3.99621871821646,-24.747643148554,11.3824972363738));
#27188=CARTESIAN_POINT('Ctrl Pts',(4.09216913012772,-24.6194703396761,12.0353086028313));
#27189=CARTESIAN_POINT('Ctrl Pts',(4.57604742933995,-25.0499419971568,11.8490025577107));
#27190=CARTESIAN_POINT('Ctrl Pts',(3.79223436493213,-24.9994962931869,11.4676424780953));
#27191=CARTESIAN_POINT('Ctrl Pts',(3.89587775698716,-24.880259680682,12.0995329053305));
#27192=CARTESIAN_POINT('Ctrl Pts',(4.34246643061078,-25.3269830936796,11.9376389892933));
#27193=CARTESIAN_POINT('Ctrl Pts',(3.45427885759424,-25.3435355466136,11.593909463285));
#27194=CARTESIAN_POINT('Ctrl Pts',(3.5593346006441,-25.2431905195649,12.1987939611122));
#27195=CARTESIAN_POINT('Ctrl Pts',(3.95547616613724,-25.7054297215759,12.0690831535375));
#27196=CARTESIAN_POINT('Ctrl Pts',(3.33602937785994,-25.4528825858882,11.6358715221986));
#27197=CARTESIAN_POINT('Ctrl Pts',(3.44182785331483,-25.35834649947,12.2319414526239));
#27198=CARTESIAN_POINT('Ctrl Pts',(3.82006949082991,-25.8257126129142,12.1127657467956));
#27199=CARTESIAN_POINT('Ctrl Pts',(3.08792996304833,-25.6608466898983,11.7184463463716));
#27200=CARTESIAN_POINT('Ctrl Pts',(3.19329244351081,-25.5781989955108,12.2979140331202));
#27201=CARTESIAN_POINT('Ctrl Pts',(3.53597248666522,-26.0544753237534,12.1987263107462));
#27202=CARTESIAN_POINT('Ctrl Pts',(2.95738179070761,-25.7598839936288,11.7592458546648));
#27203=CARTESIAN_POINT('Ctrl Pts',(3.0616485141192,-25.6836426250107,12.3309331047788));
#27204=CARTESIAN_POINT('Ctrl Pts',(3.38648260575685,-26.163417392629,12.2411986733987));
#27205=CARTESIAN_POINT('Ctrl Pts',(2.55511469027868,-26.0351012414329,11.8757244107345));
#27206=CARTESIAN_POINT('Ctrl Pts',(2.65679594043675,-25.9750106533199,12.4252277213909));
#27207=CARTESIAN_POINT('Ctrl Pts',(2.92584880312279,-26.4661594138917,12.362453120026));
#27208=CARTESIAN_POINT('Ctrl Pts',(2.27166012221888,-26.1910580609653,11.9460131777189));
#27209=CARTESIAN_POINT('Ctrl Pts',(2.36557359217751,-26.144410994428,12.4841667316537));
#27210=CARTESIAN_POINT('Ctrl Pts',(2.60126664333885,-26.6377134749538,12.4356238030185));
#27211=CARTESIAN_POINT('Ctrl Pts',(1.67298569393372,-26.4480533981848,12.0650208326994));
#27212=CARTESIAN_POINT('Ctrl Pts',(1.7476443014938,-26.4221373472383,12.584193569546));
#27213=CARTESIAN_POINT('Ctrl Pts',(1.91572775104536,-26.920411071464,12.5595109498063));
#27214=CARTESIAN_POINT('Ctrl Pts',(1.35365874382953,-26.5495415074398,12.114005519406));
#27215=CARTESIAN_POINT('Ctrl Pts',(1.41459460586887,-26.5335291638453,12.6263023633275));
#27216=CARTESIAN_POINT('Ctrl Pts',(1.55006815385439,-27.0320490032883,12.610504042265));
#27217=CARTESIAN_POINT('Ctrl Pts',(0.708759568526575,-26.685469004934,12.1802503963495));
#27218=CARTESIAN_POINT('Ctrl Pts',(0.742700211667052,-26.681396361373,12.6829030413056));
#27219=CARTESIAN_POINT('Ctrl Pts',(0.811597193074135,-27.1815707028637,
12.6794650457788));
#27220=CARTESIAN_POINT('Ctrl Pts',(0.381529450169107,-26.7214769991791,
12.1982295563787));
#27221=CARTESIAN_POINT('Ctrl Pts',(0.39883067063808,-26.721134815956,12.6985538974327));
#27222=CARTESIAN_POINT('Ctrl Pts',(0.436887620603506,-27.2211798544626,
12.6981813593444));
#27223=CARTESIAN_POINT('Ctrl Pts',(-0.11672432528406,-26.7263960269428,
12.2006688310083));
#27224=CARTESIAN_POINT('Ctrl Pts',(-0.121960033275976,-26.7264982085473,
12.7006498339556));
#27225=CARTESIAN_POINT('Ctrl Pts',(-0.13366049259157,-27.226590836366,12.7007206478696));
#27226=CARTESIAN_POINT('Ctrl Pts',(-0.284953721660202,-26.7196403876827,
12.1973109610589));
#27227=CARTESIAN_POINT('Ctrl Pts',(-0.298043404871046,-26.71910948222,12.69775442877));
#27228=CARTESIAN_POINT('Ctrl Pts',(-0.326299187379028,-27.219159562167,
12.6972251018568));
#27229=CARTESIAN_POINT('Ctrl Pts',(-0.616054324255102,-26.6896861218385,
12.1825046937998));
#27230=CARTESIAN_POINT('Ctrl Pts',(-0.643871216622145,-26.6864670918352,
12.6850470220168));
#27231=CARTESIAN_POINT('Ctrl Pts',(-0.70544095955049,-27.1862095499586,
12.6818117584869));
#27232=CARTESIAN_POINT('Ctrl Pts',(-0.779654440780969,-26.6665839293988,
12.1711045612618));
#27233=CARTESIAN_POINT('Ctrl Pts',(-0.814871506455407,-26.6612250484592,
12.6752407488006));
#27234=CARTESIAN_POINT('Ctrl Pts',(-0.892778674333035,-27.1607968950611,
12.6699442088688));
#27235=CARTESIAN_POINT('Ctrl Pts',(-1.10308417480477,-26.6045817512992,
12.1407978831975));
#27236=CARTESIAN_POINT('Ctrl Pts',(-1.15201059362342,-26.5937532945347,
12.6493224876276));
#27237=CARTESIAN_POINT('Ctrl Pts',(-1.26313652698652,-27.0925938369454,
12.6383949174095));
#27238=CARTESIAN_POINT('Ctrl Pts',(-1.26291351966876,-26.5656809459862,
12.1218902629486));
#27239=CARTESIAN_POINT('Ctrl Pts',(-1.3185970928561,-26.55133271456,12.6331387123477));
#27240=CARTESIAN_POINT('Ctrl Pts',(-1.44615632156059,-27.0498025433814,
12.6187120638605));
#27241=CARTESIAN_POINT('Ctrl Pts',(-1.57882910825917,-26.472045523799,12.0770004764839));
#27242=CARTESIAN_POINT('Ctrl Pts',(-1.64674489658538,-26.4496895602423,
12.5949866446668));
#27243=CARTESIAN_POINT('Ctrl Pts',(-1.80790969162943,-26.9468025811083,
12.5719817348827));
#27244=CARTESIAN_POINT('Ctrl Pts',(-1.7357664458342,-26.4169293390886,12.0508406581823));
#27245=CARTESIAN_POINT('Ctrl Pts',(-1.80956942120921,-26.3897811738161,
12.5727721171669));
#27246=CARTESIAN_POINT('Ctrl Pts',(-1.98761782339906,-26.8861742010614,
12.5447493327003));
#27247=CARTESIAN_POINT('Ctrl Pts',(-2.19294340094436,-26.2304792608021,
11.9639571152858));
#27248=CARTESIAN_POINT('Ctrl Pts',(-2.28460854688898,-26.1870098690536,
12.4991934983994));
#27249=CARTESIAN_POINT('Ctrl Pts',(-2.51112856541472,-26.6810772067274,
12.4543034671678));
#27250=CARTESIAN_POINT('Ctrl Pts',(-2.48019406540275,-26.0786113976599,
11.8949950968601));
#27251=CARTESIAN_POINT('Ctrl Pts',(-2.58014891835197,-26.0218933438711,
12.4412197385113));
#27252=CARTESIAN_POINT('Ctrl Pts',(-2.84005763385079,-26.5140210366101,
12.3825139332799));
#27253=CARTESIAN_POINT('Ctrl Pts',(-3.0221032942732,-25.7215217624029,11.742358595615));
#27254=CARTESIAN_POINT('Ctrl Pts',(-3.13102074266629,-25.6402445849069,
12.3162445020822));
#27255=CARTESIAN_POINT('Ctrl Pts',(-3.4605946074415,-26.1212186661171,12.223619062105));
#27256=CARTESIAN_POINT('Ctrl Pts',(-3.27719005316914,-25.5149405044532,
11.6582504274636));
#27257=CARTESIAN_POINT('Ctrl Pts',(-3.38703375447497,-25.419666275089,12.2483547934178));
#27258=CARTESIAN_POINT('Ctrl Pts',(-3.75269279737139,-25.8939771831764,
12.1360623135586));
#27259=CARTESIAN_POINT('Ctrl Pts',(-3.73612218146736,-25.0634149529074,
11.4900064799871));
#27260=CARTESIAN_POINT('Ctrl Pts',(-3.84117285767248,-24.9466832868258,
12.1166714943089));
#27261=CARTESIAN_POINT('Ctrl Pts',(-4.27821277731412,-25.3972942939697,
11.960919972182));
#27262=CARTESIAN_POINT('Ctrl Pts',(-3.9428591300061,-24.8169069162524,11.4050875170057));
#27263=CARTESIAN_POINT('Ctrl Pts',(-4.04093407956023,-24.6906342031624,
12.0521900648229));
#27264=CARTESIAN_POINT('Ctrl Pts',(-4.51494576615864,-25.1261328819914,
11.8725191056138));
#27265=CARTESIAN_POINT('Ctrl Pts',(-4.31056667036922,-24.2794160099143,
11.2429469206136));
#27266=CARTESIAN_POINT('Ctrl Pts',(-4.39056436964167,-24.1445715889292,
11.9333269822134));
#27267=CARTESIAN_POINT('Ctrl Pts',(-4.93600478532903,-24.5348870880994,
11.7037302415389));
#27268=CARTESIAN_POINT('Ctrl Pts',(-4.46745152170304,-23.9937229399016,
11.1675387733309));
#27269=CARTESIAN_POINT('Ctrl Pts',(-4.53383740962333,-23.86015852534,11.8809582569124));
#27270=CARTESIAN_POINT('Ctrl Pts',(-5.11565242286094,-24.2206215634778,
11.6252300596616));
#27271=CARTESIAN_POINT('Ctrl Pts',(-4.65922173876165,-23.5465266850194,
11.0715060585919));
#27272=CARTESIAN_POINT('Ctrl Pts',(-4.70540726860683,-23.4277698236053,
11.8168401515203));
#27273=CARTESIAN_POINT('Ctrl Pts',(-5.33524695956652,-23.7287004880997,
11.5252595713033));
#27274=CARTESIAN_POINT('Ctrl Pts',(-4.71608662573261,-23.3939539209264,
11.0422301701708));
#27275=CARTESIAN_POINT('Ctrl Pts',(-4.7557251197416,-23.2807813557057,11.7976839118));
#27276=CARTESIAN_POINT('Ctrl Pts',(-5.40036246187489,-23.5608687218702,
11.4947832415057));
#27277=CARTESIAN_POINT('Ctrl Pts',(-4.81528967505078,-23.0814164438215,
10.9903022583832));
#27278=CARTESIAN_POINT('Ctrl Pts',(-4.84282117938902,-22.9825138810756,
11.7642375532091));
#27279=CARTESIAN_POINT('Ctrl Pts',(-5.51395900583216,-23.2170739466321,
11.4407260503891));
#27280=CARTESIAN_POINT('Ctrl Pts',(-4.85782281130184,-22.9204654286535,
10.9675445919213));
#27281=CARTESIAN_POINT('Ctrl Pts',(-4.87941790820092,-22.8307997636199,
11.750008368624));
#27282=CARTESIAN_POINT('Ctrl Pts',(-5.5626633344584,-23.0400259697853,11.4170352072457));
#27283=CARTESIAN_POINT('Ctrl Pts',(-4.96283908675816,-22.4231124826611,
10.9107685647248));
#27284=CARTESIAN_POINT('Ctrl Pts',(-4.96989390455362,-22.3626227944554,
11.7146772216865));
#27285=CARTESIAN_POINT('Ctrl Pts',(-5.68291650617108,-22.4929321295635,
11.3579310989885));
#27286=CARTESIAN_POINT('Ctrl Pts',(-4.99857193949256,-22.0854699970494,
10.8906542554823));
#27287=CARTESIAN_POINT('Ctrl Pts',(-4.99871428575359,-22.0557131075165,
11.7032123083642));
#27288=CARTESIAN_POINT('Ctrl Pts',(-5.72383391223237,-22.1215213732838,
11.3369919725727));
#27289=CARTESIAN_POINT('Ctrl Pts',(-4.9999606548595,-21.7450738646105,10.8898978613776));
#27290=CARTESIAN_POINT('Ctrl Pts',(-4.9999232845375,-21.7434332325445,11.7027395821881));
#27291=CARTESIAN_POINT('Ctrl Pts',(-5.72542411954922,-21.7470814748957,
11.3362045626284));
#27292=CARTESIAN_POINT('',(-4.99974790012546,-21.775208915454,10.8900436331349));
#27293=CARTESIAN_POINT('',(5.00000093190807,-21.7249999999251,10.8899036431084));
#27294=CARTESIAN_POINT('Ctrl Pts',(-4.99974790012546,-21.775208915454,10.8900436331349));
#27295=CARTESIAN_POINT('Ctrl Pts',(-4.99862155597278,-21.8873690121469,
10.8906693458292));
#27296=CARTESIAN_POINT('Ctrl Pts',(-4.99372822121316,-21.9992115592643,
10.8933945121638));
#27297=CARTESIAN_POINT('Ctrl Pts',(-4.98509810138154,-22.1107420376394,
10.8981732472158));
#27298=CARTESIAN_POINT('Ctrl Pts',(-4.97648594371211,-22.2220403838331,
10.9029420361238));
#27299=CARTESIAN_POINT('Ctrl Pts',(-4.96415246845925,-22.3330286474081,
10.9097558543201));
#27300=CARTESIAN_POINT('Ctrl Pts',(-4.94807614325441,-22.4437088983424,
10.9185691027912));
#27301=CARTESIAN_POINT('Ctrl Pts',(-4.93284610808526,-22.5485627186516,
10.9269184041682));
#27302=CARTESIAN_POINT('Ctrl Pts',(-4.91425644508413,-22.653140568427,10.9370621685552));
#27303=CARTESIAN_POINT('Ctrl Pts',(-4.89224714016671,-22.757433009706,10.9489616257723));
#27304=CARTESIAN_POINT('Ctrl Pts',(-4.86468603771555,-22.8880329841149,
10.9638626942388));
#27305=CARTESIAN_POINT('Ctrl Pts',(-4.83202306043748,-23.0169058067954,
10.9813906240525));
#27306=CARTESIAN_POINT('Ctrl Pts',(-4.79452430018796,-23.1436390432055,
11.0011703424276));
#27307=CARTESIAN_POINT('Ctrl Pts',(-4.75683130501539,-23.2710287285292,
11.0210525151785));
#27308=CARTESIAN_POINT('Ctrl Pts',(-4.71425260210546,-23.3962563395395,
11.0432098643964));
#27309=CARTESIAN_POINT('Ctrl Pts',(-4.6670950177236,-23.5189409398137,11.0672614586823));
#27310=CARTESIAN_POINT('Ctrl Pts',(-4.64452824749322,-23.5776503758775,
11.0787710983095));
#27311=CARTESIAN_POINT('Ctrl Pts',(-4.6209134211507,-23.6357780439662,11.0907145202877));
#27312=CARTESIAN_POINT('Ctrl Pts',(-4.5962867820572,-23.6932855019245,11.1030499800133));
#27313=CARTESIAN_POINT('Ctrl Pts',(-4.49601285006955,-23.927442461232,11.1532770956529));
#27314=CARTESIAN_POINT('Ctrl Pts',(-4.37796206036335,-24.1536729575001,
11.2104673133284));
#27315=CARTESIAN_POINT('Ctrl Pts',(-4.24308688402606,-24.3700356698173,
11.2718912075364));
#27316=CARTESIAN_POINT('Ctrl Pts',(-4.20675437544135,-24.4283191903001,
11.2884375003697));
#27317=CARTESIAN_POINT('Ctrl Pts',(-4.16920085776234,-24.4858864280512,
11.3052910096004));
#27318=CARTESIAN_POINT('Ctrl Pts',(-4.13044480435484,-24.5426986563822,
11.322398381924));
#27319=CARTESIAN_POINT('Ctrl Pts',(-4.07064556195374,-24.6303579486633,
11.3487944623935));
#27320=CARTESIAN_POINT('Ctrl Pts',(-4.00839642509525,-24.7156218846498,
11.3755981754695));
#27321=CARTESIAN_POINT('Ctrl Pts',(-3.94374556949127,-24.7985762367506,
11.4026504426682));
#27322=CARTESIAN_POINT('Ctrl Pts',(-3.87734852680968,-24.8837711441591,
11.4304333779912));
#27323=CARTESIAN_POINT('Ctrl Pts',(-3.80841806017054,-24.966530674899,11.4584784754038));
#27324=CARTESIAN_POINT('Ctrl Pts',(-3.73695665037637,-25.0469203773131,
11.4866134152488));
#27325=CARTESIAN_POINT('Ctrl Pts',(-3.6654952405822,-25.1273100797272,11.5147483550939));
#27326=CARTESIAN_POINT('Ctrl Pts',(-3.59150241991524,-25.2053304747119,
11.5429731373713));
#27327=CARTESIAN_POINT('Ctrl Pts',(-3.51493712463866,-25.2810113905662,
11.571115442424));
#27328=CARTESIAN_POINT('Ctrl Pts',(-3.44606366015048,-25.3490893213272,
11.596430541656));
#27329=CARTESIAN_POINT('Ctrl Pts',(-3.37490019206008,-25.4154688541623,
11.6217515149196));
#27330=CARTESIAN_POINT('Ctrl Pts',(-3.30165936568716,-25.4798695627106,
11.6468682576675));
#27331=CARTESIAN_POINT('Ctrl Pts',(-3.22851890098722,-25.5441820231714,
11.6719505830222));
#27332=CARTESIAN_POINT('Ctrl Pts',(-3.15330706396815,-25.6065207404411,
11.6968292371907));
#27333=CARTESIAN_POINT('Ctrl Pts',(-3.0762736333601,-25.666641857487,11.7212949781596));
#27334=CARTESIAN_POINT('Ctrl Pts',(-2.9992662633753,-25.7267426353922,11.7457524423004));
#27335=CARTESIAN_POINT('Ctrl Pts',(-2.92043887733222,-25.7846270223891,
11.7697972725738));
#27336=CARTESIAN_POINT('Ctrl Pts',(-2.84007419592335,-25.8400915617578,
11.793220439256));
#27337=CARTESIAN_POINT('Ctrl Pts',(-2.81520835764417,-25.8572529844374,
11.8004678601938));
#27338=CARTESIAN_POINT('Ctrl Pts',(-2.7901955634273,-25.8741830466732,11.8076557654808));
#27339=CARTESIAN_POINT('Ctrl Pts',(-2.76504474865934,-25.890876562971,11.8147779632489));
#27340=CARTESIAN_POINT('Ctrl Pts',(-2.67541351514142,-25.9503680932188,
11.8401597004694));
#27341=CARTESIAN_POINT('Ctrl Pts',(-2.58395536026546,-26.0069103550976,
11.8647470590679));
#27342=CARTESIAN_POINT('Ctrl Pts',(-2.49063957468001,-26.0605177901881,
11.8884047411879));
#27343=CARTESIAN_POINT('Ctrl Pts',(-2.39717760460386,-26.1142092043777,
11.9120994844139));
#27344=CARTESIAN_POINT('Ctrl Pts',(-2.30185161455251,-26.1649569339623,
11.9348616360976));
#27345=CARTESIAN_POINT('Ctrl Pts',(-2.20460789532439,-26.2127281588654,
11.9565552615305));
#27346=CARTESIAN_POINT('Ctrl Pts',(-2.10736417609627,-26.2604993837685,
11.9782488869635));
#27347=CARTESIAN_POINT('Ctrl Pts',(-2.00820212260246,-26.3052944118206,
11.9988739861457));
#27348=CARTESIAN_POINT('Ctrl Pts',(-1.9070539613402,-26.3470282548397,12.0182946243687));
#27349=CARTESIAN_POINT('Ctrl Pts',(-1.83958236011387,-26.3748671120042,
12.0312492993859));
#27350=CARTESIAN_POINT('Ctrl Pts',(-1.77116522528206,-26.4013624874179,
12.0436669537073));
#27351=CARTESIAN_POINT('Ctrl Pts',(-1.70211845445723,-26.4263607356803,
12.0554616259635));
#27352=CARTESIAN_POINT('Ctrl Pts',(-1.63312683696538,-26.4513390157864,
12.0672468768452));
#27353=CARTESIAN_POINT('Ctrl Pts',(-1.56350692997892,-26.4748224190479,
12.0784101405182));
#27354=CARTESIAN_POINT('Ctrl Pts',(-1.49359250753464,-26.4967063427496,
12.0888656614418));
#27355=CARTESIAN_POINT('Ctrl Pts',(-1.47621822254929,-26.5021446702605,
12.0914639407932));
#27356=CARTESIAN_POINT('Ctrl Pts',(-1.4588258251848,-26.5074844603353,12.0940185126651));
#27357=CARTESIAN_POINT('Ctrl Pts',(-1.44142057741721,-26.5127245867947,
12.0965280609763));
#27358=CARTESIAN_POINT('Ctrl Pts',(-1.33443605684673,-26.5449339770008,
12.1119534560361));
#27359=CARTESIAN_POINT('Ctrl Pts',(-1.2265643434951,-26.5735040359102,12.1257607110881));
#27360=CARTESIAN_POINT('Ctrl Pts',(-1.11780240571892,-26.5984502954035,
12.1378800488878));
#27361=CARTESIAN_POINT('Ctrl Pts',(-1.06640774795444,-26.6102384677677,
12.1436069532744));
#27362=CARTESIAN_POINT('Ctrl Pts',(-1.0148140761704,-26.6212167384201,12.1489569515008));
#27363=CARTESIAN_POINT('Ctrl Pts',(-0.963020157800805,-26.6313827995448,
12.1539226808697));
#27364=CARTESIAN_POINT('Ctrl Pts',(-0.855269211084243,-26.6525320530682,
12.1642532767675));
#27365=CARTESIAN_POINT('Ctrl Pts',(-0.746653788707331,-26.6701690181909,
12.1729212537809));
#27366=CARTESIAN_POINT('Ctrl Pts',(-0.637152302600715,-26.6842375364859,
12.1798520908436));
#27367=CARTESIAN_POINT('Ctrl Pts',(-0.5826308696635,-26.6912423343568,12.1833029953157));
#27368=CARTESIAN_POINT('Ctrl Pts',(-0.527889749065468,-26.6973616759382,
12.1863232449754));
#27369=CARTESIAN_POINT('Ctrl Pts',(-0.47292655284801,-26.7025837989542,
12.1889036412423));
#27370=CARTESIAN_POINT('Ctrl Pts',(-0.404235664745158,-26.7091102073955,
12.1921285212244));
#27371=CARTESIAN_POINT('Ctrl Pts',(-0.335041472045689,-26.7142453423437,
12.1946593254799));
#27372=CARTESIAN_POINT('Ctrl Pts',(-0.265699869767895,-26.7179353670166,
12.1964843947152));
#27373=CARTESIAN_POINT('Ctrl Pts',(-0.196380842097205,-26.7216241903782,
12.1983088697875));
#27374=CARTESIAN_POINT('Ctrl Pts',(-0.126914850849468,-26.7238688082875,
12.199428069278));
#27375=CARTESIAN_POINT('Ctrl Pts',(-0.0576609418612023,-26.7246675105234,
12.199830345277));
#27376=CARTESIAN_POINT('Ctrl Pts',(-0.0294298005914876,-26.7249930990135,
12.1999943318407));
#27377=CARTESIAN_POINT('Ctrl Pts',(-0.00123391300176287,-26.7250790148406,
12.2000391829301));
#27378=CARTESIAN_POINT('Ctrl Pts',(0.02690243843868,-26.7249276253568,12.1999641095028));
#27379=CARTESIAN_POINT('Ctrl Pts',(0.138964937173212,-26.7243246657343,
12.199665104286));
#27380=CARTESIAN_POINT('Ctrl Pts',(0.250446307094146,-26.7199615810888,
12.1975038994839));
#27381=CARTESIAN_POINT('Ctrl Pts',(0.361351533677301,-26.7119254124269,
12.1935289489303));
#27382=CARTESIAN_POINT('Ctrl Pts',(0.473050020772804,-26.7038317642803,
12.189525567153));
#27383=CARTESIAN_POINT('Ctrl Pts',(0.584164785055125,-26.69201231097,12.1836824008448));
#27384=CARTESIAN_POINT('Ctrl Pts',(0.694705554438122,-26.6765032255501,
12.1760489510065));
#27385=CARTESIAN_POINT('Ctrl Pts',(0.799969826429573,-26.6617344429996,
12.1687798724168));
#27386=CARTESIAN_POINT('Ctrl Pts',(0.904714134528312,-26.6436194134591,
12.1598873441439));
#27387=CARTESIAN_POINT('Ctrl Pts',(1.00894214499993,-26.6221456735575,12.1494141115995));
#27388=CARTESIAN_POINT('Ctrl Pts',(1.09363406960635,-26.6046968864941,12.1409039403218));
#27389=CARTESIAN_POINT('Ctrl Pts',(1.17814728800982,-26.5849902238148,12.1312966461346));
#27390=CARTESIAN_POINT('Ctrl Pts',(1.26214615412685,-26.5630767961684,12.1206897039041));
#27391=CARTESIAN_POINT('Ctrl Pts',(1.34613296222794,-26.5411665141889,12.1100842842975));
#27392=CARTESIAN_POINT('Ctrl Pts',(1.42960515522795,-26.5170501926057,12.0984795036255));
#27393=CARTESIAN_POINT('Ctrl Pts',(1.51223946396481,-26.4908296028737,12.0859727947828));
#27394=CARTESIAN_POINT('Ctrl Pts',(1.59512110193217,-26.4645305334112,12.0734286526425));
#27395=CARTESIAN_POINT('Ctrl Pts',(1.67715943435879,-26.436114726054,12.0599771752061));
#27396=CARTESIAN_POINT('Ctrl Pts',(1.75804669282504,-26.4057341118511,12.0457166728564));
#27397=CARTESIAN_POINT('Ctrl Pts',(1.82285587208338,-26.3813922969697,12.0342907515108));
#27398=CARTESIAN_POINT('Ctrl Pts',(1.88692638866243,-26.355790141741,12.0223454627404));
#27399=CARTESIAN_POINT('Ctrl Pts',(1.95011090991557,-26.3290273065033,12.00993137371));
#27400=CARTESIAN_POINT('Ctrl Pts',(2.05042011318945,-26.2865397062684,11.9902232655323));
#27401=CARTESIAN_POINT('Ctrl Pts',(2.14890000537001,-26.240965322187,11.9693088676812));
#27402=CARTESIAN_POINT('Ctrl Pts',(2.24560160523857,-26.1923564252866,11.9473166525052));
#27403=CARTESIAN_POINT('Ctrl Pts',(2.3427067484564,-26.1435446796528,11.9252326620931));
#27404=CARTESIAN_POINT('Ctrl Pts',(2.43801933205824,-26.091672772653,11.9020618399542));
#27405=CARTESIAN_POINT('Ctrl Pts',(2.53157272698267,-26.0367443718288,11.8779342735337));
#27406=CARTESIAN_POINT('Ctrl Pts',(2.62284040748174,-25.9831579921918,11.8543961964275));
#27407=CARTESIAN_POINT('Ctrl Pts',(2.71243423321569,-25.9266621694752,11.8299475546468));
#27408=CARTESIAN_POINT('Ctrl Pts',(2.8003604129185,-25.8672194000027,11.8047091317359));
#27409=CARTESIAN_POINT('Ctrl Pts',(2.860949369842,-25.8262580457035,11.7873176139452));
#27410=CARTESIAN_POINT('Ctrl Pts',(2.92085135042964,-25.7838189328308,11.7695149004781));
#27411=CARTESIAN_POINT('Ctrl Pts',(2.979771996753,-25.740091387175,11.7514368077031));
#27412=CARTESIAN_POINT('Ctrl Pts',(3.03873246635287,-25.696334286953,11.7333464963097));
#27413=CARTESIAN_POINT('Ctrl Pts',(3.09670997807265,-25.6512872316562,11.7149804332359));
#27414=CARTESIAN_POINT('Ctrl Pts',(3.15344090921893,-25.6051817524524,11.6964747104228));
#27415=CARTESIAN_POINT('Ctrl Pts',(3.16531031431661,-25.5955354343181,11.6926028910069));
#27416=CARTESIAN_POINT('Ctrl Pts',(3.17712526920413,-25.5858429232248,11.6887249580996));
#27417=CARTESIAN_POINT('Ctrl Pts',(3.18888355034015,-25.576106555572,11.6848421581069));
#27418=CARTESIAN_POINT('Ctrl Pts',(3.27071584751788,-25.5083458580709,11.6578196333676));
#27419=CARTESIAN_POINT('Ctrl Pts',(3.35003194509616,-25.4382776550022,11.630495647921));
#27420=CARTESIAN_POINT('Ctrl Pts',(3.42690620703297,-25.3659221150965,11.6030230525742));
#27421=CARTESIAN_POINT('Ctrl Pts',(3.46663172712634,-25.3285316884183,11.5888263226028));
#27422=CARTESIAN_POINT('Ctrl Pts',(3.50570473102955,-25.2905297142222,11.5745899077572));
#27423=CARTESIAN_POINT('Ctrl Pts',(3.54413226871441,-25.2519145810265,11.5603349008083));
#27424=CARTESIAN_POINT('Ctrl Pts',(3.63371231053588,-25.1618972274563,11.5271044573404));
#27425=CARTESIAN_POINT('Ctrl Pts',(3.71989006886463,-25.0684457181042,11.4937239948699));
#27426=CARTESIAN_POINT('Ctrl Pts',(3.80256443311774,-24.9716141951251,11.4605294433205));
#27427=CARTESIAN_POINT('Ctrl Pts',(3.88413333468549,-24.8760774342695,11.4277787456602));
#27428=CARTESIAN_POINT('Ctrl Pts',(3.96229233349035,-24.7772497347628,11.3952090204235));
#27429=CARTESIAN_POINT('Ctrl Pts',(4.03690038853381,-24.6751585132083,11.3631429014686));
#27430=CARTESIAN_POINT('Ctrl Pts',(4.07709703146054,-24.6201547421492,11.3458666122942));
#27431=CARTESIAN_POINT('Ctrl Pts',(4.11626213049796,-24.5642032928262,11.3287365069273));
#27432=CARTESIAN_POINT('Ctrl Pts',(4.1543676039913,-24.5073065630709,11.3118030424508));
#27433=CARTESIAN_POINT('Ctrl Pts',(4.21421033911305,-24.4179531023762,11.2852098857081));
#27434=CARTESIAN_POINT('Ctrl Pts',(4.27098639377895,-24.3269514107848,11.2593090022837));
#27435=CARTESIAN_POINT('Ctrl Pts',(4.32474835890819,-24.2342930542527,11.2342641385601));
#27436=CARTESIAN_POINT('Ctrl Pts',(4.37895464840352,-24.140868907902,11.2090122875516));
#27437=CARTESIAN_POINT('Ctrl Pts',(4.43009721669823,-24.0457600597992,11.1846306641376));
#27438=CARTESIAN_POINT('Ctrl Pts',(4.47818472846866,-23.948929301419,11.1612871082715));
#27439=CARTESIAN_POINT('Ctrl Pts',(4.52627224023909,-23.8520985430388,11.1379435524055));
#27440=CARTESIAN_POINT('Ctrl Pts',(4.57130500244527,-23.7535452679376,11.1156380640875));
#27441=CARTESIAN_POINT('Ctrl Pts',(4.61324143793115,-23.6532124974584,11.0945384832709));
#27442=CARTESIAN_POINT('Ctrl Pts',(4.64779437854339,-23.5705447118047,11.077153778194));
#27443=CARTESIAN_POINT('Ctrl Pts',(4.68032091015781,-23.4864689291325,11.0605827600001));
#27444=CARTESIAN_POINT('Ctrl Pts',(4.71063625737614,-23.401277438461,11.0449609415872));
#27445=CARTESIAN_POINT('Ctrl Pts',(4.74089320150449,-23.316250070808,11.0293692189031));
#27446=CARTESIAN_POINT('Ctrl Pts',(4.76894726681297,-23.2301116686913,11.0147230422201));
#27447=CARTESIAN_POINT('Ctrl Pts',(4.79466151550492,-23.1431752189825,11.0011571427398));
#27448=CARTESIAN_POINT('Ctrl Pts',(4.82036529714633,-23.0562741569773,10.9875967652935));
#27449=CARTESIAN_POINT('Ctrl Pts',(4.84373102103341,-22.9685761046264,10.9751157857696));
#27450=CARTESIAN_POINT('Ctrl Pts',(4.86467135302676,-22.8804101553305,10.9638487709085));
#27451=CARTESIAN_POINT('Ctrl Pts',(4.87800732471196,-22.8242611599954,10.9566733072523));
#27452=CARTESIAN_POINT('Ctrl Pts',(4.8903605993491,-22.7679227065184,10.9499902098156));
#27453=CARTESIAN_POINT('Ctrl Pts',(4.90171939734693,-22.7114821081362,10.9438342370992));
#27454=CARTESIAN_POINT('Ctrl Pts',(4.92224489379668,-22.6094932091403,10.9327103139376));
#27455=CARTESIAN_POINT('Ctrl Pts',(4.9395767042353,-22.5069383142082,10.9232291557851));
#27456=CARTESIAN_POINT('Ctrl Pts',(4.95371419021583,-22.4037604302362,10.9154640387934));
#27457=CARTESIAN_POINT('Ctrl Pts',(4.9677954134181,-22.300993162014,10.9077298245419));
#27458=CARTESIAN_POINT('Ctrl Pts',(4.97870774356615,-22.197607242805,10.9016980200141));
#27459=CARTESIAN_POINT('Ctrl Pts',(4.98639906423008,-22.093543582559,10.8974410299904));
#27460=CARTESIAN_POINT('Ctrl Pts',(4.99400877478537,-21.9905841080553,10.893229209507));
#27461=CARTESIAN_POINT('Ctrl Pts',(4.99846543872905,-21.8869606057259,10.8907547393857));
#27462=CARTESIAN_POINT('Ctrl Pts',(4.99966795889425,-21.7826220513888,10.8900877439848));
#27463=CARTESIAN_POINT('Ctrl Pts',(4.99988904773768,-21.7634389299979,10.8899651138235));
#27464=CARTESIAN_POINT('Ctrl Pts',(5.,-21.7442316692363,10.8899035808404));
#27465=CARTESIAN_POINT('Ctrl Pts',(5.,-21.725,10.8899035808404));
#27466=CARTESIAN_POINT('',(-5.7251211610453,-21.780229807,11.3363568967879));
#27467=CARTESIAN_POINT('Origin',(-5.49972269013801,-21.7802298069994,10.8900436331349));
#27468=CARTESIAN_POINT('',(5.90594023139769E-11,-27.2249981621,12.6999990362978));
#27469=CARTESIAN_POINT('Ctrl Pts',(1.18064065468548E-10,-27.2249963242,
12.6999980725955));
#27470=CARTESIAN_POINT('Ctrl Pts',(-0.171632395971071,-27.2249764687244,
12.6999876622625));
#27471=CARTESIAN_POINT('Ctrl Pts',(-0.34497573023189,-27.2174810037563,
12.6964657742887));
#27472=CARTESIAN_POINT('Ctrl Pts',(-0.515865020136667,-27.202628290705,
12.6895186386625));
#27473=CARTESIAN_POINT('Ctrl Pts',(-0.529884766594002,-27.2014097750724,
12.6889486960983));
#27474=CARTESIAN_POINT('Ctrl Pts',(-0.543892550080955,-27.2001423452679,
12.6883559858665));
#27475=CARTESIAN_POINT('Ctrl Pts',(-0.557888332060774,-27.1988261027941,
12.6877406113709));
#27476=CARTESIAN_POINT('Ctrl Pts',(-0.733011862938552,-27.1823564957489,
12.6800406804463));
#27477=CARTESIAN_POINT('Ctrl Pts',(-0.906349061560203,-27.1582411107519,
12.6687880610839));
#27478=CARTESIAN_POINT('Ctrl Pts',(-1.07794709135125,-27.1266398382469,
12.6541704614814));
#27479=CARTESIAN_POINT('Ctrl Pts',(-1.08722589090208,-27.1249310664534,
12.6533800457826));
#27480=CARTESIAN_POINT('Ctrl Pts',(-1.09649960414915,-27.1232004052766,
12.6525797890944));
#27481=CARTESIAN_POINT('Ctrl Pts',(-1.10576823104768,-27.1214478465577,
12.6517697177991));
#27482=CARTESIAN_POINT('Ctrl Pts',(-1.28133872673209,-27.0882500917697,
12.6364249833093));
#27483=CARTESIAN_POINT('Ctrl Pts',(-1.45513158176923,-27.0471835338455,
12.6175524377448));
#27484=CARTESIAN_POINT('Ctrl Pts',(-1.62701656816808,-26.998245868259,12.5953490259975));
#27485=CARTESIAN_POINT('Ctrl Pts',(-1.63201737474387,-26.9968220801493,
12.594703041902));
#27486=CARTESIAN_POINT('Ctrl Pts',(-1.63701731244541,-26.9953913121635,
12.5940540985787));
#27487=CARTESIAN_POINT('Ctrl Pts',(-1.64201629264252,-26.9939535946684,
12.5934022164756));
#27488=CARTESIAN_POINT('Ctrl Pts',(-1.81762883641368,-26.9434470480164,
12.5705018108212));
#27489=CARTESIAN_POINT('Ctrl Pts',(-1.99221998730359,-26.8843104198491,
12.5439539328558));
#27490=CARTESIAN_POINT('Ctrl Pts',(-2.16210038387339,-26.8177548520731,
12.5146043457249));
#27491=CARTESIAN_POINT('Ctrl Pts',(-2.16326958009573,-26.8172967855746,
12.5144023481602));
#27492=CARTESIAN_POINT('Ctrl Pts',(-2.16443856124667,-26.8168383746705,
12.5142002198446));
#27493=CARTESIAN_POINT('Ctrl Pts',(-2.16560732738127,-26.8163796193749,
12.5139979609133));
#27494=CARTESIAN_POINT('Ctrl Pts',(-2.42817585265368,-26.7133181959941,
12.4685595898275));
#27495=CARTESIAN_POINT('Ctrl Pts',(-2.67998559716822,-26.5928358458073,
12.4165088834739));
#27496=CARTESIAN_POINT('Ctrl Pts',(-2.92148617968103,-26.4551266226912,
12.3594132760708));
#27497=CARTESIAN_POINT('Ctrl Pts',(-2.99451972446863,-26.4134812046575,
12.3421466734106));
#27498=CARTESIAN_POINT('Ctrl Pts',(-3.06661060146402,-26.3702603926359,
12.3244190004151));
#27499=CARTESIAN_POINT('Ctrl Pts',(-3.13777165534967,-26.3254697896135,
12.3062744139855));
#27500=CARTESIAN_POINT('Ctrl Pts',(-3.14194877443755,-26.3228406031045,
12.305209335629));
#27501=CARTESIAN_POINT('Ctrl Pts',(-3.14612271412673,-26.3202059886339,
12.3041428146321));
#27502=CARTESIAN_POINT('Ctrl Pts',(-3.15029347649961,-26.3175659473305,
12.3030748600242));
#27503=CARTESIAN_POINT('Ctrl Pts',(-3.31324758257754,-26.2144180016697,
12.2613492537928));
#27504=CARTESIAN_POINT('Ctrl Pts',(-3.47148910296816,-26.1025701354325,
12.2173084213314));
#27505=CARTESIAN_POINT('Ctrl Pts',(-3.62330617417467,-25.9833742848673,
12.1721206971488));
#27506=CARTESIAN_POINT('Ctrl Pts',(-3.75269317403453,-25.8817889138823,
12.1336091910579));
#27507=CARTESIAN_POINT('Ctrl Pts',(-3.87741323405155,-25.774867164968,12.0942651966009));
#27508=CARTESIAN_POINT('Ctrl Pts',(-3.99639186226798,-25.6634672539009,
12.0548265200017));
#27509=CARTESIAN_POINT('Ctrl Pts',(-4.00274578696789,-25.6575180623772,
12.0527203402185));
#27510=CARTESIAN_POINT('Ctrl Pts',(-4.00908358390065,-25.6515558925673,
12.0506138106243));
#27511=CARTESIAN_POINT('Ctrl Pts',(-4.0154050829856,-25.6455808754667,12.0485070450674));
#27512=CARTESIAN_POINT('Ctrl Pts',(-4.18308716223757,-25.4870894674118,
11.9926236502703));
#27513=CARTESIAN_POINT('Ctrl Pts',(-4.34064777629496,-25.3188565700565,
11.9362388053108));
#27514=CARTESIAN_POINT('Ctrl Pts',(-4.48780703949086,-25.1403669812823,
11.8806468112938));
#27515=CARTESIAN_POINT('Ctrl Pts',(-4.56399636137668,-25.0479568914446,
11.8518649579843));
#27516=CARTESIAN_POINT('Ctrl Pts',(-4.63739813230243,-24.9527977843453,
11.8232962958883));
#27517=CARTESIAN_POINT('Ctrl Pts',(-4.70797686641107,-24.8548201088207,
11.7951242588372));
#27518=CARTESIAN_POINT('Ctrl Pts',(-4.71381080357356,-24.8467214143689,
11.7927955985691));
#27519=CARTESIAN_POINT('Ctrl Pts',(-4.71962549432073,-24.8386033842874,
11.7904696333387));
#27520=CARTESIAN_POINT('Ctrl Pts',(-4.7254209172366,-24.8304659809309,11.7881464680579));
#27521=CARTESIAN_POINT('Ctrl Pts',(-4.849069317038,-24.6568501951343,11.7385805134052));
#27522=CARTESIAN_POINT('Ctrl Pts',(-4.96233092517715,-24.4764189499148,
11.6909386109933));
#27523=CARTESIAN_POINT('Ctrl Pts',(-5.06454613053106,-24.2901935954381,
11.6464866495965));
#27524=CARTESIAN_POINT('Ctrl Pts',(-5.13166827091823,-24.1679041146944,
11.6172961707139));
#27525=CARTESIAN_POINT('Ctrl Pts',(-5.19402747768693,-24.0431170557518,
11.5894817374231));
#27526=CARTESIAN_POINT('Ctrl Pts',(-5.25144368329969,-23.9161310885085,
11.5634052940795));
#27527=CARTESIAN_POINT('Ctrl Pts',(-5.25497935242791,-23.9083113386782,
11.5617995161511));
#27528=CARTESIAN_POINT('Ctrl Pts',(-5.2584964217271,-23.9004829362191,11.5602002646197));
#27529=CARTESIAN_POINT('Ctrl Pts',(-5.26199484288721,-23.8926459553828,
11.5586076269338));
#27530=CARTESIAN_POINT('Ctrl Pts',(-5.33218637120295,-23.7354065502039,
11.5266533057958));
#27531=CARTESIAN_POINT('Ctrl Pts',(-5.39508015392478,-23.5743103376335,
11.4972547885584));
#27532=CARTESIAN_POINT('Ctrl Pts',(-5.45035838176973,-23.4092290587574,
11.4709892437974));
#27533=CARTESIAN_POINT('Ctrl Pts',(-5.4526197177918,-23.4024758711636,11.4699147661084));
#27534=CARTESIAN_POINT('Ctrl Pts',(-5.45486833919957,-23.3957159278597,
11.4688455187614));
#27535=CARTESIAN_POINT('Ctrl Pts',(-5.4571042251612,-23.388949216604,11.4677815411574));
#27536=CARTESIAN_POINT('Ctrl Pts',(-5.50854732838719,-23.2332612112242,
11.4433016210485));
#27537=CARTESIAN_POINT('Ctrl Pts',(-5.55343224177118,-23.0730960972466,
11.4215204228469));
#27538=CARTESIAN_POINT('Ctrl Pts',(-5.59069638198729,-22.911046832253,11.4032502530102));
#27539=CARTESIAN_POINT('Ctrl Pts',(-5.59337746515253,-22.8993876995374,
11.4019357494555));
#27540=CARTESIAN_POINT('Ctrl Pts',(-5.59601909769806,-22.887718835213,11.4006394240543));
#27541=CARTESIAN_POINT('Ctrl Pts',(-5.59862088330176,-22.8760412148246,
11.3993615807472));
#27542=CARTESIAN_POINT('Ctrl Pts',(-5.59971764885756,-22.8711185909937,
11.3988229143317));
#27543=CARTESIAN_POINT('Ctrl Pts',(-5.60080729581453,-22.8661946078742,
11.3982875507515));
#27544=CARTESIAN_POINT('Ctrl Pts',(-5.60188979660494,-22.8612693368901,
11.397755511778));
#27545=CARTESIAN_POINT('Ctrl Pts',(-5.65190530306711,-22.6337037545663,
11.3731733600113));
#27546=CARTESIAN_POINT('Ctrl Pts',(-5.68664788019735,-22.4049656318907,
11.3557815554441));
#27547=CARTESIAN_POINT('Ctrl Pts',(-5.70627364103823,-22.1749701955463,
11.3458925282718));
#27548=CARTESIAN_POINT('Ctrl Pts',(-5.71746617897322,-22.043804190466,11.3402528329416));
#27549=CARTESIAN_POINT('Ctrl Pts',(-5.72374125703581,-21.9122292652076,
11.3370537800739));
#27550=CARTESIAN_POINT('Ctrl Pts',(-5.7251211610453,-21.780229807,11.3363568967879));
#27551=CARTESIAN_POINT('',(5.72518221930917,-21.6759575456936,11.3363260607529));
#27552=CARTESIAN_POINT('Ctrl Pts',(5.72518221930917,-21.6759575456936,11.3363260607529));
#27553=CARTESIAN_POINT('Ctrl Pts',(5.72869753618992,-22.054656247908,11.3345507210535));
#27554=CARTESIAN_POINT('Ctrl Pts',(5.69169600405042,-22.4271933388261,11.353483157288));
#27555=CARTESIAN_POINT('Ctrl Pts',(5.54179856043293,-23.1557233325998,11.4273991757061));
#27556=CARTESIAN_POINT('Ctrl Pts',(5.42683471955466,-23.515723594293,11.4832806925781));
#27557=CARTESIAN_POINT('Ctrl Pts',(5.13200755045586,-24.1906498178588,11.6180363676468));
#27558=CARTESIAN_POINT('Ctrl Pts',(4.95210182586657,-24.5091884261888,11.6969653793332));
#27559=CARTESIAN_POINT('Ctrl Pts',(4.52772048446401,-25.1108860436928,11.8676896990794));
#27560=CARTESIAN_POINT('Ctrl Pts',(4.28895572693526,-25.3857672051624,11.9570844402389));
#27561=CARTESIAN_POINT('Ctrl Pts',(3.89416364467019,-25.7607959445649,12.0890339520237));
#27562=CARTESIAN_POINT('Ctrl Pts',(3.75631023962589,-25.8796597515521,12.132715698208));
#27563=CARTESIAN_POINT('Ctrl Pts',(3.46769878466619,-26.105090547267,12.218335482736));
#27564=CARTESIAN_POINT('Ctrl Pts',(3.31654194508705,-26.2117959753026,12.2603439327474));
#27565=CARTESIAN_POINT('Ctrl Pts',(2.85271276315387,-26.5069617657877,12.3795785542984));
#27566=CARTESIAN_POINT('Ctrl Pts',(2.52697785378788,-26.673150598635,12.4509224724164));
#27567=CARTESIAN_POINT('Ctrl Pts',(1.84139507760884,-26.9449521303425,12.5706146093107));
#27568=CARTESIAN_POINT('Ctrl Pts',(1.47783781121532,-27.0506741288963,12.6190624489701));
#27569=CARTESIAN_POINT('Ctrl Pts',(0.746514761693329,-27.1897926257461,
12.6833535548702));
#27570=CARTESIAN_POINT('Ctrl Pts',(0.375845029736948,-27.225,12.7));
#27571=CARTESIAN_POINT('Ctrl Pts',(5.47391594054725E-14,-27.225,12.7));
#27572=CARTESIAN_POINT('',(4.99980122230293,-21.6804159506306,10.890014011117));
#27573=CARTESIAN_POINT('Origin',(5.49978134453322,-21.6759575456936,10.890014011117));
#27574=CARTESIAN_POINT('Ctrl Pts',(5.00000186381615,-21.7249999998502,10.8899037053764));
#27575=CARTESIAN_POINT('Ctrl Pts',(5.00000067893857,-21.710138258254,10.889903626456));
#27576=CARTESIAN_POINT('Ctrl Pts',(4.99993373995471,-21.6952769138386,10.8899403932703));
#27577=CARTESIAN_POINT('Ctrl Pts',(4.99980122230293,-21.6804159506306,10.890014011117));
#27578=CARTESIAN_POINT('Ctrl Pts',(0.187614356002326,-16.7285211545107,
-12.1982543436608));
#27579=CARTESIAN_POINT('Ctrl Pts',(0.196065836120502,-16.7288385017964,
-12.6985003258571));
#27580=CARTESIAN_POINT('Ctrl Pts',(0.214833815848565,-16.2288732699618,
-12.6981828003682));
#27581=CARTESIAN_POINT('Ctrl Pts',(-0.147150608123537,-16.7159509595597,
-12.2044844246647));
#27582=CARTESIAN_POINT('Ctrl Pts',(-0.153364144532674,-16.7151512337624,
-12.7038460495061));
#27583=CARTESIAN_POINT('Ctrl Pts',(-0.168499981233245,-16.2150460406695,
-12.7046682214451));
#27584=CARTESIAN_POINT('Ctrl Pts',(-0.477103276237398,-16.736913068974,
-12.1939867058945));
#27585=CARTESIAN_POINT('Ctrl Pts',(-0.500337628562375,-16.7382895625106,
-12.6946996408902));
#27586=CARTESIAN_POINT('Ctrl Pts',(-0.546322358158132,-16.2381043757634,
-12.6937402597205));
#27587=CARTESIAN_POINT('Ctrl Pts',(-1.1277665069231,-16.8427073547839,-12.1420671135872));
#27588=CARTESIAN_POINT('Ctrl Pts',(-1.17908021929114,-16.8534749528196,
-12.6502386327239));
#27589=CARTESIAN_POINT('Ctrl Pts',(-1.29138509026417,-16.3544780903702,
-12.639692814658));
#27590=CARTESIAN_POINT('Ctrl Pts',(-1.45180549185659,-16.9291924465061,
-12.0998581413745));
#27591=CARTESIAN_POINT('Ctrl Pts',(-1.51789645660857,-16.9485764266167,
-12.6138005825543));
#27592=CARTESIAN_POINT('Ctrl Pts',(-1.6624362885213,-16.4496116918588,-12.5957539678988));
#27593=CARTESIAN_POINT('Ctrl Pts',(-2.06567044084562,-17.1598587200229,
-11.9914081040113));
#27594=CARTESIAN_POINT('Ctrl Pts',(-2.15329340789673,-17.1983479333955,
-12.5221940651536));
#27595=CARTESIAN_POINT('Ctrl Pts',(-2.36536197212213,-16.7033445913232,
-12.4828592547569));
#27596=CARTESIAN_POINT('Ctrl Pts',(-2.35751884362729,-17.3036147067357,
-11.9253357164031));
#27597=CARTESIAN_POINT('Ctrl Pts',(-2.4544528650964,-17.3549880636414,-12.4663842122447));
#27598=CARTESIAN_POINT('Ctrl Pts',(-2.69955231567642,-16.8614761770065,
-12.4140789843431));
#27599=CARTESIAN_POINT('Ctrl Pts',(-2.91233266304311,-17.6476403801818,
-11.7760710934922));
#27600=CARTESIAN_POINT('Ctrl Pts',(-3.02007704204278,-17.7234499869819,
-12.3435601844791));
#27601=CARTESIAN_POINT('Ctrl Pts',(-3.33485961450271,-17.2399044186028,
-12.2586969571052));
#27602=CARTESIAN_POINT('Ctrl Pts',(-3.17086067768701,-17.8456812804081,
-11.6939431718919));
#27603=CARTESIAN_POINT('Ctrl Pts',(-3.28059025491442,-17.9355317918585,
-12.2768183621404));
#27604=CARTESIAN_POINT('Ctrl Pts',(-3.63089538292129,-17.4577494084836,
-12.1732031391639));
#27605=CARTESIAN_POINT('Ctrl Pts',(-3.52407060676517,-18.1743952416661,
-11.5685539618248));
#27606=CARTESIAN_POINT('Ctrl Pts',(-3.62848602121164,-18.2778735858662,
-12.1788301241707));
#27607=CARTESIAN_POINT('Ctrl Pts',(-4.0353497028142,-17.8193347658154,-12.0426750252286));
#27608=CARTESIAN_POINT('Ctrl Pts',(-3.63648642665548,-18.2895856083501,
-11.5262563077414));
#27609=CARTESIAN_POINT('Ctrl Pts',(-3.7392140074201,-18.398386108395,-12.1459008906374));
#27610=CARTESIAN_POINT('Ctrl Pts',(-4.16407503160209,-17.946044168994,-11.998643861893));
#27611=CARTESIAN_POINT('Ctrl Pts',(-3.85069511498075,-18.5315296768142,
-11.4417639857172));
#27612=CARTESIAN_POINT('Ctrl Pts',(-3.94847315831418,-18.6493371688439,
-12.0811442331505));
#27613=CARTESIAN_POINT('Ctrl Pts',(-4.40936153697645,-18.2121826446868,
-11.9106887386745));
#27614=CARTESIAN_POINT('Ctrl Pts',(-3.95295516857438,-18.65898775844,-11.3993577635689));
#27615=CARTESIAN_POINT('Ctrl Pts',(-4.04721398913553,-18.7806881323527,
-12.0491838773451));
#27616=CARTESIAN_POINT('Ctrl Pts',(-4.52645768074693,-18.3523865344591,
-11.866544557826));
#27617=CARTESIAN_POINT('Ctrl Pts',(-4.23843895754273,-19.052776632876,-11.2762442535035));
#27618=CARTESIAN_POINT('Ctrl Pts',(-4.32309558726455,-19.1866873378205,
-11.9570751357176));
#27619=CARTESIAN_POINT('Ctrl Pts',(-4.85336001939467,-18.7855542958133,
-11.7383854100975));
#27620=CARTESIAN_POINT('Ctrl Pts',(-4.40155791261274,-19.330923757405,-11.1993211789935));
#27621=CARTESIAN_POINT('Ctrl Pts',(-4.47343443863781,-19.4655205022704,
-11.9028712224275));
#27622=CARTESIAN_POINT('Ctrl Pts',(-5.04014459444579,-19.0915161328719,
-11.6583097529126));
#27623=CARTESIAN_POINT('Ctrl Pts',(-4.67409657173356,-19.9199697089661,
-11.0648949485446));
#27624=CARTESIAN_POINT('Ctrl Pts',(-4.72137264525855,-20.0436505033221,
-11.8111411860372));
#27625=CARTESIAN_POINT('Ctrl Pts',(-5.35222369623599,-19.7394666801363,
-11.5183742487049));
#27626=CARTESIAN_POINT('Ctrl Pts',(-4.78415488912749,-20.2350602306099,
-11.0070077703532));
#27627=CARTESIAN_POINT('Ctrl Pts',(-4.81645131220685,-20.3443906592467,
-11.7743644929088));
#27628=CARTESIAN_POINT('Ctrl Pts',(-5.47824949189502,-20.0860662537499,
-11.4581146468883));
#27629=CARTESIAN_POINT('Ctrl Pts',(-4.9380429612508,-20.8742413782898,-10.92446348534));
#27630=CARTESIAN_POINT('Ctrl Pts',(-4.94915052970332,-20.945781637773,-11.7227342826741));
#27631=CARTESIAN_POINT('Ctrl Pts',(-5.65446394825126,-20.7891655160397,
-11.3721873979728));
#27632=CARTESIAN_POINT('Ctrl Pts',(-4.98336003428014,-21.1995722326102,
-10.8991403351018));
#27633=CARTESIAN_POINT('Ctrl Pts',(-4.98610318476649,-21.2430778372018,
-11.7080708691409));
#27634=CARTESIAN_POINT('Ctrl Pts',(-5.70635571235477,-21.1470294558371,
-11.3458264145314));
#27635=CARTESIAN_POINT('Ctrl Pts',(-5.00266731696081,-21.6965815497726,
-10.8884241164298));
#27636=CARTESIAN_POINT('Ctrl Pts',(-5.00223861227093,-21.6991431073381,
-11.701699163389));
#27637=CARTESIAN_POINT('Ctrl Pts',(-5.72846413213322,-21.6937397047669,
-11.3346710063863));
#27638=CARTESIAN_POINT('Ctrl Pts',(-5.00081507698038,-21.8648821580315,
-10.8894579454085));
#27639=CARTESIAN_POINT('Ctrl Pts',(-5.00070606285703,-21.8530375538916,
-11.7023056251899));
#27640=CARTESIAN_POINT('Ctrl Pts',(-5.72634316547121,-21.8788703738055,
-11.3357472053704));
#27641=CARTESIAN_POINT('Ctrl Pts',(-4.98043297347855,-22.1972349510333,
-10.9007548048105));
#27642=CARTESIAN_POINT('Ctrl Pts',(-4.98363102603109,-22.1586640753178,
-11.7090448681742));
#27643=CARTESIAN_POINT('Ctrl Pts',(-5.70300398739036,-22.2444584461659,
-11.3475070510051));
#27644=CARTESIAN_POINT('Ctrl Pts',(-4.96204457374108,-22.3615907720529,
-10.9109377917453));
#27645=CARTESIAN_POINT('Ctrl Pts',(-4.96829032931648,-22.3098890090207,
-11.7150991169685));
#27646=CARTESIAN_POINT('Ctrl Pts',(-5.6819477616063,-22.4252498492313,-11.358107373132));
#27647=CARTESIAN_POINT('Ctrl Pts',(-4.9093856138036,-22.6868040641598,-10.939723249135));
#27648=CARTESIAN_POINT('Ctrl Pts',(-4.92360447493945,-22.6120103473265,
-11.7326382945398));
#27649=CARTESIAN_POINT('Ctrl Pts',(-5.62164893675429,-22.7829844706028,
-11.3880725628663));
#27650=CARTESIAN_POINT('Ctrl Pts',(-4.87511405974385,-22.8476613354423,
-10.9583260040355));
#27651=CARTESIAN_POINT('Ctrl Pts',(-4.89447456049345,-22.762190236406,-11.7440423570031));
#27652=CARTESIAN_POINT('Ctrl Pts',(-5.58240519787203,-22.9599274690212,
-11.4074377251331));
#27653=CARTESIAN_POINT('Ctrl Pts',(-4.79070121415266,-23.1659328389365,
-11.0032799996246));
#27654=CARTESIAN_POINT('Ctrl Pts',(-4.82128305228624,-23.0629430253274,
-11.7724161026754));
#27655=CARTESIAN_POINT('Ctrl Pts',(-5.48574557067997,-23.3100261227954,
-11.4542340983491));
#27656=CARTESIAN_POINT('Ctrl Pts',(-4.7402188334464,-23.3241960981967,-11.0298051346839));
#27657=CARTESIAN_POINT('Ctrl Pts',(-4.77724221450061,-23.2137337054447,
-11.7893815268673));
#27658=CARTESIAN_POINT('Ctrl Pts',(-5.42793910607718,-23.4841157078226,
-11.4818463282827));
#27659=CARTESIAN_POINT('Ctrl Pts',(-4.56702528419482,-23.786720410559,-11.118533581845));
#27660=CARTESIAN_POINT('Ctrl Pts',(-4.62424876201954,-23.6565280040077,
-11.8473998555161));
#27661=CARTESIAN_POINT('Ctrl Pts',(-5.22961829823042,-23.9928924520025,
-11.5742111885494));
#27662=CARTESIAN_POINT('Ctrl Pts',(-4.42359387417642,-24.0780740234331,
-11.1894473143436));
#27663=CARTESIAN_POINT('Ctrl Pts',(-4.49512814194823,-23.9435243529638,
-11.8955241760204));
#27664=CARTESIAN_POINT('Ctrl Pts',(-5.06537757524903,-24.3133814258724,
-11.6480312194488));
#27665=CARTESIAN_POINT('Ctrl Pts',(-4.0826233928351,-24.6297076196551,-11.3451830142359));
#27666=CARTESIAN_POINT('Ctrl Pts',(-4.17463759955658,-24.4989465486276,
-12.007578812027));
#27667=CARTESIAN_POINT('Ctrl Pts',(-4.67493842640269,-24.9201783815246,
-11.8101495324332));
#27668=CARTESIAN_POINT('Ctrl Pts',(-3.88372647707385,-24.8904795903893,
-11.4304106025715));
#27669=CARTESIAN_POINT('Ctrl Pts',(-3.984687402115,-24.7673934661874,-12.0711004171962));
#27670=CARTESIAN_POINT('Ctrl Pts',(-4.44718515387294,-25.2070275492461,
-11.8988700523303));
#27671=CARTESIAN_POINT('Ctrl Pts',(-3.44582145714119,-25.3622938940098,
-11.5990498723692));
#27672=CARTESIAN_POINT('Ctrl Pts',(-3.55485430361312,-25.2585891943117,
-12.2013450525302));
#27673=CARTESIAN_POINT('Ctrl Pts',(-3.94574801342084,-25.7260232835929,
-12.074420769944));
#27674=CARTESIAN_POINT('Ctrl Pts',(-3.20535762385381,-25.5762156720902,
-11.6832544101698));
#27675=CARTESIAN_POINT('Ctrl Pts',(-3.31545222283543,-25.4856903005333,
-12.2684573033505));
#27676=CARTESIAN_POINT('Ctrl Pts',(-3.67039721375693,-25.9613372401021,
-12.1620763107896));
#27677=CARTESIAN_POINT('Ctrl Pts',(-2.67839739753851,-25.9596625639606,
-11.8427211591104));
#27678=CARTESIAN_POINT('Ctrl Pts',(-2.78262411189189,-25.8938959406292,
-12.3978587657656));
#27679=CARTESIAN_POINT('Ctrl Pts',(-3.06698456073902,-26.3831288195538,
-12.3280785851005));
#27680=CARTESIAN_POINT('Ctrl Pts',(-2.39696430629599,-26.1249947589536,
-11.9162456328691));
#27681=CARTESIAN_POINT('Ctrl Pts',(-2.4943047005054,-26.0731137579165,-12.4592173527027));
#27682=CARTESIAN_POINT('Ctrl Pts',(-2.74472060313364,-26.5649942351177,
-12.4046163545475));
#27683=CARTESIAN_POINT('Ctrl Pts',(-1.95514407670351,-26.3297540195379,
-12.010074542758));
#27684=CARTESIAN_POINT('Ctrl Pts',(-2.03642325226439,-26.2954089354032,
-12.5382912282518));
#27685=CARTESIAN_POINT('Ctrl Pts',(-2.23880022556642,-26.7902294213573,
-12.5022907130333));
#27686=CARTESIAN_POINT('Ctrl Pts',(-1.8041850263858,-26.3910270775503,-12.038729313121));
#27687=CARTESIAN_POINT('Ctrl Pts',(-1.88026792843652,-26.3618640243966,
-12.5625025239243));
#27688=CARTESIAN_POINT('Ctrl Pts',(-2.06593973930607,-26.8576297857395,
-12.5321198581943));
#27689=CARTESIAN_POINT('Ctrl Pts',(-1.49456627687956,-26.4992186734461,
-12.0899480274511));
#27690=CARTESIAN_POINT('Ctrl Pts',(-1.55940548436926,-26.4791137879929,
-12.6058593233335));
#27691=CARTESIAN_POINT('Ctrl Pts',(-1.71140089238387,-26.9766405403565,
-12.5854377012537));
#27692=CARTESIAN_POINT('Ctrl Pts',(-1.33496957447932,-26.5463513373705,
-12.1126168837253));
#27693=CARTESIAN_POINT('Ctrl Pts',(-1.3934130031268,-26.53043167763,-12.6251936475194));
#27694=CARTESIAN_POINT('Ctrl Pts',(-1.5286495864113,-27.0284864707345,-12.6090356083803));
#27695=CARTESIAN_POINT('Ctrl Pts',(-0.850736429631688,-26.6632727202837,
-12.1692968738296));
#27696=CARTESIAN_POINT('Ctrl Pts',(-0.891162980629814,-26.6570899117739,
-12.6733724473115));
#27697=CARTESIAN_POINT('Ctrl Pts',(-0.974162944628781,-27.1570999930582,
-12.6680385491623));
#27698=CARTESIAN_POINT('Ctrl Pts',(-0.524308161271277,-26.7083885177163,
-12.1917667337562));
#27699=CARTESIAN_POINT('Ctrl Pts',(-0.548298037730936,-26.7068758397837,
-12.6929211630165));
#27700=CARTESIAN_POINT('Ctrl Pts',(-0.600375360890449,-27.2067273858123,
-12.691429313444));
#27701=CARTESIAN_POINT('Ctrl Pts',(-0.194315056429422,-26.7212227391145,
-12.19812741396));
#27702=CARTESIAN_POINT('Ctrl Pts',(-0.203067890451753,-26.7208823204571,
-12.6983912923617));
#27703=CARTESIAN_POINT('Ctrl Pts',(-0.22250666707533,-27.220845013026,-12.6980506686305));
#27704=CARTESIAN_POINT('',(-0.194315056429421,-26.7212227391145,-12.19812741396));
#27705=CARTESIAN_POINT('',(-4.99997666922215,-21.7249999973104,-10.8899189904778));
#27706=CARTESIAN_POINT('Ctrl Pts',(-0.194315056429422,-26.7212227391145,
-12.19812741396));
#27707=CARTESIAN_POINT('Ctrl Pts',(-0.517160507287741,-26.7086665070814,
-12.1919045066935));
#27708=CARTESIAN_POINT('Ctrl Pts',(-0.836463039682296,-26.6652181206119,
-12.1702661146494));
#27709=CARTESIAN_POINT('Ctrl Pts',(-1.15221063656178,-26.5904306273565,
-12.1339863259509));
#27710=CARTESIAN_POINT('Ctrl Pts',(-1.15932821021372,-26.5887447697388,
-12.1331685079511));
#27711=CARTESIAN_POINT('Ctrl Pts',(-1.16644419664539,-26.5870429349294,
-12.1323432328462));
#27712=CARTESIAN_POINT('Ctrl Pts',(-1.17355855615956,-26.5853251244403,
-12.1315105117548));
#27713=CARTESIAN_POINT('Ctrl Pts',(-1.28870992706902,-26.5575210427949,
-12.1180322815532));
#27714=CARTESIAN_POINT('Ctrl Pts',(-1.40296893847855,-26.5255529604411,
-12.1026290557827));
#27715=CARTESIAN_POINT('Ctrl Pts',(-1.51509695636072,-26.4899107581404,
-12.0856261426525));
#27716=CARTESIAN_POINT('Ctrl Pts',(-1.54970069744001,-26.4789112455903,
-12.080378886751));
#27717=CARTESIAN_POINT('Ctrl Pts',(-1.58410165154691,-26.4675621170884,
-12.0749794082388));
#27718=CARTESIAN_POINT('Ctrl Pts',(-1.61826401078079,-26.4558785310263,
-12.0694375775779));
#27719=CARTESIAN_POINT('Ctrl Pts',(-1.62865497627132,-26.4523248028207,
-12.0677519512791));
#27720=CARTESIAN_POINT('Ctrl Pts',(-1.6390259358195,-26.4487394280122,-12.0660528643397));
#27721=CARTESIAN_POINT('Ctrl Pts',(-1.64937590712078,-26.4451227862257,
-12.0643405765949));
#27722=CARTESIAN_POINT('Ctrl Pts',(-1.77283478811392,-26.4019819373357,
-12.0439156765873));
#27723=CARTESIAN_POINT('Ctrl Pts',(-1.89390130238185,-26.3542523700039,
-12.0215442646662));
#27724=CARTESIAN_POINT('Ctrl Pts',(-2.01251390952204,-26.3020956687674,
-11.9974687191318));
#27725=CARTESIAN_POINT('Ctrl Pts',(-2.02912714643473,-26.2947904450216,
-11.9940966261359));
#27726=CARTESIAN_POINT('Ctrl Pts',(-2.045692280223,-26.2873984411356,-11.9906911291611));
#27727=CARTESIAN_POINT('Ctrl Pts',(-2.0622091772275,-26.2799201687114,-11.9872529194329));
#27728=CARTESIAN_POINT('Ctrl Pts',(-2.0756450403253,-26.2738368805203,-11.9844560675063));
#27729=CARTESIAN_POINT('Ctrl Pts',(-2.08904768019195,-26.2676970992911,
-11.9816378653946));
#27730=CARTESIAN_POINT('Ctrl Pts',(-2.1024175425648,-26.261500906725,-11.9787985918042));
#27731=CARTESIAN_POINT('Ctrl Pts',(-2.21132292398046,-26.2110292791262,
-11.9556710408476));
#27732=CARTESIAN_POINT('Ctrl Pts',(-2.31827772862944,-26.1566946235418,
-11.931080510528));
#27733=CARTESIAN_POINT('Ctrl Pts',(-2.42319901808342,-26.0985597639666,
-11.9052366875763));
#27734=CARTESIAN_POINT('Ctrl Pts',(-2.52888872249225,-26.0399991405094,
-11.8792035915023));
#27735=CARTESIAN_POINT('Ctrl Pts',(-2.63251551612309,-25.9775822592216,
-11.8518983286854));
#27736=CARTESIAN_POINT('Ctrl Pts',(-2.7339708470621,-25.9113288079885,-11.8235203387557));
#27737=CARTESIAN_POINT('Ctrl Pts',(-2.78507559609586,-25.8779558352078,
-11.809225870047));
#27738=CARTESIAN_POINT('Ctrl Pts',(-2.83562895803816,-25.8436087250795,
-11.7946590258624));
#27739=CARTESIAN_POINT('Ctrl Pts',(-2.88561417754537,-25.8082859864259,
-11.779844436313));
#27740=CARTESIAN_POINT('Ctrl Pts',(-2.90446611947081,-25.7949640039616,
-11.7742571090072));
#27741=CARTESIAN_POINT('Ctrl Pts',(-2.92322108539097,-25.78151462425,-11.7686394723173));
#27742=CARTESIAN_POINT('Ctrl Pts',(-2.94187845550005,-25.767938430567,-11.7629930373066));
#27743=CARTESIAN_POINT('Ctrl Pts',(-3.0425574043087,-25.6946785391229,-11.7325237301066));
#27744=CARTESIAN_POINT('Ctrl Pts',(-3.1396582516418,-25.6183409709246,-11.7014704274661));
#27745=CARTESIAN_POINT('Ctrl Pts',(-3.2334263268648,-25.5388634611819,-11.670037162782));
#27746=CARTESIAN_POINT('Ctrl Pts',(-3.32861176523931,-25.4581845991302,
-11.6381287646264));
#27747=CARTESIAN_POINT('Ctrl Pts',(-3.42036283885039,-25.3742702133662,
-11.6058283875819));
#27748=CARTESIAN_POINT('Ctrl Pts',(-3.50889796434986,-25.2870183297407,
-11.5733422163248));
#27749=CARTESIAN_POINT('Ctrl Pts',(-3.53974158547149,-25.256621760859,-11.5620247742102));
#27750=CARTESIAN_POINT('Ctrl Pts',(-3.57019456758852,-25.2258198031469,
-11.5506847507283));
#27751=CARTESIAN_POINT('Ctrl Pts',(-3.60026510628155,-25.1946070957922,
-11.539330816509));
#27752=CARTESIAN_POINT('Ctrl Pts',(-3.62197219419989,-25.1720755079936,
-11.5311347262815));
#27753=CARTESIAN_POINT('Ctrl Pts',(-3.6434747277823,-25.1493352947599,-11.5229334023544));
#27754=CARTESIAN_POINT('Ctrl Pts',(-3.66477406772298,-25.1263866337935,
-11.5147308584899));
#27755=CARTESIAN_POINT('Ctrl Pts',(-3.85657011471908,-24.9197388001296,
-11.4408686875071));
#27756=CARTESIAN_POINT('Ctrl Pts',(-4.03300769662632,-24.6939781027987,
-11.3662983799433));
#27757=CARTESIAN_POINT('Ctrl Pts',(-4.18844906630108,-24.4556967542556,
-11.2965847525213));
#27758=CARTESIAN_POINT('Ctrl Pts',(-4.21042496844413,-24.4220091483818,
-11.2867288186893));
#27759=CARTESIAN_POINT('Ctrl Pts',(-4.23198378752848,-24.3880673310623,
-11.2769688262287));
#27760=CARTESIAN_POINT('Ctrl Pts',(-4.2531092519528,-24.3538898210574,-11.2673205519542));
#27761=CARTESIAN_POINT('Ctrl Pts',(-4.39800384639207,-24.1194743141768,
-11.2011453067637));
#27762=CARTESIAN_POINT('Ctrl Pts',(-4.52349271816479,-23.8736165952387,
-11.1399302880314));
#27763=CARTESIAN_POINT('Ctrl Pts',(-4.62889730420505,-23.6153672379701,
-11.0866584152499));
#27764=CARTESIAN_POINT('Ctrl Pts',(-4.6473789897824,-23.5700856842835,-11.0773177021002));
#27765=CARTESIAN_POINT('Ctrl Pts',(-4.66524387253178,-23.5244214900292,
-11.068221540643));
#27766=CARTESIAN_POINT('Ctrl Pts',(-4.68248793936805,-23.4783700972512,
-11.0593863294591));
#27767=CARTESIAN_POINT('Ctrl Pts',(-4.74018839941497,-23.3242772968511,
-11.0298227842256));
#27768=CARTESIAN_POINT('Ctrl Pts',(-4.79068137810927,-23.1660076341135,
-11.0032913774002));
#27769=CARTESIAN_POINT('Ctrl Pts',(-4.83290764702189,-23.006797049208,-10.980803318434));
#27770=CARTESIAN_POINT('Ctrl Pts',(-4.86052680718277,-22.902661335657,-10.966094434171));
#27771=CARTESIAN_POINT('Ctrl Pts',(-4.8847554208306,-22.7977602493764,-10.9530409731728));
#27772=CARTESIAN_POINT('Ctrl Pts',(-4.90558490800675,-22.6920927561039,
-10.9417401310877));
#27773=CARTESIAN_POINT('Ctrl Pts',(-4.91657436602273,-22.6363434968373,
-10.9357779041453));
#27774=CARTESIAN_POINT('Ctrl Pts',(-4.92661811613177,-22.5803788932101,
-10.9303032859972));
#27775=CARTESIAN_POINT('Ctrl Pts',(-4.93571509377234,-22.5241974181064,
-10.9253305204401));
#27776=CARTESIAN_POINT('Ctrl Pts',(-4.94895331108583,-22.4424403108779,
-10.9180939904964));
#27777=CARTESIAN_POINT('Ctrl Pts',(-4.96018681042669,-22.3602239878914,
-10.9119201550834));
#27778=CARTESIAN_POINT('Ctrl Pts',(-4.96938050763009,-22.2775381706359,
-10.906851659997));
#27779=CARTESIAN_POINT('Ctrl Pts',(-4.97359143004183,-22.2396661858064,
-10.9045301739745));
#27780=CARTESIAN_POINT('Ctrl Pts',(-4.97737405981722,-22.2017009246778,
-10.9024407792168));
#27781=CARTESIAN_POINT('Ctrl Pts',(-4.98072713948359,-22.1636141852628,
-10.9005864070342));
#27782=CARTESIAN_POINT('Ctrl Pts',(-4.98460401281169,-22.1195778130665,
-10.8984423583474));
#27783=CARTESIAN_POINT('Ctrl Pts',(-4.98790553699991,-22.0753865188053,
-10.8966131076855));
#27784=CARTESIAN_POINT('Ctrl Pts',(-4.99062402522946,-22.0310585545324,
-10.8951063751095));
#27785=CARTESIAN_POINT('Ctrl Pts',(-4.99646709998867,-21.935780743007,-10.8918678284097));
#27786=CARTESIAN_POINT('Ctrl Pts',(-4.99956713935828,-21.8397718638307,
-10.8901472474313));
#27787=CARTESIAN_POINT('Ctrl Pts',(-4.99993867929236,-21.7441269948327,
-10.8899402435468));
#27788=CARTESIAN_POINT('Ctrl Pts',(-4.99996345275608,-21.7377496058228,
-10.8899264409841));
#27789=CARTESIAN_POINT('Ctrl Pts',(-4.9999761122425,-21.7313738326033,-10.8899193583874));
#27790=CARTESIAN_POINT('Ctrl Pts',(-4.99997666922209,-21.7249999979848,
-10.8899189904778));
#27791=CARTESIAN_POINT('',(-0.222506667109494,-27.2208450130247,-12.6980506686299));
#27792=CARTESIAN_POINT('Origin',(-0.213746562105115,-27.2208450130247,-12.1981274139594));
#27793=CARTESIAN_POINT('',(6.27271730358628E-11,-16.2250000002193,-12.7000029635389));
#27794=CARTESIAN_POINT('Ctrl Pts',(6.27271660968204E-11,-16.2250000002193,
-12.7000029635389));
#27795=CARTESIAN_POINT('Ctrl Pts',(-0.160551351076563,-16.2250000007214,
-12.7000063618174));
#27796=CARTESIAN_POINT('Ctrl Pts',(-0.320152850111539,-16.2314747517667,
-12.6969639953539));
#27797=CARTESIAN_POINT('Ctrl Pts',(-0.478672850296259,-16.244274252264,
-12.6909831439331));
#27798=CARTESIAN_POINT('Ctrl Pts',(-0.626368403327257,-16.2561997462222,
-12.6854106915159));
#27799=CARTESIAN_POINT('Ctrl Pts',(-0.773125198619939,-16.2736151280446,
-12.6772876607414));
#27800=CARTESIAN_POINT('Ctrl Pts',(-0.918842228003057,-16.296362307571,
-12.6667173659353));
#27801=CARTESIAN_POINT('Ctrl Pts',(-0.978670211742676,-16.3057017642741,
-12.6623774515927));
#27802=CARTESIAN_POINT('Ctrl Pts',(-1.03842121787906,-16.315986503065,-12.6576040485612));
#27803=CARTESIAN_POINT('Ctrl Pts',(-1.09801247670689,-16.3271894613611,
-12.6524178644869));
#27804=CARTESIAN_POINT('Ctrl Pts',(-1.27977392123081,-16.3613600078959,
-12.6365992976794));
#27805=CARTESIAN_POINT('Ctrl Pts',(-1.46078267828966,-16.4042424440069,
-12.6168750403301));
#27806=CARTESIAN_POINT('Ctrl Pts',(-1.63879216927802,-16.4552660581236,
-12.5937448757344));
#27807=CARTESIAN_POINT('Ctrl Pts',(-1.76562069343311,-16.4916194550102,
-12.5772650542213));
#27808=CARTESIAN_POINT('Ctrl Pts',(-1.89092589627654,-16.5321045091344,
-12.5590568756658));
#27809=CARTESIAN_POINT('Ctrl Pts',(-2.01389066817964,-16.5765012422573,
-12.5393079697913));
#27810=CARTESIAN_POINT('Ctrl Pts',(-2.06065103568712,-16.5933841878752,
-12.5317979644274));
#27811=CARTESIAN_POINT('Ctrl Pts',(-2.10711393447791,-16.6108244062646,
-12.5240683173945));
#27812=CARTESIAN_POINT('Ctrl Pts',(-2.15327890344298,-16.628821268942,-12.5161272078686));
#27813=CARTESIAN_POINT('Ctrl Pts',(-2.2785130815824,-16.6776423199905,-12.4945849357239));
#27814=CARTESIAN_POINT('Ctrl Pts',(-2.40149825470153,-16.7305125267001,
-12.4714978808614));
#27815=CARTESIAN_POINT('Ctrl Pts',(-2.52242557701601,-16.7875152782616,
-12.4469915584264));
#27816=CARTESIAN_POINT('Ctrl Pts',(-2.64440787895254,-16.8450153263822,
-12.4222714408764));
#27817=CARTESIAN_POINT('Ctrl Pts',(-2.76429623934248,-16.9067202916339,
-12.3961068901205));
#27818=CARTESIAN_POINT('Ctrl Pts',(-2.88226076887571,-16.9727602251875,
-12.3686145128557));
#27819=CARTESIAN_POINT('Ctrl Pts',(-2.92752129411295,-16.9980983678572,
-12.3580662621235));
#27820=CARTESIAN_POINT('Ctrl Pts',(-2.97249834394842,-17.0240751256557,
-12.3473224388959));
#27821=CARTESIAN_POINT('Ctrl Pts',(-3.01720053215441,-17.0506995836214,
-12.3363892993782));
#27822=CARTESIAN_POINT('Ctrl Pts',(-3.05217654869923,-17.0715311697178,
-12.327834960452));
#27823=CARTESIAN_POINT('Ctrl Pts',(-3.08692270139852,-17.0927295755552,
-12.3191781477242));
#27824=CARTESIAN_POINT('Ctrl Pts',(-3.12143510339615,-17.1142923538109,
-12.3104257191235));
#27825=CARTESIAN_POINT('Ctrl Pts',(-3.2295983220598,-17.1818709448236,-12.2829952653223));
#27826=CARTESIAN_POINT('Ctrl Pts',(-3.33495104508456,-17.2526947376596,
-12.2547577203916));
#27827=CARTESIAN_POINT('Ctrl Pts',(-3.43746722042114,-17.3266314645754,
-12.2259329280528));
#27828=CARTESIAN_POINT('Ctrl Pts',(-3.54078845940789,-17.4011488195829,
-12.1968817734598));
#27829=CARTESIAN_POINT('Ctrl Pts',(-3.64122887555301,-17.478828602327,-12.167233589157));
#27830=CARTESIAN_POINT('Ctrl Pts',(-3.73872681749338,-17.5595740196141,
-12.1372060767936));
#27831=CARTESIAN_POINT('Ctrl Pts',(-3.79359932791705,-17.605018094264,-12.1203063868887));
#27832=CARTESIAN_POINT('Ctrl Pts',(-3.84753913837293,-17.6514338734209,
-12.1032864556262));
#27833=CARTESIAN_POINT('Ctrl Pts',(-3.90052960838985,-17.6988086717544,
-12.0861850380435));
#27834=CARTESIAN_POINT('Ctrl Pts',(-3.92560168088156,-17.7212237282301,
-12.0780936212056));
#27835=CARTESIAN_POINT('Ctrl Pts',(-3.95047870207009,-17.7438665863787,
-12.0699791062562));
#27836=CARTESIAN_POINT('Ctrl Pts',(-3.97516256360717,-17.7667417119757,
-12.061844261215));
#27837=CARTESIAN_POINT('Ctrl Pts',(-4.07214610519881,-17.8566186824578,
-12.029882240961));
#27838=CARTESIAN_POINT('Ctrl Pts',(-4.16604631669613,-17.9499957710841,
-11.997638384144));
#27839=CARTESIAN_POINT('Ctrl Pts',(-4.25671783397987,-18.0468318032717,
-11.9653814957961));
#27840=CARTESIAN_POINT('Ctrl Pts',(-4.26675558549422,-18.0575519947702,
-11.9618105107772));
#27841=CARTESIAN_POINT('Ctrl Pts',(-4.27675380593103,-18.0683145412742,
-11.9582393689533));
#27842=CARTESIAN_POINT('Ctrl Pts',(-4.28671232658364,-18.0791193597846,
-11.9546684365246));
#27843=CARTESIAN_POINT('Ctrl Pts',(-4.30808442495687,-18.1023077079503,
-11.9470048164136));
#27844=CARTESIAN_POINT('Ctrl Pts',(-4.32928991266167,-18.1257142901536,
-11.9393354731834));
#27845=CARTESIAN_POINT('Ctrl Pts',(-4.35031349209773,-18.1493216466888,
-11.9316693999324));
#27846=CARTESIAN_POINT('Ctrl Pts',(-4.42593746646665,-18.234239732639,-11.904093747137));
#27847=CARTESIAN_POINT('Ctrl Pts',(-4.49941729284665,-18.3220081127293,
-11.8764827830282));
#27848=CARTESIAN_POINT('Ctrl Pts',(-4.56995033927333,-18.4117704764363,
-11.8492830907707));
#27849=CARTESIAN_POINT('Ctrl Pts',(-4.5920703872979,-18.4399210795449,-11.8407529261249));
#27850=CARTESIAN_POINT('Ctrl Pts',(-4.61390078044836,-18.4682674406524,
-11.8322632536808));
#27851=CARTESIAN_POINT('Ctrl Pts',(-4.6354173416563,-18.4967822997718,-11.8238278939559));
#27852=CARTESIAN_POINT('Ctrl Pts',(-4.65353301373796,-18.5207901248266,
-11.8167258199213));
#27853=CARTESIAN_POINT('Ctrl Pts',(-4.67143565529656,-18.5449204374923,
-11.8096599383198));
#27854=CARTESIAN_POINT('Ctrl Pts',(-4.68912315776799,-18.5691708542537,
-11.8026338819312));
#27855=CARTESIAN_POINT('Ctrl Pts',(-4.78633495947354,-18.7024529108523,
-11.7640181643344));
#27856=CARTESIAN_POINT('Ctrl Pts',(-4.87725397819097,-18.8396319188562,
-11.7265223047439));
#27857=CARTESIAN_POINT('Ctrl Pts',(-4.96178027815071,-18.9806973912532,
-11.6906454810317));
#27858=CARTESIAN_POINT('Ctrl Pts',(-5.04630657811045,-19.1217628636502,
-11.6547686573195));
#27859=CARTESIAN_POINT('Ctrl Pts',(-5.12444023116057,-19.2667148316449,
-11.6205113851506));
#27860=CARTESIAN_POINT('Ctrl Pts',(-5.19612983342037,-19.4155215868604,
-11.5883663492601));
#27861=CARTESIAN_POINT('Ctrl Pts',(-5.20862363940037,-19.4414550928302,
-11.5827642280462));
#27862=CARTESIAN_POINT('Ctrl Pts',(-5.22092652900315,-19.4675351737443,
-11.5772236713179));
#27863=CARTESIAN_POINT('Ctrl Pts',(-5.23303411516651,-19.4937521092468,
-11.5717487071689));
#27864=CARTESIAN_POINT('Ctrl Pts',(-5.2881331110772,-19.6130596906717,-11.5468333340149));
#27865=CARTESIAN_POINT('Ctrl Pts',(-5.33931133249327,-19.7355273100298,
-11.5232195967625));
#27866=CARTESIAN_POINT('Ctrl Pts',(-5.38606864208178,-19.8601850940752,
-11.5013248529885));
#27867=CARTESIAN_POINT('Ctrl Pts',(-5.43394641197694,-19.9878300923159,
-11.4789054384938));
#27868=CARTESIAN_POINT('Ctrl Pts',(-5.47718805239988,-20.1177702057423,
-11.4582890473383));
#27869=CARTESIAN_POINT('Ctrl Pts',(-5.51529287795625,-20.2489262530324,
-11.4399142062654));
#27870=CARTESIAN_POINT('Ctrl Pts',(-5.53349773916788,-20.3115870211403,
-11.4311354905349));
#27871=CARTESIAN_POINT('Ctrl Pts',(-5.55053071326472,-20.3745249014908,
-11.4228682121373));
#27872=CARTESIAN_POINT('Ctrl Pts',(-5.56634084337765,-20.4376206162029,
-11.4151587639929));
#27873=CARTESIAN_POINT('Ctrl Pts',(-5.57372038673109,-20.4670712000253,
-11.411560298553));
#27874=CARTESIAN_POINT('Ctrl Pts',(-5.58084550385779,-20.496565737035,-11.4080784831432));
#27875=CARTESIAN_POINT('Ctrl Pts',(-5.58771530165224,-20.5261026282267,
-11.4047148520531));
#27876=CARTESIAN_POINT('Ctrl Pts',(-5.62523447933326,-20.6874174007898,
-11.3863444900279));
#27877=CARTESIAN_POINT('Ctrl Pts',(-5.65520198469204,-20.8502556764816,
-11.3714677743116));
#27878=CARTESIAN_POINT('Ctrl Pts',(-5.67746909575661,-21.0145222008876,
-11.3603357097898));
#27879=CARTESIAN_POINT('Ctrl Pts',(-5.69973620682117,-21.1787887252936,
-11.3492036452679));
#27880=CARTESIAN_POINT('Ctrl Pts',(-5.7143028423889,-21.344483527548,-11.3418164518137));
#27881=CARTESIAN_POINT('Ctrl Pts',(-5.72106920988503,-21.5115041954204,
-11.3384023158398));
#27882=CARTESIAN_POINT('Ctrl Pts',(-5.72241125095109,-21.5446310681913,
-11.3377251562435));
#27883=CARTESIAN_POINT('Ctrl Pts',(-5.72343991250265,-21.577851098803,-11.3372063173585));
#27884=CARTESIAN_POINT('Ctrl Pts',(-5.72415500646433,-21.6111318063052,
-11.3368457725736));
#27885=CARTESIAN_POINT('Ctrl Pts',(-5.72623376206871,-21.7078777738921,
-11.3357976802496));
#27886=CARTESIAN_POINT('Ctrl Pts',(-5.72565676881658,-21.8053972850323,
-11.3360902643429));
#27887=CARTESIAN_POINT('Ctrl Pts',(-5.72239835662252,-21.9027047860458,
-11.3377334731175));
#27888=CARTESIAN_POINT('Ctrl Pts',(-5.72062014903454,-21.9558082383917,
-11.3386302185682));
#27889=CARTESIAN_POINT('Ctrl Pts',(-5.7180441674224,-22.0088482095149,-11.3399287986014));
#27890=CARTESIAN_POINT('Ctrl Pts',(-5.71467206515978,-22.0616642937744,
-11.3416278896644));
#27891=CARTESIAN_POINT('Ctrl Pts',(-5.71244343540748,-22.0965705592471,
-11.3427508226598));
#27892=CARTESIAN_POINT('Ctrl Pts',(-5.70987306068047,-22.1313912428016,
-11.3440456125498));
#27893=CARTESIAN_POINT('Ctrl Pts',(-5.70696482992104,-22.1661172689757,
-11.3455089795396));
#27894=CARTESIAN_POINT('Ctrl Pts',(-5.69462104364358,-22.3135095087314,
-11.351720140504));
#27895=CARTESIAN_POINT('Ctrl Pts',(-5.67617402862204,-22.4594930247,-11.3609766046823));
#27896=CARTESIAN_POINT('Ctrl Pts',(-5.65179657073802,-22.6041168008349,
-11.3730908517823));
#27897=CARTESIAN_POINT('Ctrl Pts',(-5.64581627910689,-22.6395959866547,
-11.3760627256707));
#27898=CARTESIAN_POINT('Ctrl Pts',(-5.63947902636718,-22.674993314026,-11.37920660631));
#27899=CARTESIAN_POINT('Ctrl Pts',(-5.63278512402843,-22.7103090990635,
-11.3825196496405));
#27900=CARTESIAN_POINT('Ctrl Pts',(-5.60992706383812,-22.8309039776864,
-11.3938328926529));
#27901=CARTESIAN_POINT('Ctrl Pts',(-5.5828943210023,-22.9506186766624,-11.407126368778));
#27902=CARTESIAN_POINT('Ctrl Pts',(-5.55175036832976,-23.0692983375885,
-11.4222623891215));
#27903=CARTESIAN_POINT('Ctrl Pts',(-5.54599612621493,-23.0912259172459,
-11.425058961754));
#27904=CARTESIAN_POINT('Ctrl Pts',(-5.54010166696578,-23.113118194875,-11.4279183783432));
#27905=CARTESIAN_POINT('Ctrl Pts',(-5.53406756508731,-23.1349742360145,
-11.4308396971981));
#27906=CARTESIAN_POINT('Ctrl Pts',(-5.52421074093538,-23.1706765092787,
-11.4356117290306));
#27907=CARTESIAN_POINT('Ctrl Pts',(-5.51396503368307,-23.2063209196587,
-11.440556474689));
#27908=CARTESIAN_POINT('Ctrl Pts',(-5.50334318984205,-23.2418731602839,
-11.4456638614209));
#27909=CARTESIAN_POINT('Ctrl Pts',(-5.47422129239668,-23.3393466988651,
-11.4596667779433));
#27910=CARTESIAN_POINT('Ctrl Pts',(-5.44216808041369,-23.4364412947893,
-11.4749420848567));
#27911=CARTESIAN_POINT('Ctrl Pts',(-5.40744548628297,-23.5323334983927,
-11.4912810885387));
#27912=CARTESIAN_POINT('Ctrl Pts',(-5.39271029600427,-23.5730271706748,
-11.4982148541241));
#27913=CARTESIAN_POINT('Ctrl Pts',(-5.37749497084478,-23.6135044192064,
-11.5053399237658));
#27914=CARTESIAN_POINT('Ctrl Pts',(-5.36182198105209,-23.6537033130043,
-11.5126393602804));
#27915=CARTESIAN_POINT('Ctrl Pts',(-5.34807804106611,-23.6889544802143,
-11.5190403736616));
#27916=CARTESIAN_POINT('Ctrl Pts',(-5.33399487567552,-23.7239839927291,
-11.5255704863632));
#27917=CARTESIAN_POINT('Ctrl Pts',(-5.31957905406975,-23.7587842426349,
-11.5322217060459));
#27918=CARTESIAN_POINT('Ctrl Pts',(-5.21968477345348,-23.9999321996973,
-11.5783112612298));
#27919=CARTESIAN_POINT('Ctrl Pts',(-5.10354433287028,-24.2309165425076,
-11.6303378369389));
#27920=CARTESIAN_POINT('Ctrl Pts',(-4.97181336051486,-24.4524305274384,
-11.6863685750191));
#27921=CARTESIAN_POINT('Ctrl Pts',(-4.9388890927989,-24.507794771794,-11.7003726546057));
#27922=CARTESIAN_POINT('Ctrl Pts',(-4.90499097869716,-24.5625673949196,
-11.7146271094503));
#27923=CARTESIAN_POINT('Ctrl Pts',(-4.87012937260121,-24.6167591578513,
-11.7291022614585));
#27924=CARTESIAN_POINT('Ctrl Pts',(-4.85012818139547,-24.6478506631936,
-11.7374071078345));
#27925=CARTESIAN_POINT('Ctrl Pts',(-4.82979351783297,-24.6787566452107,
-11.7457890364924));
#27926=CARTESIAN_POINT('Ctrl Pts',(-4.8091365289925,-24.7094657995178,-11.7542385964132));
#27927=CARTESIAN_POINT('Ctrl Pts',(-4.75805163579853,-24.7854097756689,
-11.7751344234586));
#27928=CARTESIAN_POINT('Ctrl Pts',(-4.70484306691042,-24.8603526764483,
-11.7965054522725));
#27929=CARTESIAN_POINT('Ctrl Pts',(-4.64981679274065,-24.9339036057569,
-11.8181502989304));
#27930=CARTESIAN_POINT('Ctrl Pts',(-4.59674139491384,-25.0048468940766,
-11.8390277591002));
#27931=CARTESIAN_POINT('Ctrl Pts',(-4.54197565148049,-25.074494762381,-11.86015946751));
#27932=CARTESIAN_POINT('Ctrl Pts',(-4.48582982272794,-25.1425250797796,
-11.8813605121747));
#27933=CARTESIAN_POINT('Ctrl Pts',(-4.41553127291297,-25.2277038501857,
-11.9079057200309));
#27934=CARTESIAN_POINT('Ctrl Pts',(-4.34292780254635,-25.3105340896975,
-11.9346152987756));
#27935=CARTESIAN_POINT('Ctrl Pts',(-4.26816207748717,-25.3908946583701,
-11.9613004937469));
#27936=CARTESIAN_POINT('Ctrl Pts',(-4.24447716774308,-25.4163519493211,
-11.9697540522979));
#27937=CARTESIAN_POINT('Ctrl Pts',(-4.22057495581456,-25.4415611563123,
-11.9782052033095));
#27938=CARTESIAN_POINT('Ctrl Pts',(-4.19645917443268,-25.4665176968915,
-11.9866480049388));
#27939=CARTESIAN_POINT('Ctrl Pts',(-4.17286608252751,-25.4909333252386,
-11.9949078158743));
#27940=CARTESIAN_POINT('Ctrl Pts',(-4.14905382008069,-25.5151351607172,
-12.0031669432351));
#27941=CARTESIAN_POINT('Ctrl Pts',(-4.12501614907756,-25.5391273663444,
-12.0114232046958));
#27942=CARTESIAN_POINT('Ctrl Pts',(-4.02840878195849,-25.6355520081795,
-12.0446051082944));
#27943=CARTESIAN_POINT('Ctrl Pts',(-3.92850678614335,-25.7282868705338,
-12.077622403484));
#27944=CARTESIAN_POINT('Ctrl Pts',(-3.82511519986933,-25.8174762702012,
-12.1102803913693));
#27945=CARTESIAN_POINT('Ctrl Pts',(-3.72253229275247,-25.9059680733701,
-12.1426829442132));
#27946=CARTESIAN_POINT('Ctrl Pts',(-3.61651425633536,-25.990969588709,-12.174732203639));
#27947=CARTESIAN_POINT('Ctrl Pts',(-3.50683570393584,-26.0725844683868,
-12.2062367240606));
#27948=CARTESIAN_POINT('Ctrl Pts',(-3.46142078356523,-26.106378981357,-12.2192818933754));
#27949=CARTESIAN_POINT('Ctrl Pts',(-3.41537782072005,-26.1395923956987,
-12.2322336131407));
#27950=CARTESIAN_POINT('Ctrl Pts',(-3.36868898142294,-26.1722302124877,
-12.2450779722361));
#27951=CARTESIAN_POINT('Ctrl Pts',(-3.34494120197565,-26.1888310894085,
-12.2516111183056));
#27952=CARTESIAN_POINT('Ctrl Pts',(-3.32106222794322,-26.2052544591287,
-12.2581052773238));
#27953=CARTESIAN_POINT('Ctrl Pts',(-3.2970531911292,-26.2214997110646,-12.2645583708621));
#27954=CARTESIAN_POINT('Ctrl Pts',(-3.18926116062163,-26.2944351105913,
-12.2935304642011));
#27955=CARTESIAN_POINT('Ctrl Pts',(-3.07933993096031,-26.3634600160092,
-12.321543437565));
#27956=CARTESIAN_POINT('Ctrl Pts',(-2.96741633131083,-26.4286185085995,
-12.348436395749));
#27957=CARTESIAN_POINT('Ctrl Pts',(-2.85491302458214,-26.4941144889006,
-12.3754686457203));
#27958=CARTESIAN_POINT('Ctrl Pts',(-2.74038608933694,-26.555704132313,-12.4013696670383));
#27959=CARTESIAN_POINT('Ctrl Pts',(-2.62393179659187,-26.613391646093,-12.4259692635982));
#27960=CARTESIAN_POINT('Ctrl Pts',(-2.55248788444691,-26.6487825412605,
-12.4410609478462));
#27961=CARTESIAN_POINT('Ctrl Pts',(-2.4803179587437,-26.6827039703826,-12.4556626512271));
#27962=CARTESIAN_POINT('Ctrl Pts',(-2.40743936726011,-26.7151488232138,
-12.469732783537));
#27963=CARTESIAN_POINT('Ctrl Pts',(-2.38826730991567,-26.7236840400223,
-12.4734341912893));
#27964=CARTESIAN_POINT('Ctrl Pts',(-2.36904016562544,-26.7321202559583,
-12.4771004338297));
#27965=CARTESIAN_POINT('Ctrl Pts',(-2.34975691726018,-26.7404574419512,
-12.4807309908139));
#27966=CARTESIAN_POINT('Ctrl Pts',(-2.22751843903057,-26.7933077143316,
-12.5037454618446));
#27967=CARTESIAN_POINT('Ctrl Pts',(-2.10312858729452,-26.8421272940633,
-12.5253046284089));
#27968=CARTESIAN_POINT('Ctrl Pts',(-1.9766937777278,-26.8868045823368,-12.545225735693));
#27969=CARTESIAN_POINT('Ctrl Pts',(-1.94746069254071,-26.8971344509743,
-12.5498317095404));
#27970=CARTESIAN_POINT('Ctrl Pts',(-1.91811838175776,-26.9072430607902,
-12.554350193968));
#27971=CARTESIAN_POINT('Ctrl Pts',(-1.88866833366658,-26.9171293622485,
-12.5587790777787));
#27972=CARTESIAN_POINT('Ctrl Pts',(-1.87307483841099,-26.9223640564129,
-12.5611241258573));
#27973=CARTESIAN_POINT('Ctrl Pts',(-1.85744283727076,-26.9275382488964,
-12.5634448995501));
#27974=CARTESIAN_POINT('Ctrl Pts',(-1.84177501360111,-26.9326510488533,
-12.5657408000865));
#27975=CARTESIAN_POINT('Ctrl Pts',(-1.70170427568277,-26.9783596091414,
-12.5862662086628));
#27976=CARTESIAN_POINT('Ctrl Pts',(-1.55841542310951,-27.019262367169,-12.6048539316864));
#27977=CARTESIAN_POINT('Ctrl Pts',(-1.41371523767078,-27.0546908316659,
-12.6210683091496));
#27978=CARTESIAN_POINT('Ctrl Pts',(-1.39045059543795,-27.0603869581005,
-12.623675228343));
#27979=CARTESIAN_POINT('Ctrl Pts',(-1.36714948897486,-27.0659416747688,
-12.6262208411194));
#27980=CARTESIAN_POINT('Ctrl Pts',(-1.34381943497189,-27.0713523220188,
-12.6287033905082));
#27981=CARTESIAN_POINT('Ctrl Pts',(-1.33278908881188,-27.0739104520647,
-12.6298771288593));
#27982=CARTESIAN_POINT('Ctrl Pts',(-1.32175599390771,-27.0764361857391,
-12.6310365715612));
#27983=CARTESIAN_POINT('Ctrl Pts',(-1.31072022027439,-27.0789295403597,
-12.6321816971157));
#27984=CARTESIAN_POINT('Ctrl Pts',(-0.951608746146348,-27.1600649716452,
-12.6694448505291));
#27985=CARTESIAN_POINT('Ctrl Pts',(-0.588860750681474,-27.207157585446,
-12.6916310828017));
#27986=CARTESIAN_POINT('Ctrl Pts',(-0.222506667109494,-27.2208450130247,
-12.6980506686299));
#27987=CARTESIAN_POINT('',(0.214833815848646,-16.2288732699618,-12.6981828003682));
#27988=CARTESIAN_POINT('Origin',(-7.67065009257134E-6,-21.1105838635361,
-10.4083425226561));
#27989=CARTESIAN_POINT('',(0.187614356002326,-16.7285211545107,-12.1982543436608));
#27990=CARTESIAN_POINT('Origin',(0.206375791602559,-16.2288732699618,-12.1982543436608));
#27991=CARTESIAN_POINT('Ctrl Pts',(-4.99997666922215,-21.7249999972923,
-10.8899189904778));
#27992=CARTESIAN_POINT('Ctrl Pts',(-4.99998234101381,-21.6600944959454,
-10.8899160716605));
#27993=CARTESIAN_POINT('Ctrl Pts',(-4.99873301488811,-21.595304502466,-10.8906091337332));
#27994=CARTESIAN_POINT('Ctrl Pts',(-4.99623155731798,-21.530911809512,-10.8919978308171));
#27995=CARTESIAN_POINT('Ctrl Pts',(-4.98793986214795,-21.3174664216997,
-10.8966010081967));
#27996=CARTESIAN_POINT('Ctrl Pts',(-4.96617998392237,-21.106513506024,-10.9087478277567));
#27997=CARTESIAN_POINT('Ctrl Pts',(-4.93119702679394,-20.8980705932228,
-10.9278316856883));
#27998=CARTESIAN_POINT('Ctrl Pts',(-4.92101994987409,-20.8374313639778,
-10.9333834716446));
#27999=CARTESIAN_POINT('Ctrl Pts',(-4.90972407973498,-20.7770045122468,
-10.9395221982223));
#28000=CARTESIAN_POINT('Ctrl Pts',(-4.89731618003943,-20.7167903516954,
-10.9462325729994));
#28001=CARTESIAN_POINT('Ctrl Pts',(-4.88614901395925,-20.6625973337186,
-10.952271940776));
#28002=CARTESIAN_POINT('Ctrl Pts',(-4.87407481030087,-20.608546748349,-10.9587774566803));
#28003=CARTESIAN_POINT('Ctrl Pts',(-4.86109898192199,-20.5546510400728,
-10.9657377511903));
#28004=CARTESIAN_POINT('Ctrl Pts',(-4.83174926734893,-20.432745631922,-10.9814810741789));
#28005=CARTESIAN_POINT('Ctrl Pts',(-4.79756722607834,-20.3114529823632,
-10.9996494442541));
#28006=CARTESIAN_POINT('Ctrl Pts',(-4.75898711148544,-20.1918167377945,
-11.0198136305987));
#28007=CARTESIAN_POINT('Ctrl Pts',(-4.720655625942,-20.0729514874565,-11.0398478691053));
#28008=CARTESIAN_POINT('Ctrl Pts',(-4.67798326007562,-19.9557228113236,
-11.0618515925471));
#28009=CARTESIAN_POINT('Ctrl Pts',(-4.63143601061823,-19.8411294983212,
-11.0853880635562));
#28010=CARTESIAN_POINT('Ctrl Pts',(-4.61955732598353,-19.8118857117974,
-11.091394483265));
#28011=CARTESIAN_POINT('Ctrl Pts',(-4.60742646402923,-19.7828133652514,
-11.0975006724954));
#28012=CARTESIAN_POINT('Ctrl Pts',(-4.5950515077976,-19.7539286231138,-11.1036992902712));
#28013=CARTESIAN_POINT('Ctrl Pts',(-4.5765422227149,-19.7107255671386,-11.1129705944588));
#28014=CARTESIAN_POINT('Ctrl Pts',(-4.55746124119458,-19.6678824271789,
-11.1224592641773));
#28015=CARTESIAN_POINT('Ctrl Pts',(-4.53783003076107,-19.625452757179,-11.1321433191472));
#28016=CARTESIAN_POINT('Ctrl Pts',(-4.47768226052557,-19.4954531297508,
-11.1618141494433));
#28017=CARTESIAN_POINT('Ctrl Pts',(-4.41224167944152,-19.3685202707715,
-11.1933951840664));
#28018=CARTESIAN_POINT('Ctrl Pts',(-4.34153092407304,-19.244728467047,-11.2264766384861));
#28019=CARTESIAN_POINT('Ctrl Pts',(-4.27166647685399,-19.122418276859,-11.2591621544898));
#28020=CARTESIAN_POINT('Ctrl Pts',(-4.19665731093853,-19.0031743253473,
-11.2933118568733));
#28021=CARTESIAN_POINT('Ctrl Pts',(-4.11656733346088,-18.887044107912,-11.3285184255984));
#28022=CARTESIAN_POINT('Ctrl Pts',(-4.09415340249297,-18.8545439779474,
-11.3383713138857));
#28023=CARTESIAN_POINT('Ctrl Pts',(-4.07133677950163,-18.8222802633444,
-11.3483085153344));
#28024=CARTESIAN_POINT('Ctrl Pts',(-4.04811668956903,-18.7902510724644,
-11.3583218371279));
#28025=CARTESIAN_POINT('Ctrl Pts',(-3.95293798793259,-18.6589640356236,
-11.3993662503985));
#28026=CARTESIAN_POINT('Ctrl Pts',(-3.85068360691524,-18.5315166896151,
-11.4417695249564));
#28027=CARTESIAN_POINT('Ctrl Pts',(-3.74359091922971,-18.4105578102084,
-11.4840110886132));
#28028=CARTESIAN_POINT('Ctrl Pts',(-3.65812755471859,-18.3140287845111,
-11.5177211974015));
#28029=CARTESIAN_POINT('Ctrl Pts',(-3.56928502721573,-18.221183434314,-11.5514631987063));
#28030=CARTESIAN_POINT('Ctrl Pts',(-3.47704521778017,-18.1319269682117,
-11.5849605673345));
#28031=CARTESIAN_POINT('Ctrl Pts',(-3.45368649324617,-18.1093237428005,
-11.5934434101676));
#28032=CARTESIAN_POINT('Ctrl Pts',(-3.43011673544645,-18.0869573014828,
-11.6019082045496));
#28033=CARTESIAN_POINT('Ctrl Pts',(-3.40633409590771,-18.0648240442483,
-11.610351129418));
#28034=CARTESIAN_POINT('Ctrl Pts',(-3.31351007565654,-17.9784375893547,
-11.6433039994176));
#28035=CARTESIAN_POINT('Ctrl Pts',(-3.21717077395441,-17.8953870071991,
-11.6760079177476));
#28036=CARTESIAN_POINT('Ctrl Pts',(-3.11744419797313,-17.8158628991426,
-11.7081356286851));
#28037=CARTESIAN_POINT('Ctrl Pts',(-3.01974880409736,-17.7379584992096,
-11.7396089781255));
#28038=CARTESIAN_POINT('Ctrl Pts',(-2.91880218367213,-17.6634380085559,
-11.7705299357143));
#28039=CARTESIAN_POINT('Ctrl Pts',(-2.81469354777058,-17.5925182788626,
-11.8005824061336));
#28040=CARTESIAN_POINT('Ctrl Pts',(-2.77718074687106,-17.5669642248997,
-11.8114110211627));
#28041=CARTESIAN_POINT('Ctrl Pts',(-2.73925715163687,-17.5418780564676,
-11.822126755195));
#28042=CARTESIAN_POINT('Ctrl Pts',(-2.70092611220132,-17.5172712981393,
-11.8327143231594));
#28043=CARTESIAN_POINT('Ctrl Pts',(-2.67904116891535,-17.5032221745467,
-11.838759249878));
#28044=CARTESIAN_POINT('Ctrl Pts',(-2.65704081181229,-17.4893405226794,
-11.844757694435));
#28045=CARTESIAN_POINT('Ctrl Pts',(-2.63492637900982,-17.475627931408,-11.8507069466921));
#28046=CARTESIAN_POINT('Ctrl Pts',(-2.52129478005667,-17.4051678980948,
-11.8812762609759));
#28047=CARTESIAN_POINT('Ctrl Pts',(-2.40539761260767,-17.339541832115,-11.9103691828862));
#28048=CARTESIAN_POINT('Ctrl Pts',(-2.28706438300499,-17.2786609863284,
-11.9378018380373));
#28049=CARTESIAN_POINT('Ctrl Pts',(-2.17007764129556,-17.2184728903471,
-11.9649223430159));
#28050=CARTESIAN_POINT('Ctrl Pts',(-2.05070998244525,-17.1629227076627,
-11.990420463892));
#28051=CARTESIAN_POINT('Ctrl Pts',(-1.9287742755276,-17.111967992304,-12.0141038891066));
#28052=CARTESIAN_POINT('Ctrl Pts',(-1.88971247615946,-17.0956447764183,
-12.0216908152619));
#28053=CARTESIAN_POINT('Ctrl Pts',(-1.85038696231078,-17.0797934904909,
-12.0290913799705));
#28054=CARTESIAN_POINT('Ctrl Pts',(-1.81079108152958,-17.0644136789109,
-12.0362988569225));
#28055=CARTESIAN_POINT('Ctrl Pts',(-1.79349000894213,-17.0576936052245,
-12.039448100719));
#28056=CARTESIAN_POINT('Ctrl Pts',(-1.77613909683667,-17.051064243726,-12.0425602292707));
#28057=CARTESIAN_POINT('Ctrl Pts',(-1.75873817661222,-17.0445256622699,
-12.0456346167024));
#28058=CARTESIAN_POINT('Ctrl Pts',(-1.57559193939589,-16.9757065093197,
-12.0779928186019));
#28059=CARTESIAN_POINT('Ctrl Pts',(-1.38618282670759,-16.9170929190887,
-12.106111409062));
#28060=CARTESIAN_POINT('Ctrl Pts',(-1.19382360958483,-16.8697505421426,
-12.1290510506316));
#28061=CARTESIAN_POINT('Ctrl Pts',(-1.07428552506051,-16.840330495931,-12.1433064674186));
#28062=CARTESIAN_POINT('Ctrl Pts',(-0.953608844790518,-16.8152636561332,
-12.1555615926741));
#28063=CARTESIAN_POINT('Ctrl Pts',(-0.832596678325463,-16.794811151152,
-12.1655876027153));
#28064=CARTESIAN_POINT('Ctrl Pts',(-0.822547136999614,-16.7931126583473,
-12.1664202198413));
#28065=CARTESIAN_POINT('Ctrl Pts',(-0.812493307657583,-16.7914456570965,
-12.1672376753802));
#28066=CARTESIAN_POINT('Ctrl Pts',(-0.80243580320674,-16.789810359935,-12.1680398086835));
#28067=CARTESIAN_POINT('Ctrl Pts',(-0.695016219010128,-16.772344502277,
-12.1766070259623));
#28068=CARTESIAN_POINT('Ctrl Pts',(-0.586813990430978,-16.7583188314844,
-12.1835103776808));
#28069=CARTESIAN_POINT('Ctrl Pts',(-0.477998355044125,-16.7478515832007,
-12.1886740113227));
#28070=CARTESIAN_POINT('Ctrl Pts',(-0.368071624253781,-16.7372774558695,
-12.1938903698289));
#28071=CARTESIAN_POINT('Ctrl Pts',(-0.257518864835462,-16.7303350234902,
-12.1973311475917));
#28072=CARTESIAN_POINT('Ctrl Pts',(-0.146521659500288,-16.7270973793117,
-12.1989418461153));
#28073=CARTESIAN_POINT('Ctrl Pts',(-0.0355244541651161,-16.7238597351332,
-12.200552544639));
#28074=CARTESIAN_POINT('Ctrl Pts',(0.0759172118544166,-16.7243270033065,
-12.2003330628352));
#28075=CARTESIAN_POINT('Ctrl Pts',(0.187614356002326,-16.7285211545107,
-12.1982543436608));
#28076=CARTESIAN_POINT('Origin',(0.,-0.999999999999945,0.));
#28077=CARTESIAN_POINT('',(1.68059064192457,0.,-11.5786706963397));
#28078=CARTESIAN_POINT('',(-1.68059064192455,0.,-11.5786706963397));
#28079=CARTESIAN_POINT('Origin',(0.,0.,0.));
#28080=CARTESIAN_POINT('',(3.46944695195361E-15,-0.848960155852397,-12.5489601558525));
#28081=CARTESIAN_POINT('Ctrl Pts',(1.68059064192456,5.84411658722412E-15,
-11.5786706963397));
#28082=CARTESIAN_POINT('Ctrl Pts',(0.869714200879421,-0.346830427858442,
-12.0468304278567));
#28083=CARTESIAN_POINT('Ctrl Pts',(2.62089735138893E-11,-0.848960155837265,
-12.5489601558373));
#28084=CARTESIAN_POINT('Ctrl Pts',(-2.62073916106111E-11,-0.84896015583726,
-12.5489601558373));
#28085=CARTESIAN_POINT('Ctrl Pts',(-0.869714200879411,-0.346830427858444,
-12.0468304278567));
#28086=CARTESIAN_POINT('Ctrl Pts',(-1.68059064192454,1.5245521531889E-15,
-11.5786706963397));
#28087=CARTESIAN_POINT('Origin',(0.,-21.725,-21.5));
#28088=CARTESIAN_POINT('',(5.00001172195141,-21.7250000023451,-10.8899050240605));
#28089=CARTESIAN_POINT('Ctrl Pts',(5.00002344390285,-21.725000004566,-10.8899064672807));
#28090=CARTESIAN_POINT('Ctrl Pts',(5.00001152141201,-21.7882748865493,-10.8899059311929));
#28091=CARTESIAN_POINT('Ctrl Pts',(4.99879927122167,-21.8516587474073,-10.8905724964452));
#28092=CARTESIAN_POINT('Ctrl Pts',(4.99638310479926,-21.9151469697699,-10.8919139762305));
#28093=CARTESIAN_POINT('Ctrl Pts',(4.990060963821,-22.0812702502336,-10.8954240921909));
#28094=CARTESIAN_POINT('Ctrl Pts',(4.97522566801055,-22.2490604010701,-10.9036628526843));
#28095=CARTESIAN_POINT('Ctrl Pts',(4.95239190657507,-22.4133417782704,-10.9161966077095));
#28096=CARTESIAN_POINT('Ctrl Pts',(4.93706818544299,-22.5235908941913,-10.9246080018325));
#28097=CARTESIAN_POINT('Ctrl Pts',(4.91817280124604,-22.6326091834789,-10.9349360548822));
#28098=CARTESIAN_POINT('Ctrl Pts',(4.89581131018126,-22.7404136161556,-10.947035666435));
#28099=CARTESIAN_POINT('Ctrl Pts',(4.88482334405882,-22.7933864456807,-10.9529811609215));
#28100=CARTESIAN_POINT('Ctrl Pts',(4.87299763343813,-22.8460709434397,-10.9593547795652));
#28101=CARTESIAN_POINT('Ctrl Pts',(4.86034588878338,-22.8984725567251,-10.9661397284499));
#28102=CARTESIAN_POINT('Ctrl Pts',(4.79422159663562,-23.1723493761247,-11.0016012362895));
#28103=CARTESIAN_POINT('Ctrl Pts',(4.70571139778224,-23.4385476398574,-11.048296021071));
#28104=CARTESIAN_POINT('Ctrl Pts',(4.5945753052774,-23.6973148396108,-11.1039144219712));
#28105=CARTESIAN_POINT('Ctrl Pts',(4.57643367394708,-23.7395554747861,-11.1129934574274));
#28106=CARTESIAN_POINT('Ctrl Pts',(4.55767872580587,-23.7816218623763,-11.1223160148244));
#28107=CARTESIAN_POINT('Ctrl Pts',(4.53831397330642,-23.8235009601411,-11.1318694619704));
#28108=CARTESIAN_POINT('Ctrl Pts',(4.49243330473491,-23.9227245884666,-11.1545043261255));
#28109=CARTESIAN_POINT('Ctrl Pts',(4.44358835177731,-24.0198695778208,-11.1781944567248));
#28110=CARTESIAN_POINT('Ctrl Pts',(4.39196253677333,-24.1147721393631,-11.2026884744858));
#28111=CARTESIAN_POINT('Ctrl Pts',(4.38586624978507,-24.1259788050794,-11.2055808755405));
#28112=CARTESIAN_POINT('Ctrl Pts',(4.37973123224749,-24.1371542364042,-11.2084844733256));
#28113=CARTESIAN_POINT('Ctrl Pts',(4.37355782324247,-24.1482981914757,-11.211398844494));
#28114=CARTESIAN_POINT('Ctrl Pts',(4.30980965679331,-24.2633734606211,-11.241493370579));
#28115=CARTESIAN_POINT('Ctrl Pts',(4.24191254319682,-24.3752010240399,-11.2727586116446));
#28116=CARTESIAN_POINT('Ctrl Pts',(4.16995158407907,-24.4839330077148,-11.3048712900011));
#28117=CARTESIAN_POINT('Ctrl Pts',(4.15102174685418,-24.5125357219829,-11.3133187562606));
#28118=CARTESIAN_POINT('Ctrl Pts',(4.13181047583863,-24.540924060519,-11.321824927182));
#28119=CARTESIAN_POINT('Ctrl Pts',(4.11231885863813,-24.5691004415348,-11.330384030271));
#28120=CARTESIAN_POINT('Ctrl Pts',(4.09072627107986,-24.6003139097607,-11.3398657054427));
#28121=CARTESIAN_POINT('Ctrl Pts',(4.06879087060822,-24.631265442764,-11.349411600643));
#28122=CARTESIAN_POINT('Ctrl Pts',(4.04651664935594,-24.6619547164646,-11.3590125548681));
#28123=CARTESIAN_POINT('Ctrl Pts',(3.95198509136906,-24.7921996675026,-11.3997589024409));
#28124=CARTESIAN_POINT('Ctrl Pts',(3.85121377604902,-24.9178494050859,-11.4415547761407));
#28125=CARTESIAN_POINT('Ctrl Pts',(3.74406673020293,-25.0389046938329,-11.4838238526989));
#28126=CARTESIAN_POINT('Ctrl Pts',(3.65760774291518,-25.1365865066,-11.5179315737653));
#28127=CARTESIAN_POINT('Ctrl Pts',(3.56661037535839,-25.2315979421455,-11.5524774355491));
#28128=CARTESIAN_POINT('Ctrl Pts',(3.47237289989047,-25.32257642859,-11.5866541000274));
#28129=CARTESIAN_POINT('Ctrl Pts',(3.44980057505032,-25.3443681408498,-11.5948402995061));
#28130=CARTESIAN_POINT('Ctrl Pts',(3.42703985515985,-25.365930928998,-11.6030062755313));
#28131=CARTESIAN_POINT('Ctrl Pts',(3.40410824423346,-25.3872461770815,-11.6111410187316));
#28132=CARTESIAN_POINT('Ctrl Pts',(3.18470052889287,-25.5911886693441,-11.6889735541861));
#28133=CARTESIAN_POINT('Ctrl Pts',(2.94900150199431,-25.7739299727301,-11.7643260370852));
#28134=CARTESIAN_POINT('Ctrl Pts',(2.696322025512,-25.9356885348437,-11.8339822109817));
#28135=CARTESIAN_POINT('Ctrl Pts',(2.67583165664485,-25.9488059144238,-11.8396307928011));
#28136=CARTESIAN_POINT('Ctrl Pts',(2.65522784224586,-25.9617864319314,-11.8452425778975));
#28137=CARTESIAN_POINT('Ctrl Pts',(2.63451048821384,-25.9746299235927,-11.850815697453));
#28138=CARTESIAN_POINT('Ctrl Pts',(2.49198588806835,-26.0629864536144,-11.8891558559009));
#28139=CARTESIAN_POINT('Ctrl Pts',(2.34348714532903,-26.1448951794979,-11.925708481326));
#28140=CARTESIAN_POINT('Ctrl Pts',(2.19098226277494,-26.2192493576819,-11.9595228911452));
#28141=CARTESIAN_POINT('Ctrl Pts',(2.06371540788928,-26.2812986655245,-11.9877413554686));
#28142=CARTESIAN_POINT('Ctrl Pts',(1.93366011679675,-26.3380870977829,-12.0140526922932));
#28143=CARTESIAN_POINT('Ctrl Pts',(1.80197549472834,-26.3889932854301,-12.0379121302175));
#28144=CARTESIAN_POINT('Ctrl Pts',(1.78615368929159,-26.3951096244819,-12.0407788232203));
#28145=CARTESIAN_POINT('Ctrl Pts',(1.77030548911759,-26.4011421911994,-12.0436108293463));
#28146=CARTESIAN_POINT('Ctrl Pts',(1.75443286313541,-26.4070898465095,-12.0464071869036));
#28147=CARTESIAN_POINT('Ctrl Pts',(1.58749408431246,-26.4696437248303,-12.0758176018078));
#28148=CARTESIAN_POINT('Ctrl Pts',(1.41707113919231,-26.5234254396691,-12.1015564914957));
#28149=CARTESIAN_POINT('Ctrl Pts',(1.24311481949365,-26.5680679342181,-12.1231373121445));
#28150=CARTESIAN_POINT('Ctrl Pts',(1.10701123067326,-26.6029962641146,-12.1400221666015));
#28151=CARTESIAN_POINT('Ctrl Pts',(0.968744958017119,-26.6323308041622,
-12.1543618446964));
#28152=CARTESIAN_POINT('Ctrl Pts',(0.82829974493686,-26.655915398572,-12.1659311274838));
#28153=CARTESIAN_POINT('Ctrl Pts',(0.819544689390747,-26.6573856119709,
-12.1666523319394));
#28154=CARTESIAN_POINT('Ctrl Pts',(0.810782077925004,-26.6588333343054,
-12.1673626945561));
#28155=CARTESIAN_POINT('Ctrl Pts',(0.802011826845791,-26.6602585575249,
-12.1680621755967));
#28156=CARTESIAN_POINT('Ctrl Pts',(0.686607364415905,-26.6790125382266,
-12.1772663856868));
#28157=CARTESIAN_POINT('Ctrl Pts',(0.570129714195444,-26.6936648092245,
-12.1844828834562));
#28158=CARTESIAN_POINT('Ctrl Pts',(0.453284493692702,-26.704253353433,-12.1897098761392));
#28159=CARTESIAN_POINT('Ctrl Pts',(0.338620856724135,-26.7146442019755,
-12.1948392771438));
#28160=CARTESIAN_POINT('Ctrl Pts',(0.223601703868209,-26.7211215084667,
-12.1980527358992));
#28161=CARTESIAN_POINT('Ctrl Pts',(0.108892707969018,-26.7236778818544,
-12.1993273015262));
#28162=CARTESIAN_POINT('Ctrl Pts',(0.00742336080110954,-26.7259392000425,
-12.200454757495));
#28163=CARTESIAN_POINT('Ctrl Pts',(-0.0938039899970676,-26.7251318549737,
-12.200064783988));
#28164=CARTESIAN_POINT('Ctrl Pts',(-0.194315056429422,-26.7212227391145,
-12.19812741396));
#28165=CARTESIAN_POINT('',(-4.99999160226712,-21.72500000341,10.8899098036299));
#28166=CARTESIAN_POINT('',(-5.,-21.725,-21.5));
#28167=CARTESIAN_POINT('Origin',(-3.89307326486085,-21.3390068413815,11.5111137315767));
#28168=CARTESIAN_POINT('Ctrl Pts',(4.99980122230293,-21.6804159506306,10.890014011117));
#28169=CARTESIAN_POINT('Ctrl Pts',(4.99681149794833,-21.3451384759755,10.8916749023389));
#28170=CARTESIAN_POINT('Ctrl Pts',(4.96051653026192,-21.0171256611318,10.9120450197627));
#28171=CARTESIAN_POINT('Ctrl Pts',(4.89293081575696,-20.695811954881,10.94859196248));
#28172=CARTESIAN_POINT('Ctrl Pts',(4.89289834722306,-20.6956575940809,10.9486095198242));
#28173=CARTESIAN_POINT('Ctrl Pts',(4.89286587140735,-20.6955032348325,10.9486270809002));
#28174=CARTESIAN_POINT('Ctrl Pts',(4.89283338830974,-20.6953488771359,10.9486446457078));
#28175=CARTESIAN_POINT('Ctrl Pts',(4.86683621968048,-20.5718119190493,10.9627022725655));
#28176=CARTESIAN_POINT('Ctrl Pts',(4.83616535482728,-20.4492430359115,10.9791550395257));
#28177=CARTESIAN_POINT('Ctrl Pts',(4.80081433199506,-20.3277880416923,10.9978254612168));
#28178=CARTESIAN_POINT('Ctrl Pts',(4.79028605113857,-20.2916161805093,11.0033859069275));
#28179=CARTESIAN_POINT('Ctrl Pts',(4.77934296232174,-20.2555430495807,11.0091429015769));
#28180=CARTESIAN_POINT('Ctrl Pts',(4.76798568777015,-20.2195723261415,11.0150913877129));
#28181=CARTESIAN_POINT('Ctrl Pts',(4.73197766638454,-20.1055278365969,11.0339509490475));
#28182=CARTESIAN_POINT('Ctrl Pts',(4.69162361143881,-19.9922070920438,11.054822610137));
#28183=CARTESIAN_POINT('Ctrl Pts',(4.64765781272916,-19.8813291049973,11.0771437849085));
#28184=CARTESIAN_POINT('Ctrl Pts',(4.63098022901674,-19.839269664134,11.0856108950654));
#28185=CARTESIAN_POINT('Ctrl Pts',(4.61378318693029,-19.7975612928432,11.0942865168028));
#28186=CARTESIAN_POINT('Ctrl Pts',(4.5961074869497,-19.7562958657012,11.1031398492434));
#28187=CARTESIAN_POINT('Ctrl Pts',(4.59601302641415,-19.7560753395353,11.1031871622508));
#28188=CARTESIAN_POINT('Ctrl Pts',(4.59591855188769,-19.7558548240601,11.1032344805497));
#28189=CARTESIAN_POINT('Ctrl Pts',(4.59582406337146,-19.7556343192758,11.1032818041376));
#28190=CARTESIAN_POINT('Ctrl Pts',(4.50148136442582,-19.535469824063,11.1505323610586));
#28191=CARTESIAN_POINT('Ctrl Pts',(4.39280939934476,-19.3250607724011,11.2032466660903));
#28192=CARTESIAN_POINT('Ctrl Pts',(4.27010858683285,-19.1237335109746,11.2595416663626));
#28193=CARTESIAN_POINT('Ctrl Pts',(4.22574734402706,-19.0509456675633,11.2798945566549));
#28194=CARTESIAN_POINT('Ctrl Pts',(4.1795520246957,-18.9793451745005,11.3007157428127));
#28195=CARTESIAN_POINT('Ctrl Pts',(4.13153565263822,-18.9089010457424,11.3219170106647));
#28196=CARTESIAN_POINT('Ctrl Pts',(4.13080975140498,-18.9078360864848,11.3222375268933));
#28197=CARTESIAN_POINT('Ctrl Pts',(4.13008343381006,-18.9067713912948,11.3225581300807));
#28198=CARTESIAN_POINT('Ctrl Pts',(4.12935669989677,-18.9057069600664,11.3228788199229));
#28199=CARTESIAN_POINT('Ctrl Pts',(3.99139364898032,-18.7036355043609,11.3837585287321));
#28200=CARTESIAN_POINT('Ctrl Pts',(3.8371376032085,-18.510168652598,11.4481955970778));
#28201=CARTESIAN_POINT('Ctrl Pts',(3.67050413426203,-18.3298890659559,11.5125041611507));
#28202=CARTESIAN_POINT('Ctrl Pts',(3.61935966431457,-18.2745562210031,11.532242257245));
#28203=CARTESIAN_POINT('Ctrl Pts',(3.56704882610507,-18.220465779807,11.551968361796));
#28204=CARTESIAN_POINT('Ctrl Pts',(3.51368401016484,-18.1677506558258,11.5715760913822));
#28205=CARTESIAN_POINT('Ctrl Pts',(3.51140243577175,-18.165496858546,11.5724144057836));
#28206=CARTESIAN_POINT('Ctrl Pts',(3.50911892302814,-18.1632455637268,11.5732525081862));
#28207=CARTESIAN_POINT('Ctrl Pts',(3.5068334807527,-18.1609967819498,11.5740903902315));
#28208=CARTESIAN_POINT('Ctrl Pts',(3.28058390602085,-17.9383764488207,11.6570373359732));
#28209=CARTESIAN_POINT('Ctrl Pts',(3.03441230305267,-17.7380727100291,11.7384462854316));
#28210=CARTESIAN_POINT('Ctrl Pts',(2.76690911959257,-17.560361184534,11.8142501978774));
#28211=CARTESIAN_POINT('Ctrl Pts',(2.76267967067482,-17.5575514167792,11.8154487210923));
#28212=CARTESIAN_POINT('Ctrl Pts',(2.75844487664652,-17.554747289089,11.8166458456229));
#28213=CARTESIAN_POINT('Ctrl Pts',(2.75420473161427,-17.5519488025721,11.8178415553647));
#28214=CARTESIAN_POINT('Ctrl Pts',(2.61812893871101,-17.4621390746436,11.8562145709011));
#28215=CARTESIAN_POINT('Ctrl Pts',(2.4765031260948,-17.3783234220784,11.8930824769717));
#28216=CARTESIAN_POINT('Ctrl Pts',(2.33205830830434,-17.3021610874157,11.9272556062802));
#28217=CARTESIAN_POINT('Ctrl Pts',(2.1934549885892,-17.2290788364705,11.9600467388363));
#28218=CARTESIAN_POINT('Ctrl Pts',(2.0516181351631,-17.1625961247258,11.9905469912575));
#28219=CARTESIAN_POINT('Ctrl Pts',(1.90647238682508,-17.1027317310734,12.018406332931));
#28220=CARTESIAN_POINT('Ctrl Pts',(1.90049463025599,-17.1002662453358,12.0195537062755));
#28221=CARTESIAN_POINT('Ctrl Pts',(1.89451126025318,-17.0978119855393,12.0206965994529));
#28222=CARTESIAN_POINT('Ctrl Pts',(1.88852227143256,-17.0953689531127,12.0218349879028));
#28223=CARTESIAN_POINT('Ctrl Pts',(1.74366730051123,-17.0362796140396,12.0493690559644));
#28224=CARTESIAN_POINT('Ctrl Pts',(1.59552621727336,-16.9837569593759,12.0742699322544));
#28225=CARTESIAN_POINT('Ctrl Pts',(1.44393008546716,-16.9380315409714,12.0961660723804));
#28226=CARTESIAN_POINT('Ctrl Pts',(1.4372414835026,-16.9360140810288,12.0971321561724));
#28227=CARTESIAN_POINT('Ctrl Pts',(1.43054599105914,-16.9340098044762,12.0980924221045));
#28228=CARTESIAN_POINT('Ctrl Pts',(1.42384361790784,-16.9320187407269,12.0990468327269));
#28229=CARTESIAN_POINT('Ctrl Pts',(1.30167033908194,-16.8957249114949,12.1164441743029));
#28230=CARTESIAN_POINT('Ctrl Pts',(1.17692640634316,-16.8638307026676,12.1318926790276));
#28231=CARTESIAN_POINT('Ctrl Pts',(1.05166758402415,-16.8368632173258,12.145026869394));
#28232=CARTESIAN_POINT('Ctrl Pts',(1.02161405873619,-16.8303928706655,12.1481781741485));
#28233=CARTESIAN_POINT('Ctrl Pts',(0.991530972260571,-16.824205939237,12.1511963433226));
#28234=CARTESIAN_POINT('Ctrl Pts',(0.961446789444828,-16.8183093004312,
12.1540765186724));
#28235=CARTESIAN_POINT('Ctrl Pts',(0.954305426975421,-16.8169095603977,
12.154760212701));
#28236=CARTESIAN_POINT('Ctrl Pts',(0.94716354233454,-16.8155260870371,12.1554361899411));
#28237=CARTESIAN_POINT('Ctrl Pts',(0.9400214921796,-16.8141589728088,12.1561043861852));
#28238=CARTESIAN_POINT('Ctrl Pts',(0.740888611067521,-16.7760414310389,
12.1747348690792));
#28239=CARTESIAN_POINT('Ctrl Pts',(0.540319367334083,-16.7500849358455,
12.1875483549967));
#28240=CARTESIAN_POINT('Ctrl Pts',(0.338393099035631,-16.7364089056273,
12.1943261791738));
#28241=CARTESIAN_POINT('Ctrl Pts',(0.218276230812764,-16.7282736494599,
12.1983580023754));
#28242=CARTESIAN_POINT('Ctrl Pts',(0.0976792709987591,-16.7244829836586,
12.2002544963976));
#28243=CARTESIAN_POINT('Ctrl Pts',(-0.0233802237688804,-16.7250541700989,
12.1999734032215));
#28244=CARTESIAN_POINT('Ctrl Pts',(-0.0310072465875391,-16.7250901561405,
12.1999556937137));
#28245=CARTESIAN_POINT('Ctrl Pts',(-0.038636314214975,-16.7251434546806,
12.1999293526452));
#28246=CARTESIAN_POINT('Ctrl Pts',(-0.0462674058931988,-16.7252140718672,
12.1998943671571));
#28247=CARTESIAN_POINT('Ctrl Pts',(-0.18722183044295,-16.7265184468272,
12.1992481477764));
#28248=CARTESIAN_POINT('Ctrl Pts',(-0.329643856273163,-16.7338997864519,
12.1955863398144));
#28249=CARTESIAN_POINT('Ctrl Pts',(-0.470516177416762,-16.7471945727973,
12.1890167310796));
#28250=CARTESIAN_POINT('Ctrl Pts',(-0.48794375998246,-16.7488392960818,
12.1882039922979));
#28251=CARTESIAN_POINT('Ctrl Pts',(-0.50534763266374,-16.7505744639994,
12.1873467792465));
#28252=CARTESIAN_POINT('Ctrl Pts',(-0.522722097817875,-16.752399717777,
12.186445319834));
#28253=CARTESIAN_POINT('Ctrl Pts',(-0.530415524002231,-16.7532079415169,
12.1860461529309));
#28254=CARTESIAN_POINT('Ctrl Pts',(-0.538103390625485,-16.7540338501271,
12.1856383264121));
#28255=CARTESIAN_POINT('Ctrl Pts',(-0.54578521940695,-16.7548774165665,
12.1852218592229));
#28256=CARTESIAN_POINT('Ctrl Pts',(-0.703274852129899,-16.7721718620023,
12.1766836235324));
#28257=CARTESIAN_POINT('Ctrl Pts',(-0.85856929506714,-16.7967821156056,
12.1645667163415));
#28258=CARTESIAN_POINT('Ctrl Pts',(-1.01171262550948,-16.8284257973864,
12.1491355438321));
#28259=CARTESIAN_POINT('Ctrl Pts',(-1.01938094710419,-16.8300102864244,
12.1483628611887));
#28260=CARTESIAN_POINT('Ctrl Pts',(-1.02704392334188,-16.8316124164775,
12.1475818645961));
#28261=CARTESIAN_POINT('Ctrl Pts',(-1.03470156646483,-16.83323215306,12.1467925870816));
#28262=CARTESIAN_POINT('Ctrl Pts',(-1.34782292335014,-16.8994632516321,
12.1145189955418));
#28263=CARTESIAN_POINT('Ctrl Pts',(-1.65208339548054,-16.9949098339779,
12.0684105022407));
#28264=CARTESIAN_POINT('Ctrl Pts',(-1.94762155723166,-17.1199183744877,
12.0104202812587));
#28265=CARTESIAN_POINT('Ctrl Pts',(-1.95561400152696,-17.1232990674938,
12.0088520113333));
#28266=CARTESIAN_POINT('Ctrl Pts',(-1.96360003997595,-17.1267013710748,
12.0072750551016));
#28267=CARTESIAN_POINT('Ctrl Pts',(-1.97157967297179,-17.1301252908132,
12.0056894514984));
#28268=CARTESIAN_POINT('Ctrl Pts',(-2.24657951621896,-17.248122871886,11.9510452413496));
#28269=CARTESIAN_POINT('Ctrl Pts',(-2.50646165958052,-17.3887242213049,
11.8876066014172));
#28270=CARTESIAN_POINT('Ctrl Pts',(-2.75051310584763,-17.5495107130101,
11.8188822479445));
#28271=CARTESIAN_POINT('Ctrl Pts',(-2.76764198236856,-17.560795595787,11.814058793781));
#28272=CARTESIAN_POINT('Ctrl Pts',(-2.78469289361425,-17.5721799027812,
11.8092092914112));
#28273=CARTESIAN_POINT('Ctrl Pts',(-2.80166560080175,-17.5836627944812,
11.804334948629));
#28274=CARTESIAN_POINT('Ctrl Pts',(-2.80984000984178,-17.5891931941211,
11.8019873636937));
#28275=CARTESIAN_POINT('Ctrl Pts',(-2.81799647167743,-17.594746591815,11.7996339650656));
#28276=CARTESIAN_POINT('Ctrl Pts',(-2.82613496059901,-17.6003228993675,
11.797274885726));
#28277=CARTESIAN_POINT('Ctrl Pts',(-2.95920726957285,-17.6915010196188,
11.758701615208));
#28278=CARTESIAN_POINT('Ctrl Pts',(-3.08768365836285,-17.7889671040843,
11.7185499987111));
#28279=CARTESIAN_POINT('Ctrl Pts',(-3.21161242246995,-17.8928275550485,
11.6773084639027));
#28280=CARTESIAN_POINT('Ctrl Pts',(-3.32656816409712,-17.9891680233194,
11.6390530092155));
#28281=CARTESIAN_POINT('Ctrl Pts',(-3.43810167779714,-18.0915480029184,
11.5996663706253));
#28282=CARTESIAN_POINT('Ctrl Pts',(-3.5442103899849,-18.1981656868409,11.5603064707464));
#28283=CARTESIAN_POINT('Ctrl Pts',(-3.55253769572624,-18.2065329361755,
11.5572175451202));
#28284=CARTESIAN_POINT('Ctrl Pts',(-3.56083171048927,-18.2149264067726,
11.5541287493587));
#28285=CARTESIAN_POINT('Ctrl Pts',(-3.56909146879911,-18.2233452358416,
11.5510406406348));
#28286=CARTESIAN_POINT('Ctrl Pts',(-3.74708806780088,-18.4047697867366,
11.4844923435088));
#28287=CARTESIAN_POINT('Ctrl Pts',(-3.90975366927737,-18.597920472388,11.4181748287074));
#28288=CARTESIAN_POINT('Ctrl Pts',(-4.05749346642025,-18.8031764790736,
11.3542801320666));
#28289=CARTESIAN_POINT('Ctrl Pts',(-4.09019119673731,-18.8486036806967,
11.3401389757914));
#28290=CARTESIAN_POINT('Ctrl Pts',(-4.12215767289834,-18.8946239569954,
11.326116534228));
#28291=CARTESIAN_POINT('Ctrl Pts',(-4.15339703200001,-18.9412416390385,
11.3122366565339));
#28292=CARTESIAN_POINT('Ctrl Pts',(-4.16101062698528,-18.9526032085596,
11.3088538801183));
#28293=CARTESIAN_POINT('Ctrl Pts',(-4.16858130744644,-18.9640006749311,
11.3054794637819));
#28294=CARTESIAN_POINT('Ctrl Pts',(-4.17610909058629,-18.9754340590648,
11.3021137712519));
#28295=CARTESIAN_POINT('Ctrl Pts',(-4.27733878375571,-19.1291842330849,
11.2568536972321));
#28296=CARTESIAN_POINT('Ctrl Pts',(-4.37098435674311,-19.2903091486333,
11.2130472316835));
#28297=CARTESIAN_POINT('Ctrl Pts',(-4.45554758708343,-19.4563285341691,
11.1722457075528));
#28298=CARTESIAN_POINT('Ctrl Pts',(-4.51249022059306,-19.5681215793025,
11.1447710447962));
#28299=CARTESIAN_POINT('Ctrl Pts',(-4.56531514750588,-19.6821327615954,
11.1186590444948));
#28300=CARTESIAN_POINT('Ctrl Pts',(-4.61357514386104,-19.7975966837424,
11.0943808405147));
#28301=CARTESIAN_POINT('Ctrl Pts',(-4.61949338394989,-19.8117563038103,
11.0914035456343));
#28302=CARTESIAN_POINT('Ctrl Pts',(-4.62534375904922,-19.8259396168614,
11.088453350286));
#28303=CARTESIAN_POINT('Ctrl Pts',(-4.631125403848,-19.8401452323389,11.0855311429861));
#28304=CARTESIAN_POINT('Ctrl Pts',(-4.70435613436058,-20.0200745837608,
11.0485182543125));
#28305=CARTESIAN_POINT('Ctrl Pts',(-4.76726266141392,-20.2043492164639,
11.0156989175618));
#28306=CARTESIAN_POINT('Ctrl Pts',(-4.81941146141461,-20.3931233167233,
10.9880108622482));
#28307=CARTESIAN_POINT('Ctrl Pts',(-4.85028537022025,-20.5048841694408,
10.9716185676078));
#28308=CARTESIAN_POINT('Ctrl Pts',(-4.87738947269955,-20.6182217880058,
10.9570246661856));
#28309=CARTESIAN_POINT('Ctrl Pts',(-4.90064154479525,-20.7331649364595,
10.944421333994));
#28310=CARTESIAN_POINT('Ctrl Pts',(-4.90391515449991,-20.7493475375075,
10.9426469376992));
#28311=CARTESIAN_POINT('Ctrl Pts',(-4.90711191771618,-20.7655594581114,
10.9409122343397));
#28312=CARTESIAN_POINT('Ctrl Pts',(-4.91023176158242,-20.7818011622264,
10.9392176722592));
#28313=CARTESIAN_POINT('Ctrl Pts',(-4.93378311546319,-20.9044079777082,
10.9264256118414));
#28314=CARTESIAN_POINT('Ctrl Pts',(-4.95272914746289,-21.0287068137377,
10.9160511524931));
#28315=CARTESIAN_POINT('Ctrl Pts',(-4.96704580471618,-21.1536260169313,
10.9081724913842));
#28316=CARTESIAN_POINT('Ctrl Pts',(-4.98091661294089,-21.2746549890179,
10.9005391873681));
#28317=CARTESIAN_POINT('Ctrl Pts',(-4.99044175459251,-21.396268070175,10.8952486342404));
#28318=CARTESIAN_POINT('Ctrl Pts',(-4.99555846674246,-21.5174896076691,
10.8923943107704));
#28319=CARTESIAN_POINT('Ctrl Pts',(-4.99848614792585,-21.586850166548,10.8907611235069));
#28320=CARTESIAN_POINT('Ctrl Pts',(-4.99996980849573,-21.6560823781017,
10.8899259483772));
#28321=CARTESIAN_POINT('Ctrl Pts',(-4.9999916022669,-21.7250000027207,10.88990980363));
#28322=CARTESIAN_POINT('Ctrl Pts',(0.187614356002326,-16.7285211545107,
-12.1982543436608));
#28323=CARTESIAN_POINT('Ctrl Pts',(0.5158722932195,-16.7408470150613,-12.1921453596449));
#28324=CARTESIAN_POINT('Ctrl Pts',(0.83589624549473,-16.7849264922226,-12.1702069739155));
#28325=CARTESIAN_POINT('Ctrl Pts',(1.30454329276147,-16.8955146240847,-12.1165436423938));
#28326=CARTESIAN_POINT('Ctrl Pts',(1.45884748782628,-16.9398479007978,-12.0951867686849));
#28327=CARTESIAN_POINT('Ctrl Pts',(1.76364451604006,-17.0436033466199,-12.0459567376793));
#28328=CARTESIAN_POINT('Ctrl Pts',(1.91480729566499,-17.1034045601589,-12.0179123563443));
#28329=CARTESIAN_POINT('Ctrl Pts',(2.35241421703558,-17.3013507250399,-11.9268899925891));
#28330=CARTESIAN_POINT('Ctrl Pts',(2.62606025966841,-17.4585239024972,-11.8567015361229));
#28331=CARTESIAN_POINT('Ctrl Pts',(3.14021868341892,-17.8214071167348,-11.7044430212222));
#28332=CARTESIAN_POINT('Ctrl Pts',(3.38265418689342,-18.0295254408124,-11.6214946028354));
#28333=CARTESIAN_POINT('Ctrl Pts',(3.81899306541419,-18.4824433648695,-11.4567396232169));
#28334=CARTESIAN_POINT('Ctrl Pts',(4.01441011445594,-18.727563041203,-11.3746407517478));
#28335=CARTESIAN_POINT('Ctrl Pts',(4.36024299024928,-19.2575320761983,-11.2195371333797));
#28336=CARTESIAN_POINT('Ctrl Pts',(4.50951743476146,-19.5419625548479,-11.1469697786176));
#28337=CARTESIAN_POINT('Ctrl Pts',(4.68989568786932,-19.9842448672363,-11.0558220109167));
#28338=CARTESIAN_POINT('Ctrl Pts',(4.74315776047347,-20.134924483598,-11.0281977430586));
#28339=CARTESIAN_POINT('Ctrl Pts',(4.83557077179125,-20.4431493848349,-10.9795288829077));
#28340=CARTESIAN_POINT('Ctrl Pts',(4.87488907212697,-20.6016955942573,-10.9583929606265));
#28341=CARTESIAN_POINT('Ctrl Pts',(4.96879046717059,-21.0795960122762,-10.9074448087627));
#28342=CARTESIAN_POINT('Ctrl Pts',(4.99999999999992,-21.4009211496768,-10.8899035808404));
#28343=CARTESIAN_POINT('Ctrl Pts',(5.,-21.7249999999987,-10.8899035808404));
#28344=CARTESIAN_POINT('Origin',(0.,-244.63,0.));
#28345=CARTESIAN_POINT('',(9.10831056865844E-16,-237.1925,-7.4375));
#28346=CARTESIAN_POINT('',(-9.10831056865844E-16,-237.1925,7.4375));
#28347=CARTESIAN_POINT('Origin',(0.,-237.1925,0.));
#28348=CARTESIAN_POINT('Origin',(0.,-237.1925,0.));
#28349=CARTESIAN_POINT('',(-9.10831056865844E-16,-212.63,7.4375));
#28350=CARTESIAN_POINT('',(-9.10831056865844E-16,-244.63,7.4375));
#28351=CARTESIAN_POINT('Origin',(0.,-212.63,0.));
#28352=CARTESIAN_POINT('Origin',(0.,-237.1925,0.));
#28353=CARTESIAN_POINT('',(0.,-244.63,0.));
#28354=CARTESIAN_POINT('',(-9.10831056865844E-16,-237.1925,-7.4375));
#28355=CARTESIAN_POINT('Origin',(0.,-44.45,0.));
#28356=CARTESIAN_POINT('',(1.55530143491714E-15,-43.45,12.7));
#28357=CARTESIAN_POINT('',(-1.55530143491714E-15,-43.45,-12.7));
#28358=CARTESIAN_POINT('Origin',(0.,-43.45,0.));
#28359=CARTESIAN_POINT('Origin',(0.,-43.45,0.));
#28360=CARTESIAN_POINT('',(-1.4328367550024E-15,-44.45,-11.7));
#28361=CARTESIAN_POINT('',(-1.43283675500241E-15,-44.45,-11.7));
#28362=CARTESIAN_POINT('Origin',(0.,-44.45,0.));
#28363=CARTESIAN_POINT('Origin',(0.,-244.63,0.));
#28364=CARTESIAN_POINT('',(-9.42978035343463E-16,-47.63,7.70000000000001));
#28365=CARTESIAN_POINT('Origin',(0.,-47.63,0.));
#28366=CARTESIAN_POINT('',(-9.42978035343463E-16,-44.45,7.70000000000001));
#28367=CARTESIAN_POINT('',(-9.42978035343463E-16,-244.63,7.70000000000001));
#28368=CARTESIAN_POINT('Origin',(0.,-44.45,0.));
#28369=CARTESIAN_POINT('Origin',(0.,-244.63,0.));
#28370=CARTESIAN_POINT('',(-1.55530143491714E-15,-244.63,12.7));
#28371=CARTESIAN_POINT('',(-1.71325927436869E-11,-16.2250000000013,12.7000002117864));
#28372=CARTESIAN_POINT('Ctrl Pts',(-5.7251211610453,-21.780229807,11.3363568967879));
#28373=CARTESIAN_POINT('Ctrl Pts',(-5.72592155092587,-21.7036657452032,
11.3359526814757));
#28374=CARTESIAN_POINT('Ctrl Pts',(-5.7250008654272,-21.6269621693104,11.3364279110386));
#28375=CARTESIAN_POINT('Ctrl Pts',(-5.72240032932084,-21.550122887081,11.3377497611332));
#28376=CARTESIAN_POINT('Ctrl Pts',(-5.71973912251023,-21.4714909385792,
11.3391024500906));
#28377=CARTESIAN_POINT('Ctrl Pts',(-5.71531887266977,-21.3927158329317,
11.3413417249685));
#28378=CARTESIAN_POINT('Ctrl Pts',(-5.70913701129969,-21.3137889985803,
11.3444562327139));
#28379=CARTESIAN_POINT('Ctrl Pts',(-5.70665440520126,-21.2820923576238,
11.3457070041984));
#28380=CARTESIAN_POINT('Ctrl Pts',(-5.70388716149817,-21.250371194257,11.3470991961792));
#28381=CARTESIAN_POINT('Ctrl Pts',(-5.70083299908356,-21.2186249953703,
11.3486331200433));
#28382=CARTESIAN_POINT('Ctrl Pts',(-5.69081304792642,-21.1144735721361,
11.3536655446856));
#28383=CARTESIAN_POINT('Ctrl Pts',(-5.67772497916359,-21.0103130463191,
11.3602133443104));
#28384=CARTESIAN_POINT('Ctrl Pts',(-5.6616113424946,-20.906924066588,11.3682258570849));
#28385=CARTESIAN_POINT('Ctrl Pts',(-5.65013554789805,-20.8332926003141,
11.3739322008911));
#28386=CARTESIAN_POINT('Ctrl Pts',(-5.63712616237809,-20.7600526651473,
11.3803809524082));
#28387=CARTESIAN_POINT('Ctrl Pts',(-5.62261270070195,-20.6874823252654,
11.3875469885781));
#28388=CARTESIAN_POINT('Ctrl Pts',(-5.62071109870733,-20.6779739180949,
11.3884859064585));
#28389=CARTESIAN_POINT('Ctrl Pts',(-5.61878497703484,-20.6684770185026,
11.389436447028));
#28390=CARTESIAN_POINT('Ctrl Pts',(-5.61683442793834,-20.6589917496983,
11.3903985013602));
#28391=CARTESIAN_POINT('Ctrl Pts',(-5.57286731662002,-20.4451853553105,
11.4120840615902));
#28392=CARTESIAN_POINT('Ctrl Pts',(-5.51634888901757,-20.2366355634731,
11.4396871913827));
#28393=CARTESIAN_POINT('Ctrl Pts',(-5.44783320687091,-20.0331524601257,
11.4722129615946));
#28394=CARTESIAN_POINT('Ctrl Pts',(-5.40433526811686,-19.9039689609678,
11.4928623066246));
#28395=CARTESIAN_POINT('Ctrl Pts',(-5.35600285931867,-19.7768269845679,
11.5154955399265));
#28396=CARTESIAN_POINT('Ctrl Pts',(-5.30298711896009,-19.651672639573,11.5398582133199));
#28397=CARTESIAN_POINT('Ctrl Pts',(-5.29614565259561,-19.6355219787341,
11.5430021175536));
#28398=CARTESIAN_POINT('Ctrl Pts',(-5.28922082277232,-19.6193988034393,
11.5461768842716));
#28399=CARTESIAN_POINT('Ctrl Pts',(-5.28221377395364,-19.603304781917,11.5493814791098));
#28400=CARTESIAN_POINT('Ctrl Pts',(-5.21348500003055,-19.4454462603995,
11.5808138095882));
#28401=CARTESIAN_POINT('Ctrl Pts',(-5.13672427863156,-19.2901792507329,
11.6151706224263));
#28402=CARTESIAN_POINT('Ctrl Pts',(-5.05299140769763,-19.1391643487573,
11.6514834037853));
#28403=CARTESIAN_POINT('Ctrl Pts',(-4.97563621249873,-18.9996517882781,
11.6850303520615));
#28404=CARTESIAN_POINT('Ctrl Pts',(-4.89233170424652,-18.8637690311732,
11.7202458572368));
#28405=CARTESIAN_POINT('Ctrl Pts',(-4.80393880809263,-18.7327852615055,
11.7563670702825));
#28406=CARTESIAN_POINT('Ctrl Pts',(-4.79665111102847,-18.7219860901332,
11.7593451428395));
#28407=CARTESIAN_POINT('Ctrl Pts',(-4.78932883567085,-18.7112201915641,
11.7623293760803));
#28408=CARTESIAN_POINT('Ctrl Pts',(-4.78197246933197,-18.7004882614148,
11.7653193451523));
#28409=CARTESIAN_POINT('Ctrl Pts',(-4.76879514041666,-18.6812643447474,
11.7706752238692));
#28410=CARTESIAN_POINT('Ctrl Pts',(-4.75550582199898,-18.6621369757864,
11.7760511749375));
#28411=CARTESIAN_POINT('Ctrl Pts',(-4.74210471042919,-18.6431061081163,
11.7814457754623));
#28412=CARTESIAN_POINT('Ctrl Pts',(-4.60834180066191,-18.4531499077152,
11.8352918657269));
#28413=CARTESIAN_POINT('Ctrl Pts',(-4.46337134494643,-18.2726619633985,
11.8910215785681));
#28414=CARTESIAN_POINT('Ctrl Pts',(-4.3070685843823,-18.1012807046439,11.9473601508487));
#28415=CARTESIAN_POINT('Ctrl Pts',(-4.23602178678706,-18.0233800357215,
11.9729686246029));
#28416=CARTESIAN_POINT('Ctrl Pts',(-4.16263331204804,-17.9473613616324,
11.9987034169121));
#28417=CARTESIAN_POINT('Ctrl Pts',(-4.08689000518079,-17.8731928595689,
12.0244471838457));
#28418=CARTESIAN_POINT('Ctrl Pts',(-4.06785307389009,-17.8545517315786,
12.0309174891776));
#28419=CARTESIAN_POINT('Ctrl Pts',(-4.04866165056352,-17.8360279422144,
12.0373891632641));
#28420=CARTESIAN_POINT('Ctrl Pts',(-4.02932492572199,-17.817629051679,12.043857485744));
#28421=CARTESIAN_POINT('Ctrl Pts',(-3.91639267653785,-17.7101740349846,
12.0816344211914));
#28422=CARTESIAN_POINT('Ctrl Pts',(-3.79852390663081,-17.6070014770466,
12.1192899300043));
#28423=CARTESIAN_POINT('Ctrl Pts',(-3.67755706750205,-17.5096130464424,
12.1558863936335));
#28424=CARTESIAN_POINT('Ctrl Pts',(-3.53535623962652,-17.3951294775805,
12.1989068400869));
#28425=CARTESIAN_POINT('Ctrl Pts',(-3.38821406470576,-17.2879449005781,
12.2406999056768));
#28426=CARTESIAN_POINT('Ctrl Pts',(-3.23615133134969,-17.1878625428924,
12.2807705197441));
#28427=CARTESIAN_POINT('Ctrl Pts',(-3.21342145855415,-17.1729025378401,
12.28676015271));
#28428=CARTESIAN_POINT('Ctrl Pts',(-3.19057632043218,-17.1580972322623,
12.2927127051079));
#28429=CARTESIAN_POINT('Ctrl Pts',(-3.16761661322188,-17.1434477682921,
12.2986262265451));
#28430=CARTESIAN_POINT('Ctrl Pts',(-2.97069010100861,-17.0177986117496,
12.3493467841231));
#28431=CARTESIAN_POINT('Ctrl Pts',(-2.7651980604181,-16.9035088337294,12.3972286024479));
#28432=CARTESIAN_POINT('Ctrl Pts',(-2.55156492209342,-16.8013656927296,
12.4410424599757));
#28433=CARTESIAN_POINT('Ctrl Pts',(-2.45522310210993,-16.7553023517146,
12.4608011304135));
#28434=CARTESIAN_POINT('Ctrl Pts',(-2.35722584962307,-16.7117088138121,
12.4797328794738));
#28435=CARTESIAN_POINT('Ctrl Pts',(-2.25761329062413,-16.6706547188598,
12.4977270822136));
#28436=CARTESIAN_POINT('Ctrl Pts',(-2.23350870399902,-16.6607203090019,
12.5020813807383));
#28437=CARTESIAN_POINT('Ctrl Pts',(-2.20935990045449,-16.6509543847314,
12.5063717966401));
#28438=CARTESIAN_POINT('Ctrl Pts',(-2.18516698386428,-16.6413565854661,
12.5105976886306));
#28439=CARTESIAN_POINT('Ctrl Pts',(-1.8843086225196,-16.5220002379706,12.5631500518289));
#28440=CARTESIAN_POINT('Ctrl Pts',(-1.57625905934626,-16.4284075359873,
12.6057869924533));
#28441=CARTESIAN_POINT('Ctrl Pts',(-1.26100785637197,-16.3600575419048,
12.6372413556761));
#28442=CARTESIAN_POINT('Ctrl Pts',(-1.23565759797098,-16.3545613217624,
12.6397706917357));
#28443=CARTESIAN_POINT('Ctrl Pts',(-1.21026079827882,-16.3492283346357,
12.6422277248466));
#28444=CARTESIAN_POINT('Ctrl Pts',(-1.18481746577651,-16.3440583132815,
12.6446117999945));
#28445=CARTESIAN_POINT('Ctrl Pts',(-1.16292712550636,-16.3396102510382,
12.6466629548978));
#28446=CARTESIAN_POINT('Ctrl Pts',(-1.14100210430354,-16.3352837242408,
12.6486600728867));
#28447=CARTESIAN_POINT('Ctrl Pts',(-1.11904222815108,-16.3310792360298,
12.6506026687393));
#28448=CARTESIAN_POINT('Ctrl Pts',(-0.956285503636157,-16.2999174605833,
12.6650003154217));
#28449=CARTESIAN_POINT('Ctrl Pts',(-0.791601235446541,-16.2754586182219,
12.6764033427023));
#28450=CARTESIAN_POINT('Ctrl Pts',(-0.624967432599858,-16.2578763159761,
12.6846133447174));
#28451=CARTESIAN_POINT('Ctrl Pts',(-0.604806175958912,-16.2557490086599,
12.6856066843329));
#28452=CARTESIAN_POINT('Ctrl Pts',(-0.584611468485983,-16.2537238228531,
12.686552593652));
#28453=CARTESIAN_POINT('Ctrl Pts',(-0.564389928132223,-16.2518009854779,
12.6874508724902));
#28454=CARTESIAN_POINT('Ctrl Pts',(-0.394675486070499,-16.2356630817079,
12.6949899070625));
#28455=CARTESIAN_POINT('Ctrl Pts',(-0.222970110451938,-16.2267466956113,
12.6991803470038));
#28456=CARTESIAN_POINT('Ctrl Pts',(-0.052979955040351,-16.2252370584114,
12.6998894926019));
#28457=CARTESIAN_POINT('Ctrl Pts',(-0.0353121499055092,-16.2250801553495,
12.6999631971421));
#28458=CARTESIAN_POINT('Ctrl Pts',(-0.0176522202715522,-16.2250011418722,
12.7000000775714));
#28459=CARTESIAN_POINT('Ctrl Pts',(-1.713259621314E-11,-16.2250000000013,
12.7000002117864));
#28460=CARTESIAN_POINT('',(-1.55530143491714E-15,-15.875,12.7));
#28461=CARTESIAN_POINT('',(-1.55530143491714E-15,-244.63,12.7));
#28462=CARTESIAN_POINT('Origin',(0.,-15.875,0.));
#28463=CARTESIAN_POINT('Ctrl Pts',(-1.713259621314E-11,-16.2250000000013,
12.7000002117864));
#28464=CARTESIAN_POINT('Ctrl Pts',(0.221363672027344,-16.2250000000212,
12.7000018947916));
#28465=CARTESIAN_POINT('Ctrl Pts',(0.441513190754386,-16.2372332268251,
12.6942230208429));
#28466=CARTESIAN_POINT('Ctrl Pts',(0.660354951916768,-16.2616652077622,
12.6828260961163));
#28467=CARTESIAN_POINT('Ctrl Pts',(0.799573752842758,-16.2772079043309,
12.6755758062894));
#28468=CARTESIAN_POINT('Ctrl Pts',(0.938263335008136,-16.2976865147767,
12.6660523329633));
#28469=CARTESIAN_POINT('Ctrl Pts',(1.07639994840503,-16.3230822291724,12.6543021597253));
#28470=CARTESIAN_POINT('Ctrl Pts',(1.08491495480765,-16.3246476698283,12.6535778564585));
#28471=CARTESIAN_POINT('Ctrl Pts',(1.09342994759773,-16.3262326511218,12.6528447542495));
#28472=CARTESIAN_POINT('Ctrl Pts',(1.10194446509101,-16.3278370612125,12.6521029273764));
#28473=CARTESIAN_POINT('Ctrl Pts',(1.27949553558937,-16.3612934172959,12.6366338000235));
#28474=CARTESIAN_POINT('Ctrl Pts',(1.45703513698099,-16.4032419539272,12.6173536765979));
#28475=CARTESIAN_POINT('Ctrl Pts',(1.63041748363299,-16.4527210984502,12.5949092425891));
#28476=CARTESIAN_POINT('Ctrl Pts',(1.6346503273299,-16.4539290500616,12.5943612987941));
#28477=CARTESIAN_POINT('Ctrl Pts',(1.63888098675367,-16.4551414837025,12.593811470957));
#28478=CARTESIAN_POINT('Ctrl Pts',(1.64310946414815,-16.4563583966121,12.5932597642597));
#28479=CARTESIAN_POINT('Ctrl Pts',(1.81996315945393,-16.507255096502,12.5701849410938));
#28480=CARTESIAN_POINT('Ctrl Pts',(1.99304998846898,-16.5660000215187,12.5438162804331));
#28481=CARTESIAN_POINT('Ctrl Pts',(2.16251275385891,-16.63240593341,12.5145330951417));
#28482=CARTESIAN_POINT('Ctrl Pts',(2.1630668666123,-16.6326230687942,12.5144373443944));
#28483=CARTESIAN_POINT('Ctrl Pts',(2.16362094061177,-16.6328402860942,12.5143415624717));
#28484=CARTESIAN_POINT('Ctrl Pts',(2.16417497585848,-16.6330575853119,12.5142457493862));
#28485=CARTESIAN_POINT('Ctrl Pts',(2.33666764411718,-16.7007112627337,12.484415418421));
#28486=CARTESIAN_POINT('Ctrl Pts',(2.50538039674436,-16.7762931353467,12.4515685497952));
#28487=CARTESIAN_POINT('Ctrl Pts',(2.6703975412241,-16.8598778146148,12.4160773584821));
#28488=CARTESIAN_POINT('Ctrl Pts',(2.83063219705356,-16.9410400620732,12.381614764653));
#28489=CARTESIAN_POINT('Ctrl Pts',(2.98813248544786,-17.0302527035357,12.3444553838994));
#28490=CARTESIAN_POINT('Ctrl Pts',(3.14001471210688,-17.1259429702128,12.3057021386053));
#28491=CARTESIAN_POINT('Ctrl Pts',(3.14461081664355,-17.1288386511523,12.3045294275487));
#28492=CARTESIAN_POINT('Ctrl Pts',(3.14920178649894,-17.131740271378,12.3033552545028));
#28493=CARTESIAN_POINT('Ctrl Pts',(3.15378754001488,-17.1346477865787,12.3021796504457));
#28494=CARTESIAN_POINT('Ctrl Pts',(3.38076485787962,-17.2785587053891,12.2439917310906));
#28495=CARTESIAN_POINT('Ctrl Pts',(3.59505414777261,-17.4364785198026,12.1824013050721));
#28496=CARTESIAN_POINT('Ctrl Pts',(3.79709489785007,-17.6085262541715,12.1190881100363));
#28497=CARTESIAN_POINT('Ctrl Pts',(3.86478108590455,-17.666164405378,12.097877394753));
#28498=CARTESIAN_POINT('Ctrl Pts',(3.93109267813204,-17.7253882661821,12.0764737353512));
#28499=CARTESIAN_POINT('Ctrl Pts',(3.99604650387532,-17.7862025795357,12.0549415457737));
#28500=CARTESIAN_POINT('Ctrl Pts',(4.00258006511678,-17.7923197564087,12.0527756705899));
#28501=CARTESIAN_POINT('Ctrl Pts',(4.00909996613724,-17.7984531203158,12.0506084698285));
#28502=CARTESIAN_POINT('Ctrl Pts',(4.01560621589262,-17.8046026712755,12.0484400117636));
#28503=CARTESIAN_POINT('Ctrl Pts',(4.14721247732648,-17.9289937478159,12.0045771614675));
#28504=CARTESIAN_POINT('Ctrl Pts',(4.27353389575726,-18.0606680305253,11.9600313905221));
#28505=CARTESIAN_POINT('Ctrl Pts',(4.39314902114322,-18.198165116782,11.9159327227938));
#28506=CARTESIAN_POINT('Ctrl Pts',(4.50543725205698,-18.3272399684927,11.8745352710177));
#28507=CARTESIAN_POINT('Ctrl Pts',(4.61181501935763,-18.4614451487399,11.8335324557008));
#28508=CARTESIAN_POINT('Ctrl Pts',(4.71110159808237,-18.5995347793932,11.7938760921501));
#28509=CARTESIAN_POINT('Ctrl Pts',(4.71690460935499,-18.6076057160052,11.7915582932323));
#28510=CARTESIAN_POINT('Ctrl Pts',(4.72268368303533,-18.6156902524801,11.7892449830829));
#28511=CARTESIAN_POINT('Ctrl Pts',(4.7284385795538,-18.6237881449308,11.7869363530806));
#28512=CARTESIAN_POINT('Ctrl Pts',(4.8696838599945,-18.8225387369724,11.7302745015473));
#28513=CARTESIAN_POINT('Ctrl Pts',(4.99754710031512,-19.0301338086101,11.6760653892489));
#28514=CARTESIAN_POINT('Ctrl Pts',(5.11150237280828,-19.2471420652657,11.6259546820761));
#28515=CARTESIAN_POINT('Ctrl Pts',(5.16114959164122,-19.3416866718558,11.6041228072496));
#28516=CARTESIAN_POINT('Ctrl Pts',(5.20815730681002,-19.4380178471292,11.583069405877));
#28517=CARTESIAN_POINT('Ctrl Pts',(5.2524838589806,-19.5361817726934,11.5629328655827));
#28518=CARTESIAN_POINT('Ctrl Pts',(5.25597752321097,-19.5439187109091,11.5613457737132));
#28519=CARTESIAN_POINT('Ctrl Pts',(5.25945467845056,-19.5516673853462,11.5597643117532));
#28520=CARTESIAN_POINT('Ctrl Pts',(5.2629152811409,-19.5594277771001,11.5581885580222));
#28521=CARTESIAN_POINT('Ctrl Pts',(5.31419025317372,-19.6744117569871,11.5348409692573));
#28522=CARTESIAN_POINT('Ctrl Pts',(5.36191135925266,-19.7924554425857,11.5126967199581));
#28523=CARTESIAN_POINT('Ctrl Pts',(5.40532924820431,-19.9118553979064,11.4922758454265));
#28524=CARTESIAN_POINT('Ctrl Pts',(5.42197752137286,-19.9576384408062,11.4844456098773));
#28525=CARTESIAN_POINT('Ctrl Pts',(5.43799345603299,-20.0036204551374,11.4768686567325));
#28526=CARTESIAN_POINT('Ctrl Pts',(5.45333635060538,-20.0497042730614,11.4695737653081));
#28527=CARTESIAN_POINT('Ctrl Pts',(5.45548050920907,-20.0561444538387,11.4685543094201));
#28528=CARTESIAN_POINT('Ctrl Pts',(5.45761164744171,-20.0625869137453,11.4675403033073));
#28529=CARTESIAN_POINT('Ctrl Pts',(5.45972965702712,-20.0690314064627,11.4665318240264));
#28530=CARTESIAN_POINT('Ctrl Pts',(5.5149605904824,-20.2370832183523,11.4402339014689));
#28531=CARTESIAN_POINT('Ctrl Pts',(5.56163184513152,-20.4071281981078,11.4175334462604));
#28532=CARTESIAN_POINT('Ctrl Pts',(5.59976054259138,-20.5790716204159,11.3988017977733));
#28533=CARTESIAN_POINT('Ctrl Pts',(5.60078189485067,-20.5836774636401,11.398300033675));
#28534=CARTESIAN_POINT('Ctrl Pts',(5.60179713081954,-20.588284691568,11.3978011111594));
#28535=CARTESIAN_POINT('Ctrl Pts',(5.6028062520001,-20.5928933047512,11.3973050368294));
#28536=CARTESIAN_POINT('Ctrl Pts',(5.66132456308721,-20.8601439235408,11.3685379942569));
#28537=CARTESIAN_POINT('Ctrl Pts',(5.69945338485962,-21.1320367632465,11.3493502464404));
#28538=CARTESIAN_POINT('Ctrl Pts',(5.71598745130091,-21.4089064857561,11.3409866054978));
#28539=CARTESIAN_POINT('Ctrl Pts',(5.72127276086345,-21.4974111616721,11.3383130689174));
#28540=CARTESIAN_POINT('Ctrl Pts',(5.72435111690867,-21.5864244670614,11.3367457922127));
#28541=CARTESIAN_POINT('Ctrl Pts',(5.72518221930917,-21.6759575456936,11.3363260607529));
#28542=CARTESIAN_POINT('',(-3.98168013490685E-8,-27.2249172597151,-12.6999510078656));
#28543=CARTESIAN_POINT('Origin',(-0.00396284819304756,-22.4165755189871,
-10.43604364865));
#28544=CARTESIAN_POINT('Ctrl Pts',(-1.7019301551402E-8,-27.2249172597024,
-12.6999510078581));
#28545=CARTESIAN_POINT('Ctrl Pts',(0.0919620281499745,-27.2248657333756,
-12.6999204986825));
#28546=CARTESIAN_POINT('Ctrl Pts',(0.184353662992845,-27.2226823876497,
-12.6988891026387));
#28547=CARTESIAN_POINT('Ctrl Pts',(0.276862348897653,-27.2183634804325,
-12.6968621751401));
#28548=CARTESIAN_POINT('Ctrl Pts',(0.462124174604044,-27.2097142533001,
-12.6928029639936));
#28549=CARTESIAN_POINT('Ctrl Pts',(0.647839459875023,-27.1925034530069,
-12.6847525512908));
#28550=CARTESIAN_POINT('Ctrl Pts',(0.831475394891656,-27.1666637039099,
-12.6727423017414));
#28551=CARTESIAN_POINT('Ctrl Pts',(0.860494367798756,-27.1625803910283,
-12.6708443883169));
#28552=CARTESIAN_POINT('Ctrl Pts',(0.889461358294665,-27.1582815166792,
-12.6688475550619));
#28553=CARTESIAN_POINT('Ctrl Pts',(0.918366295604896,-27.1537667230844,
-12.6667518858992));
#28554=CARTESIAN_POINT('Ctrl Pts',(0.98055647506929,-27.144052956163,-12.662242966197));
#28555=CARTESIAN_POINT('Ctrl Pts',(1.04239650412929,-27.1333908258806,-12.6573008409862));
#28556=CARTESIAN_POINT('Ctrl Pts',(1.10389408971677,-27.1217856443861,-12.6519371017105));
#28557=CARTESIAN_POINT('Ctrl Pts',(1.2625620332833,-27.0918434886922,-12.6380982904371));
#28558=CARTESIAN_POINT('Ctrl Pts',(1.41904274673861,-27.0556254034858,-12.6214427615578));
#28559=CARTESIAN_POINT('Ctrl Pts',(1.57325978677928,-27.0132680486838,-12.6021877405304));
#28560=CARTESIAN_POINT('Ctrl Pts',(1.72057085549696,-26.9728074925592,-12.5837949758593));
#28561=CARTESIAN_POINT('Ctrl Pts',(1.86581664047618,-26.9267456378757,-12.5630306730307));
#28562=CARTESIAN_POINT('Ctrl Pts',(2.00894530566494,-26.8752398114438,-12.5401012219179));
#28563=CARTESIAN_POINT('Ctrl Pts',(2.05715126527635,-26.8578925680705,-12.5323785467096));
#28564=CARTESIAN_POINT('Ctrl Pts',(2.10517405230903,-26.8398844404735,-12.524392320235));
#28565=CARTESIAN_POINT('Ctrl Pts',(2.15296898450167,-26.8212387765873,-12.5161611890146));
#28566=CARTESIAN_POINT('Ctrl Pts',(2.29352047974884,-26.7664071068085,-12.491955739869));
#28567=CARTESIAN_POINT('Ctrl Pts',(2.43251125386155,-26.7058815234932,-12.4655601671862));
#28568=CARTESIAN_POINT('Ctrl Pts',(2.5687690002987,-26.6401870104483,-12.4374255022749));
#28569=CARTESIAN_POINT('Ctrl Pts',(2.71342992195853,-26.5704410396425,-12.4075557395416));
#28570=CARTESIAN_POINT('Ctrl Pts',(2.85500904214592,-26.4948690946154,-12.3757261024131));
#28571=CARTESIAN_POINT('Ctrl Pts',(2.992100362019,-26.4141509519538,-12.3425004113455));
#28572=CARTESIAN_POINT('Ctrl Pts',(3.00032253918009,-26.4093098076006,-12.3405076701675));
#28573=CARTESIAN_POINT('Ctrl Pts',(3.00852857598774,-26.4044501657706,-12.3385099130153));
#28574=CARTESIAN_POINT('Ctrl Pts',(3.01671817046085,-26.3995721783131,-12.3365072636135));
#28575=CARTESIAN_POINT('Ctrl Pts',(3.05290384570193,-26.3780188192859,-12.3276585689542));
#28576=CARTESIAN_POINT('Ctrl Pts',(3.0888021169251,-26.3561051263587,-12.318712157291));
#28577=CARTESIAN_POINT('Ctrl Pts',(3.12441174007421,-26.333831450486,-12.309674813074));
#28578=CARTESIAN_POINT('Ctrl Pts',(3.34125762189574,-26.198195224688,-12.2546416309523));
#28579=CARTESIAN_POINT('Ctrl Pts',(3.54772308859836,-26.0490733658479,-12.1961505100754));
#28580=CARTESIAN_POINT('Ctrl Pts',(3.74391756194467,-25.8861282255617,-12.1356158763297));
#28581=CARTESIAN_POINT('Ctrl Pts',(3.79599109572935,-25.8428796614048,-12.1195488982863));
#28582=CARTESIAN_POINT('Ctrl Pts',(3.84734106675829,-25.7986573538643,-12.1033382387448));
#28583=CARTESIAN_POINT('Ctrl Pts',(3.89796951692403,-25.7534551371196,-12.087010947047));
#28584=CARTESIAN_POINT('Ctrl Pts',(3.92454494649468,-25.7297279970707,-12.0784405723036));
#28585=CARTESIAN_POINT('Ctrl Pts',(3.9509298956712,-25.7057129097212,-12.069833672881));
#28586=CARTESIAN_POINT('Ctrl Pts',(3.97710293758018,-25.6814305242753,-12.061202131027));
#28587=CARTESIAN_POINT('Ctrl Pts',(4.08451935206046,-25.5817735264872,-12.0257775410761));
#28588=CARTESIAN_POINT('Ctrl Pts',(4.18841193528078,-25.4775729320852,-11.9899221486096));
#28589=CARTESIAN_POINT('Ctrl Pts',(4.28726008864082,-25.3702924740377,-11.954472005567));
#28590=CARTESIAN_POINT('Ctrl Pts',(4.40974977111969,-25.2373537311704,-11.9105432459744));
#28591=CARTESIAN_POINT('Ctrl Pts',(4.5251682098118,-25.0991480820203,-11.867030450089));
#28592=CARTESIAN_POINT('Ctrl Pts',(4.6335846329197,-24.9556438900871,-11.8245462258172));
#28593=CARTESIAN_POINT('Ctrl Pts',(4.65262203277703,-24.9304452476239,-11.8170862013864));
#28594=CARTESIAN_POINT('Ctrl Pts',(4.67144842031647,-24.9050788727734,-11.8096560552095));
#28595=CARTESIAN_POINT('Ctrl Pts',(4.69006145813723,-24.8795447530719,-11.8022598374611));
#28596=CARTESIAN_POINT('Ctrl Pts',(4.7723035961848,-24.7667216546804,-11.7695794782985));
#28597=CARTESIAN_POINT('Ctrl Pts',(4.85034730639964,-24.650651948875,-11.7375752393652));
#28598=CARTESIAN_POINT('Ctrl Pts',(4.92411608245589,-24.5311963270221,-11.7065464803374));
#28599=CARTESIAN_POINT('Ctrl Pts',(4.94459812070782,-24.4980292508281,-11.6979312875242));
#28600=CARTESIAN_POINT('Ctrl Pts',(4.96475039072747,-24.4646009375596,-11.6893913462764));
#28601=CARTESIAN_POINT('Ctrl Pts',(4.98457075206297,-24.4309079012617,-11.6809332077249));
#28602=CARTESIAN_POINT('Ctrl Pts',(5.03933188484637,-24.3378183352667,-11.6575644486756));
#28603=CARTESIAN_POINT('Ctrl Pts',(5.09161161619109,-24.2425967726689,-11.6347969726201));
#28604=CARTESIAN_POINT('Ctrl Pts',(5.14119233544617,-24.1453998846143,-11.612845006953));
#28605=CARTESIAN_POINT('Ctrl Pts',(5.16010085472048,-24.1083320635178,-11.604473221062));
#28606=CARTESIAN_POINT('Ctrl Pts',(5.17861722716774,-24.0709772880951,-11.596219974711));
#28607=CARTESIAN_POINT('Ctrl Pts',(5.19673091228954,-24.0333455211125,-11.5880968161816));
#28608=CARTESIAN_POINT('Ctrl Pts',(5.21022735894756,-24.0053062164479,-11.5820442777252));
#28609=CARTESIAN_POINT('Ctrl Pts',(5.22346537779254,-23.9771875661639,-11.576080555973));
#28610=CARTESIAN_POINT('Ctrl Pts',(5.23644298045248,-23.9489937764396,-11.5702090530435));
#28611=CARTESIAN_POINT('Ctrl Pts',(5.34709859392846,-23.7085949000134,-11.5201447402644));
#28612=CARTESIAN_POINT('Ctrl Pts',(5.43928172673109,-23.4620964725225,-11.4765736062942));
#28613=CARTESIAN_POINT('Ctrl Pts',(5.51299566525125,-23.2092865166259,-11.4410293714832));
#28614=CARTESIAN_POINT('Ctrl Pts',(5.53168082450053,-23.1452037341757,-11.4320195464601));
#28615=CARTESIAN_POINT('Ctrl Pts',(5.54917921254299,-23.0807155378359,-11.4235256980846));
#28616=CARTESIAN_POINT('Ctrl Pts',(5.56549076766331,-23.0158187456202,-11.4155732451165));
#28617=CARTESIAN_POINT('Ctrl Pts',(5.57329864162245,-22.98475451108,-11.4117666337921));
#28618=CARTESIAN_POINT('Ctrl Pts',(5.58083243181111,-22.9535960971172,-11.4080840716811));
#28619=CARTESIAN_POINT('Ctrl Pts',(5.5880897436265,-22.9223425326086,-11.4045284354039));
#28620=CARTESIAN_POINT('Ctrl Pts',(5.62167888031574,-22.7776911414314,-11.3880718250264));
#28621=CARTESIAN_POINT('Ctrl Pts',(5.64935105012608,-22.6309587679954,-11.3743312617738));
#28622=CARTESIAN_POINT('Ctrl Pts',(5.67088043129442,-22.4821735999493,-11.3635872473284));
#28623=CARTESIAN_POINT('Ctrl Pts',(5.67570457147357,-22.4488349497754,-11.361179810191));
#28624=CARTESIAN_POINT('Ctrl Pts',(5.68021785890798,-22.4153642376299,-11.3589241136083));
#28625=CARTESIAN_POINT('Ctrl Pts',(5.68441662585656,-22.3817978431521,-11.3568229803739));
#28626=CARTESIAN_POINT('Ctrl Pts',(5.69835045506675,-22.2704059955969,-11.3498502590979));
#28627=CARTESIAN_POINT('Ctrl Pts',(5.70882198550556,-22.1578045395964,-11.3445789402659));
#28628=CARTESIAN_POINT('Ctrl Pts',(5.71566537362297,-22.0454619815195,-11.3411284191284));
#28629=CARTESIAN_POINT('Ctrl Pts',(5.71792815975813,-22.0083155887615,-11.3399874943036));
#28630=CARTESIAN_POINT('Ctrl Pts',(5.71979464301309,-21.9711976311711,-11.3390454595814));
#28631=CARTESIAN_POINT('Ctrl Pts',(5.72125994327243,-21.9341613129817,-11.3383060753985));
#28632=CARTESIAN_POINT('Ctrl Pts',(5.72265809038181,-21.8988223298017,-11.3376005764051));
#28633=CARTESIAN_POINT('Ctrl Pts',(5.72370246038071,-21.8635184569659,-11.337075434071));
#28634=CARTESIAN_POINT('Ctrl Pts',(5.72439386792677,-21.8282553410221,-11.336729461383));
#28635=CARTESIAN_POINT('Ctrl Pts',(5.72763135267748,-21.6631373859456,-11.3351094598252));
#28636=CARTESIAN_POINT('Ctrl Pts',(5.72315277323322,-21.4986115543393,-11.3374063209502));
#28637=CARTESIAN_POINT('Ctrl Pts',(5.71101505935482,-21.3347960248396,-11.3435120227631));
#28638=CARTESIAN_POINT('Ctrl Pts',(5.69891170879394,-21.1714442766673,-11.3496004386051));
#28639=CARTESIAN_POINT('Ctrl Pts',(5.67919259864153,-21.0087987989881,-11.3594760501232));
#28640=CARTESIAN_POINT('Ctrl Pts',(5.65196058833497,-20.8469737346032,-11.3730093420465));
#28641=CARTESIAN_POINT('Ctrl Pts',(5.64564096375417,-20.8094196340002,-11.3761499594059));
#28642=CARTESIAN_POINT('Ctrl Pts',(5.63889928922109,-20.7718633753357,-11.379494165011));
#28643=CARTESIAN_POINT('Ctrl Pts',(5.63174531056276,-20.7343459984228,-11.3830339551735));
#28644=CARTESIAN_POINT('Ctrl Pts',(5.61323924531877,-20.6372952441373,-11.3921907601945));
#28645=CARTESIAN_POINT('Ctrl Pts',(5.59191445744438,-20.5402412872527,-11.4026858495865));
#28646=CARTESIAN_POINT('Ctrl Pts',(5.56795652307117,-20.4440800872431,-11.4143716869199));
#28647=CARTESIAN_POINT('Ctrl Pts',(5.55687489104712,-20.3996011677796,-11.4197769170705));
#28648=CARTESIAN_POINT('Ctrl Pts',(5.54523057951688,-20.3553132317987,-11.4254365819491));
#28649=CARTESIAN_POINT('Ctrl Pts',(5.53304526406038,-20.3113039893352,-11.4313345723834));
#28650=CARTESIAN_POINT('Ctrl Pts',(5.52253653690031,-20.2733500173415,-11.436421053114));
#28651=CARTESIAN_POINT('Ctrl Pts',(5.51163177819215,-20.2355988095398,-11.4416817157982));
#28652=CARTESIAN_POINT('Ctrl Pts',(5.50033952748779,-20.198060350804,-11.4471079837937));
#28653=CARTESIAN_POINT('Ctrl Pts',(5.46317549856261,-20.0745171880821,-11.4649664237118));
#28654=CARTESIAN_POINT('Ctrl Pts',(5.42172773120231,-19.9529931589739,-11.4846598695274));
#28655=CARTESIAN_POINT('Ctrl Pts',(5.37619491489848,-19.8335655490195,-11.5059345966497));
#28656=CARTESIAN_POINT('Ctrl Pts',(5.37127472611302,-19.8206604305824,-11.5082335028518));
#28657=CARTESIAN_POINT('Ctrl Pts',(5.36630688151358,-19.8077797714875,-11.510550858192));
#28658=CARTESIAN_POINT('Ctrl Pts',(5.36129166305822,-19.7949236552371,-11.5128863323853));
#28659=CARTESIAN_POINT('Ctrl Pts',(5.34691188376625,-19.7580622271897,-11.519582671486));
#28660=CARTESIAN_POINT('Ctrl Pts',(5.33212860288283,-19.7213755536174,-11.5264349197701));
#28661=CARTESIAN_POINT('Ctrl Pts',(5.31695054271167,-19.6848766190699,-11.533433113328));
#28662=CARTESIAN_POINT('Ctrl Pts',(5.27638526845153,-19.5873286272035,-11.5521366655475));
#28663=CARTESIAN_POINT('Ctrl Pts',(5.23300493090568,-19.4911313617358,-11.5718807649671));
#28664=CARTESIAN_POINT('Ctrl Pts',(5.18683768202814,-19.3962495630333,-11.5925387023274));
#28665=CARTESIAN_POINT('Ctrl Pts',(5.1539521155395,-19.3286639525485,-11.6072536352961));
#28666=CARTESIAN_POINT('Ctrl Pts',(5.11965146781014,-19.2617460640714,-11.6224327042036));
#28667=CARTESIAN_POINT('Ctrl Pts',(5.0839318381286,-19.1954891982059,-11.6380349922324));
#28668=CARTESIAN_POINT('Ctrl Pts',(5.04090598405321,-19.115679909374,-11.6568286296232));
#28669=CARTESIAN_POINT('Ctrl Pts',(4.99577829317954,-19.0367621135859,-11.6762543884676));
#28670=CARTESIAN_POINT('Ctrl Pts',(4.94872505777747,-18.9590662319327,-11.6961606247422));
#28671=CARTESIAN_POINT('Ctrl Pts',(4.92227129859887,-18.9153848968479,-11.7073520927902));
#28672=CARTESIAN_POINT('Ctrl Pts',(4.89520974043141,-18.8720893817075,-11.7186951745409));
#28673=CARTESIAN_POINT('Ctrl Pts',(4.8675778112301,-18.8292348509718,-11.7301613905388));
#28674=CARTESIAN_POINT('Ctrl Pts',(4.84627354591299,-18.7961939334816,-11.739001862951));
#28675=CARTESIAN_POINT('Ctrl Pts',(4.82466820516189,-18.7634613348383,-11.7478998973589));
#28676=CARTESIAN_POINT('Ctrl Pts',(4.80277580072744,-18.7310503313297,-11.7568440949918));
#28677=CARTESIAN_POINT('Ctrl Pts',(4.69567916281518,-18.5724971894157,-11.8005986993878));
#28678=CARTESIAN_POINT('Ctrl Pts',(4.58107418642852,-18.4206274814446,-11.8457174546917));
#28679=CARTESIAN_POINT('Ctrl Pts',(4.45915446310147,-18.2752432087695,-11.8914321663685));
#28680=CARTESIAN_POINT('Ctrl Pts',(4.37478828667904,-18.1746400014881,-11.9230658949006));
#28681=CARTESIAN_POINT('Ctrl Pts',(4.28692040782722,-18.0771416225569,-11.9549851094832));
#28682=CARTESIAN_POINT('Ctrl Pts',(4.1956265966026,-17.9826746468627,-11.9869394509486));
#28683=CARTESIAN_POINT('Ctrl Pts',(4.17052053334575,-17.95669595416,-11.9957269876655));
#28684=CARTESIAN_POINT('Ctrl Pts',(4.14512819596976,-17.9309341256672,-12.004523640522));
#28685=CARTESIAN_POINT('Ctrl Pts',(4.11946314917148,-17.9053995464596,-12.0133206849436));
#28686=CARTESIAN_POINT('Ctrl Pts',(3.99766032356665,-17.7842159023165,-12.0550702627233));
#28687=CARTESIAN_POINT('Ctrl Pts',(3.86946339986725,-17.6679311930972,-12.0969136064702));
#28688=CARTESIAN_POINT('Ctrl Pts',(3.73626746162298,-17.557697063915,-12.1379220118173));
#28689=CARTESIAN_POINT('Ctrl Pts',(3.61575222290182,-17.4579575931118,-12.1750262795984));
#28690=CARTESIAN_POINT('Ctrl Pts',(3.49114538313714,-17.3631715319409,-12.2114466943468));
#28691=CARTESIAN_POINT('Ctrl Pts',(3.36348515525031,-17.2741576657265,-12.2465083840004));
#28692=CARTESIAN_POINT('Ctrl Pts',(3.33817437369643,-17.2565091736291,-12.2534599520998));
#28693=CARTESIAN_POINT('Ctrl Pts',(3.31273120437577,-17.2390694750856,-12.2603640039171));
#28694=CARTESIAN_POINT('Ctrl Pts',(3.28715560804173,-17.2218389907719,-12.2672180913233));
#28695=CARTESIAN_POINT('Ctrl Pts',(3.13817522652918,-17.1214697132324,-12.3071438292555));
#28696=CARTESIAN_POINT('Ctrl Pts',(2.98455940472934,-17.028087697893,-12.345410271681));
#28697=CARTESIAN_POINT('Ctrl Pts',(2.82627288516427,-16.9417913892476,-12.3815390224694));
#28698=CARTESIAN_POINT('Ctrl Pts',(2.68919781167141,-16.8670593597467,-12.4128262804313));
#28699=CARTESIAN_POINT('Ctrl Pts',(2.5486203623837,-16.7976406813461,-12.4425104528035));
#28700=CARTESIAN_POINT('Ctrl Pts',(2.40453611326549,-16.7335765984635,-12.4702929425024));
#28701=CARTESIAN_POINT('Ctrl Pts',(2.38315623382809,-16.7240704770333,-12.4744154353069));
#28702=CARTESIAN_POINT('Ctrl Pts',(2.36168266030452,-16.7146790116667,-12.4784979351355));
#28703=CARTESIAN_POINT('Ctrl Pts',(2.3401251353203,-16.7054060581952,-12.4825380108379));
#28704=CARTESIAN_POINT('Ctrl Pts',(2.22756904715961,-16.6569901398923,-12.5036320426096));
#28705=CARTESIAN_POINT('Ctrl Pts',(2.11250061650078,-16.6117209023858,-12.5236098153468));
#28706=CARTESIAN_POINT('Ctrl Pts',(1.99642655688378,-16.5702166143712,-12.5420945500035));
#28707=CARTESIAN_POINT('Ctrl Pts',(1.95758723480752,-16.5563289428702,-12.5482796921893));
#28708=CARTESIAN_POINT('Ctrl Pts',(1.91863542297512,-16.5428624279043,-12.5542978218573));
#28709=CARTESIAN_POINT('Ctrl Pts',(1.87962761015771,-16.5298389828478,-12.5601353514636));
#28710=CARTESIAN_POINT('Ctrl Pts',(1.8619346620097,-16.5239318806175,-12.5627831058794));
#28711=CARTESIAN_POINT('Ctrl Pts',(1.84422418636504,-16.5181122065921,-12.5653952768144));
#28712=CARTESIAN_POINT('Ctrl Pts',(1.82649684649618,-16.5123799001449,-12.5679716062491));
#28713=CARTESIAN_POINT('Ctrl Pts',(1.66534273955609,-16.4602691642401,-12.5913922701672));
#28714=CARTESIAN_POINT('Ctrl Pts',(1.50261810408699,-16.4153143921165,-12.611876524808));
#28715=CARTESIAN_POINT('Ctrl Pts',(1.3383391466942,-16.3773802058618,-12.6292853450775));
#28716=CARTESIAN_POINT('Ctrl Pts',(1.32563644048517,-16.374446982819,-12.6306314647075));
#28717=CARTESIAN_POINT('Ctrl Pts',(1.31292448911361,-16.3715553979143,-12.6319592494833));
#28718=CARTESIAN_POINT('Ctrl Pts',(1.30020327362486,-16.3687055245917,-12.6332686220619));
#28719=CARTESIAN_POINT('Ctrl Pts',(1.01314339992633,-16.3043968681773,-12.6628151954506));
#28720=CARTESIAN_POINT('Ctrl Pts',(0.721379562021647,-16.2612760127206,
-12.68298231415));
#28721=CARTESIAN_POINT('Ctrl Pts',(0.42469199194604,-16.2401281321735,-12.6929008886698));
#28722=CARTESIAN_POINT('Ctrl Pts',(0.355011601791331,-16.2351613161822,
-12.695230376697));
#28723=CARTESIAN_POINT('Ctrl Pts',(0.285059746695848,-16.2314063896488,
-12.6969946851133));
#28724=CARTESIAN_POINT('Ctrl Pts',(0.214833815848646,-16.2288732699618,
-12.6981828003682));
#28725=CARTESIAN_POINT('Origin',(0.,-44.45,12.7));
#28726=CARTESIAN_POINT('Origin',(0.,-47.63,7.70000000000001));
#28727=CARTESIAN_POINT('',(2.55537495509676,-47.63,-8.00360031633711));
#28728=CARTESIAN_POINT('',(-7.96780251527898,-47.63,-2.66489817109789));
#28729=CARTESIAN_POINT('Ctrl Pts',(2.55537495509679,-47.63,-8.0036003163371));
#28730=CARTESIAN_POINT('Ctrl Pts',(1.86263429679466,-47.63,-8.16654376028585));
#28731=CARTESIAN_POINT('Ctrl Pts',(0.765908078329645,-47.63,-8.37785612188963));
#28732=CARTESIAN_POINT('Ctrl Pts',(-1.6692617677719,-47.63,-8.16209001543163));
#28733=CARTESIAN_POINT('Ctrl Pts',(-2.74375110300835,-47.63,-7.85437659041765));
#28734=CARTESIAN_POINT('Ctrl Pts',(-4.69944968573892,-47.63,-6.8614528643732));
#28735=CARTESIAN_POINT('Ctrl Pts',(-5.56511466324777,-47.63,-6.19428529183315));
#28736=CARTESIAN_POINT('Ctrl Pts',(-7.19394906010722,-47.63,-4.37070183094962));
#28737=CARTESIAN_POINT('Ctrl Pts',(-7.67609992676134,-47.63,-3.3577148847143));
#28738=CARTESIAN_POINT('Ctrl Pts',(-7.96780251527896,-47.63,-2.66489817109788));
#28739=CARTESIAN_POINT('',(4.50738083181344,-47.63,8.84193633985987));
#28740=CARTESIAN_POINT('Ctrl Pts',(-7.96780251527901,-47.63,-2.66489817109774));
#28741=CARTESIAN_POINT('Ctrl Pts',(-8.23599312974433,-47.63,-2.027924255025));
#28742=CARTESIAN_POINT('Ctrl Pts',(-8.42634396183627,-47.63,-1.36096366704783));
#28743=CARTESIAN_POINT('Ctrl Pts',(-8.64297828766043,-47.63,0.00360816572509623));
#28744=CARTESIAN_POINT('Ctrl Pts',(-8.66859900866028,-47.63,0.696135165601388));
#28745=CARTESIAN_POINT('Ctrl Pts',(-8.52525050570627,-47.63,2.41043360782728));
#28746=CARTESIAN_POINT('Ctrl Pts',(-8.25568996932099,-47.6300000000836,
3.41277917262432));
#28747=CARTESIAN_POINT('Ctrl Pts',(-7.37169226325108,-47.6300000000836,
5.28253364315782));
#28748=CARTESIAN_POINT('Ctrl Pts',(-6.69159903012225,-47.6300000000001,
6.31291964415818));
#28749=CARTESIAN_POINT('Ctrl Pts',(-4.74829296569675,-47.6300000000001,
8.0685409876383));
#28750=CARTESIAN_POINT('Ctrl Pts',(-3.68909457138915,-47.63,8.69991320242805));
#28751=CARTESIAN_POINT('Ctrl Pts',(-1.08588604418679,-47.63,9.62226726459695));
#28752=CARTESIAN_POINT('Ctrl Pts',(0.195202339559025,-47.63,9.67166205579392));
#28753=CARTESIAN_POINT('Ctrl Pts',(2.25253429025304,-47.63,9.57488020226805));
#28754=CARTESIAN_POINT('Ctrl Pts',(3.41720895858092,-47.63,9.30785410203652));
#28755=CARTESIAN_POINT('Ctrl Pts',(4.50738083181199,-47.63,8.84193633986041));
#28756=CARTESIAN_POINT('Ctrl Pts',(4.50738083181341,-47.63,8.84193633985991));
#28757=CARTESIAN_POINT('Ctrl Pts',(5.50129019941108,-47.63,8.24752673459283));
#28758=CARTESIAN_POINT('Ctrl Pts',(6.3827306396232,-47.63,7.48282682306558));
#28759=CARTESIAN_POINT('Ctrl Pts',(7.7290655812775,-47.63,5.82007728703929));
#28760=CARTESIAN_POINT('Ctrl Pts',(8.42964347032193,-47.6300000000064,4.72920057212086));
#28761=CARTESIAN_POINT('Ctrl Pts',(9.20437486461963,-47.6300000000064,2.13877895901777));
#28762=CARTESIAN_POINT('Ctrl Pts',(9.31838831238719,-47.63,0.915490022080004));
#28763=CARTESIAN_POINT('Ctrl Pts',(9.06300659638666,-47.63,-1.5079931069641));
#28764=CARTESIAN_POINT('Ctrl Pts',(8.69486484793724,-47.63,-2.68367031517789));
#28765=CARTESIAN_POINT('Ctrl Pts',(7.55278087878427,-47.63,-4.7656464219269));
#28766=CARTESIAN_POINT('Ctrl Pts',(6.81838193887884,-47.630000000013,-5.6526889049818));
#28767=CARTESIAN_POINT('Ctrl Pts',(5.41795245135679,-47.630000000013,-6.76839622139177));
#28768=CARTESIAN_POINT('Ctrl Pts',(4.87996243897364,-47.6300000023591,-7.10670058837738));
#28769=CARTESIAN_POINT('Ctrl Pts',(3.74918166874711,-47.6300000023591,-7.6527881999309));
#28770=CARTESIAN_POINT('Ctrl Pts',(3.16100732091453,-47.63,-7.86114610599088));
#28771=CARTESIAN_POINT('Ctrl Pts',(2.55537495509679,-47.63,-8.00360031633713));
#28772=CARTESIAN_POINT('Ctrl Pts',(-1.78726082715848E-11,-214.73675111262,
-9.92453123331945));
#28773=CARTESIAN_POINT('Ctrl Pts',(-5.7299307791557,-214.56175111262,-9.92453123330913));
#28774=CARTESIAN_POINT('Ctrl Pts',(-8.59489616871569,-214.38675111262,-4.96226561664425));
#28775=CARTESIAN_POINT('Ctrl Pts',(-11.4598615582757,-214.21175111262,2.06368086793017E-11));
#28776=CARTESIAN_POINT('Ctrl Pts',(-8.59489616869782,-214.03675111262,4.9622656166752));
#28777=CARTESIAN_POINT('Ctrl Pts',(-5.72993077911996,-213.86175111262,9.92453123332977));
#28778=CARTESIAN_POINT('Ctrl Pts',(1.7871392867044E-11,-213.68675111262,
9.92453123331945));
#28779=CARTESIAN_POINT('Ctrl Pts',(5.7299307791557,-213.51175111262,9.92453123330913));
#28780=CARTESIAN_POINT('Ctrl Pts',(8.59489616871569,-213.33675111262,4.96226561664425));
#28781=CARTESIAN_POINT('Ctrl Pts',(11.4598615582757,-213.16175111262,-2.06354052510241E-11));
#28782=CARTESIAN_POINT('Ctrl Pts',(8.59489616869782,-212.98675111262,-4.9622656166752));
#28783=CARTESIAN_POINT('Ctrl Pts',(5.72993077911996,-212.81175111262,-9.92453123332976));
#28784=CARTESIAN_POINT('Ctrl Pts',(-1.78726082715848E-11,-212.63675111262,
-9.92453123331945));
#28785=CARTESIAN_POINT('Ctrl Pts',(-5.7299307791557,-212.46175111262,-9.92453123330913));
#28786=CARTESIAN_POINT('Ctrl Pts',(-8.59489616871569,-212.28675111262,-4.96226561664425));
#28787=CARTESIAN_POINT('Ctrl Pts',(-11.4598615582757,-212.11175111262,2.06368086793017E-11));
#28788=CARTESIAN_POINT('Ctrl Pts',(-8.59489616869782,-211.93675111262,4.9622656166752));
#28789=CARTESIAN_POINT('Ctrl Pts',(-5.72993077911996,-211.76175111262,9.92453123332977));
#28790=CARTESIAN_POINT('Ctrl Pts',(1.7871392867044E-11,-211.58675111262,
9.92453123331945));
#28791=CARTESIAN_POINT('Ctrl Pts',(5.7299307791557,-211.41175111262,9.92453123330913));
#28792=CARTESIAN_POINT('Ctrl Pts',(8.59489616871569,-211.23675111262,4.96226561664425));
#28793=CARTESIAN_POINT('Ctrl Pts',(11.4598615582757,-211.06175111262,-2.06354052510241E-11));
#28794=CARTESIAN_POINT('Ctrl Pts',(8.59489616869782,-210.88675111262,-4.9622656166752));
#28795=CARTESIAN_POINT('Ctrl Pts',(5.72993077911996,-210.71175111262,-9.92453123332976));
#28796=CARTESIAN_POINT('Ctrl Pts',(-1.78726082715848E-11,-210.53675111262,
-9.92453123331945));
#28797=CARTESIAN_POINT('Ctrl Pts',(-5.7299307791557,-210.36175111262,-9.92453123330913));
#28798=CARTESIAN_POINT('Ctrl Pts',(-8.59489616871569,-210.18675111262,-4.96226561664425));
#28799=CARTESIAN_POINT('Ctrl Pts',(-11.4598615582757,-210.01175111262,2.06368086793017E-11));
#28800=CARTESIAN_POINT('Ctrl Pts',(-8.59489616869782,-209.83675111262,4.9622656166752));
#28801=CARTESIAN_POINT('Ctrl Pts',(-5.72993077911996,-209.66175111262,9.92453123332977));
#28802=CARTESIAN_POINT('Ctrl Pts',(1.7871392867044E-11,-209.48675111262,
9.92453123331945));
#28803=CARTESIAN_POINT('Ctrl Pts',(5.7299307791557,-209.31175111262,9.92453123330913));
#28804=CARTESIAN_POINT('Ctrl Pts',(8.59489616871569,-209.13675111262,4.96226561664425));
#28805=CARTESIAN_POINT('Ctrl Pts',(11.4598615582757,-208.96175111262,-2.06354052510241E-11));
#28806=CARTESIAN_POINT('Ctrl Pts',(8.59489616869782,-208.78675111262,-4.9622656166752));
#28807=CARTESIAN_POINT('Ctrl Pts',(5.72993077911996,-208.61175111262,-9.92453123332976));
#28808=CARTESIAN_POINT('Ctrl Pts',(-1.78726082715848E-11,-208.43675111262,
-9.92453123331945));
#28809=CARTESIAN_POINT('Ctrl Pts',(-5.7299307791557,-208.26175111262,-9.92453123330913));
#28810=CARTESIAN_POINT('Ctrl Pts',(-8.59489616871569,-208.08675111262,-4.96226561664425));
#28811=CARTESIAN_POINT('Ctrl Pts',(-11.4598615582757,-207.91175111262,2.06368086793017E-11));
#28812=CARTESIAN_POINT('Ctrl Pts',(-8.59489616869782,-207.73675111262,4.9622656166752));
#28813=CARTESIAN_POINT('Ctrl Pts',(-5.72993077911996,-207.56175111262,9.92453123332977));
#28814=CARTESIAN_POINT('Ctrl Pts',(1.7871392867044E-11,-207.38675111262,
9.92453123331945));
#28815=CARTESIAN_POINT('Ctrl Pts',(5.7299307791557,-207.21175111262,9.92453123330913));
#28816=CARTESIAN_POINT('Ctrl Pts',(8.59489616871569,-207.03675111262,4.96226561664425));
#28817=CARTESIAN_POINT('Ctrl Pts',(11.4598615582757,-206.86175111262,-2.06354052510241E-11));
#28818=CARTESIAN_POINT('Ctrl Pts',(8.59489616869782,-206.68675111262,-4.9622656166752));
#28819=CARTESIAN_POINT('Ctrl Pts',(5.72993077911996,-206.51175111262,-9.92453123332976));
#28820=CARTESIAN_POINT('Ctrl Pts',(-1.78726082715848E-11,-206.33675111262,
-9.92453123331945));
#28821=CARTESIAN_POINT('Ctrl Pts',(-5.7299307791557,-206.16175111262,-9.92453123330913));
#28822=CARTESIAN_POINT('Ctrl Pts',(-8.59489616871569,-205.98675111262,-4.96226561664425));
#28823=CARTESIAN_POINT('Ctrl Pts',(-11.4598615582757,-205.81175111262,2.06368086793017E-11));
#28824=CARTESIAN_POINT('Ctrl Pts',(-8.59489616869782,-205.63675111262,4.9622656166752));
#28825=CARTESIAN_POINT('Ctrl Pts',(-5.72993077911996,-205.46175111262,9.92453123332977));
#28826=CARTESIAN_POINT('Ctrl Pts',(1.7871392867044E-11,-205.28675111262,
9.92453123331945));
#28827=CARTESIAN_POINT('Ctrl Pts',(5.7299307791557,-205.11175111262,9.92453123330913));
#28828=CARTESIAN_POINT('Ctrl Pts',(8.59489616871569,-204.93675111262,4.96226561664425));
#28829=CARTESIAN_POINT('Ctrl Pts',(11.4598615582757,-204.76175111262,-2.06354052510241E-11));
#28830=CARTESIAN_POINT('Ctrl Pts',(8.59489616869782,-204.58675111262,-4.9622656166752));
#28831=CARTESIAN_POINT('Ctrl Pts',(5.72993077911996,-204.41175111262,-9.92453123332976));
#28832=CARTESIAN_POINT('Ctrl Pts',(-1.78726082715848E-11,-204.23675111262,
-9.92453123331945));
#28833=CARTESIAN_POINT('Ctrl Pts',(-5.7299307791557,-204.06175111262,-9.92453123330913));
#28834=CARTESIAN_POINT('Ctrl Pts',(-8.59489616871569,-203.88675111262,-4.96226561664425));
#28835=CARTESIAN_POINT('Ctrl Pts',(-11.4598615582757,-203.71175111262,2.06368086793017E-11));
#28836=CARTESIAN_POINT('Ctrl Pts',(-8.59489616869782,-203.53675111262,4.9622656166752));
#28837=CARTESIAN_POINT('Ctrl Pts',(-5.72993077911996,-203.36175111262,9.92453123332977));
#28838=CARTESIAN_POINT('Ctrl Pts',(1.7871392867044E-11,-203.18675111262,
9.92453123331945));
#28839=CARTESIAN_POINT('Ctrl Pts',(5.7299307791557,-203.01175111262,9.92453123330913));
#28840=CARTESIAN_POINT('Ctrl Pts',(8.59489616871569,-202.83675111262,4.96226561664425));
#28841=CARTESIAN_POINT('Ctrl Pts',(11.4598615582757,-202.66175111262,-2.06354052510241E-11));
#28842=CARTESIAN_POINT('Ctrl Pts',(8.59489616869782,-202.48675111262,-4.9622656166752));
#28843=CARTESIAN_POINT('Ctrl Pts',(5.72993077911996,-202.31175111262,-9.92453123332976));
#28844=CARTESIAN_POINT('Ctrl Pts',(-1.78726082715848E-11,-202.13675111262,
-9.92453123331945));
#28845=CARTESIAN_POINT('Ctrl Pts',(-5.7299307791557,-201.96175111262,-9.92453123330913));
#28846=CARTESIAN_POINT('Ctrl Pts',(-8.59489616871569,-201.78675111262,-4.96226561664425));
#28847=CARTESIAN_POINT('Ctrl Pts',(-11.4598615582757,-201.61175111262,2.06368086793017E-11));
#28848=CARTESIAN_POINT('Ctrl Pts',(-8.59489616869782,-201.43675111262,4.9622656166752));
#28849=CARTESIAN_POINT('Ctrl Pts',(-5.72993077911996,-201.26175111262,9.92453123332977));
#28850=CARTESIAN_POINT('Ctrl Pts',(1.7871392867044E-11,-201.08675111262,
9.92453123331945));
#28851=CARTESIAN_POINT('Ctrl Pts',(5.7299307791557,-200.91175111262,9.92453123330913));
#28852=CARTESIAN_POINT('Ctrl Pts',(8.59489616871569,-200.73675111262,4.96226561664425));
#28853=CARTESIAN_POINT('Ctrl Pts',(11.4598615582757,-200.56175111262,-2.06354052510241E-11));
#28854=CARTESIAN_POINT('Ctrl Pts',(8.59489616869782,-200.38675111262,-4.9622656166752));
#28855=CARTESIAN_POINT('Ctrl Pts',(5.72993077911996,-200.21175111262,-9.92453123332976));
#28856=CARTESIAN_POINT('Ctrl Pts',(-1.78726082715848E-11,-200.03675111262,
-9.92453123331945));
#28857=CARTESIAN_POINT('Ctrl Pts',(-5.7299307791557,-199.86175111262,-9.92453123330913));
#28858=CARTESIAN_POINT('Ctrl Pts',(-8.59489616871569,-199.68675111262,-4.96226561664425));
#28859=CARTESIAN_POINT('Ctrl Pts',(-11.4598615582757,-199.51175111262,2.06368086793017E-11));
#28860=CARTESIAN_POINT('Ctrl Pts',(-8.59489616869782,-199.33675111262,4.9622656166752));
#28861=CARTESIAN_POINT('Ctrl Pts',(-5.72993077911996,-199.16175111262,9.92453123332977));
#28862=CARTESIAN_POINT('Ctrl Pts',(1.7871392867044E-11,-198.98675111262,
9.92453123331945));
#28863=CARTESIAN_POINT('Ctrl Pts',(5.7299307791557,-198.81175111262,9.92453123330913));
#28864=CARTESIAN_POINT('Ctrl Pts',(8.59489616871569,-198.63675111262,4.96226561664425));
#28865=CARTESIAN_POINT('Ctrl Pts',(11.4598615582757,-198.46175111262,-2.06354052510241E-11));
#28866=CARTESIAN_POINT('Ctrl Pts',(8.59489616869782,-198.28675111262,-4.9622656166752));
#28867=CARTESIAN_POINT('Ctrl Pts',(5.72993077911996,-198.11175111262,-9.92453123332976));
#28868=CARTESIAN_POINT('Ctrl Pts',(-1.78726082715848E-11,-197.93675111262,
-9.92453123331945));
#28869=CARTESIAN_POINT('Ctrl Pts',(-5.7299307791557,-197.76175111262,-9.92453123330913));
#28870=CARTESIAN_POINT('Ctrl Pts',(-8.59489616871569,-197.58675111262,-4.96226561664425));
#28871=CARTESIAN_POINT('Ctrl Pts',(-11.4598615582757,-197.41175111262,2.06368086793017E-11));
#28872=CARTESIAN_POINT('Ctrl Pts',(-8.59489616869782,-197.23675111262,4.9622656166752));
#28873=CARTESIAN_POINT('Ctrl Pts',(-5.72993077911996,-197.06175111262,9.92453123332977));
#28874=CARTESIAN_POINT('Ctrl Pts',(1.7871392867044E-11,-196.88675111262,
9.92453123331945));
#28875=CARTESIAN_POINT('Ctrl Pts',(5.7299307791557,-196.71175111262,9.92453123330913));
#28876=CARTESIAN_POINT('Ctrl Pts',(8.59489616871569,-196.53675111262,4.96226561664425));
#28877=CARTESIAN_POINT('Ctrl Pts',(11.4598615582757,-196.36175111262,-2.06354052510241E-11));
#28878=CARTESIAN_POINT('Ctrl Pts',(8.59489616869782,-196.18675111262,-4.9622656166752));
#28879=CARTESIAN_POINT('Ctrl Pts',(5.72993077911996,-196.01175111262,-9.92453123332976));
#28880=CARTESIAN_POINT('Ctrl Pts',(-1.78726082715848E-11,-195.83675111262,
-9.92453123331945));
#28881=CARTESIAN_POINT('Ctrl Pts',(-5.7299307791557,-195.66175111262,-9.92453123330913));
#28882=CARTESIAN_POINT('Ctrl Pts',(-8.59489616871569,-195.48675111262,-4.96226561664425));
#28883=CARTESIAN_POINT('Ctrl Pts',(-11.4598615582757,-195.31175111262,2.06368086793017E-11));
#28884=CARTESIAN_POINT('Ctrl Pts',(-8.59489616869782,-195.13675111262,4.9622656166752));
#28885=CARTESIAN_POINT('Ctrl Pts',(-5.72993077911996,-194.96175111262,9.92453123332977));
#28886=CARTESIAN_POINT('Ctrl Pts',(1.7871392867044E-11,-194.78675111262,
9.92453123331945));
#28887=CARTESIAN_POINT('Ctrl Pts',(5.7299307791557,-194.61175111262,9.92453123330913));
#28888=CARTESIAN_POINT('Ctrl Pts',(8.59489616871569,-194.43675111262,4.96226561664425));
#28889=CARTESIAN_POINT('Ctrl Pts',(11.4598615582757,-194.26175111262,-2.06354052510241E-11));
#28890=CARTESIAN_POINT('Ctrl Pts',(8.59489616869782,-194.08675111262,-4.9622656166752));
#28891=CARTESIAN_POINT('Ctrl Pts',(5.72993077911996,-193.91175111262,-9.92453123332976));
#28892=CARTESIAN_POINT('Ctrl Pts',(-1.78726082715848E-11,-193.73675111262,
-9.92453123331945));
#28893=CARTESIAN_POINT('Ctrl Pts',(-5.7299307791557,-193.56175111262,-9.92453123330913));
#28894=CARTESIAN_POINT('Ctrl Pts',(-8.59489616871569,-193.38675111262,-4.96226561664425));
#28895=CARTESIAN_POINT('Ctrl Pts',(-11.4598615582757,-193.21175111262,2.06368086793017E-11));
#28896=CARTESIAN_POINT('Ctrl Pts',(-8.59489616869782,-193.03675111262,4.9622656166752));
#28897=CARTESIAN_POINT('Ctrl Pts',(-5.72993077911996,-192.86175111262,9.92453123332977));
#28898=CARTESIAN_POINT('Ctrl Pts',(1.7871392867044E-11,-192.68675111262,
9.92453123331945));
#28899=CARTESIAN_POINT('Ctrl Pts',(5.7299307791557,-192.51175111262,9.92453123330913));
#28900=CARTESIAN_POINT('Ctrl Pts',(8.59489616871569,-192.33675111262,4.96226561664425));
#28901=CARTESIAN_POINT('Ctrl Pts',(11.4598615582757,-192.16175111262,-2.06354052510241E-11));
#28902=CARTESIAN_POINT('Ctrl Pts',(8.59489616869782,-191.98675111262,-4.9622656166752));
#28903=CARTESIAN_POINT('Ctrl Pts',(5.72993077911996,-191.81175111262,-9.92453123332976));
#28904=CARTESIAN_POINT('Ctrl Pts',(-1.78726082715848E-11,-191.63675111262,
-9.92453123331945));
#28905=CARTESIAN_POINT('Ctrl Pts',(-5.7299307791557,-191.46175111262,-9.92453123330913));
#28906=CARTESIAN_POINT('Ctrl Pts',(-8.59489616871569,-191.28675111262,-4.96226561664425));
#28907=CARTESIAN_POINT('Ctrl Pts',(-11.4598615582757,-191.11175111262,2.06368086793017E-11));
#28908=CARTESIAN_POINT('Ctrl Pts',(-8.59489616869782,-190.93675111262,4.9622656166752));
#28909=CARTESIAN_POINT('Ctrl Pts',(-5.72993077911996,-190.76175111262,9.92453123332977));
#28910=CARTESIAN_POINT('Ctrl Pts',(1.7871392867044E-11,-190.58675111262,
9.92453123331945));
#28911=CARTESIAN_POINT('Ctrl Pts',(5.7299307791557,-190.41175111262,9.92453123330913));
#28912=CARTESIAN_POINT('Ctrl Pts',(8.59489616871569,-190.23675111262,4.96226561664425));
#28913=CARTESIAN_POINT('Ctrl Pts',(11.4598615582757,-190.06175111262,-2.06354052510241E-11));
#28914=CARTESIAN_POINT('Ctrl Pts',(8.59489616869782,-189.88675111262,-4.9622656166752));
#28915=CARTESIAN_POINT('Ctrl Pts',(5.72993077911996,-189.71175111262,-9.92453123332976));
#28916=CARTESIAN_POINT('Ctrl Pts',(-1.78726082715848E-11,-189.53675111262,
-9.92453123331945));
#28917=CARTESIAN_POINT('Ctrl Pts',(-5.7299307791557,-189.36175111262,-9.92453123330913));
#28918=CARTESIAN_POINT('Ctrl Pts',(-8.59489616871569,-189.18675111262,-4.96226561664425));
#28919=CARTESIAN_POINT('Ctrl Pts',(-11.4598615582757,-189.01175111262,2.06368086793017E-11));
#28920=CARTESIAN_POINT('Ctrl Pts',(-8.59489616869782,-188.83675111262,4.9622656166752));
#28921=CARTESIAN_POINT('Ctrl Pts',(-5.72993077911996,-188.66175111262,9.92453123332977));
#28922=CARTESIAN_POINT('Ctrl Pts',(1.7871392867044E-11,-188.48675111262,
9.92453123331945));
#28923=CARTESIAN_POINT('Ctrl Pts',(5.7299307791557,-188.31175111262,9.92453123330913));
#28924=CARTESIAN_POINT('Ctrl Pts',(8.59489616871569,-188.13675111262,4.96226561664425));
#28925=CARTESIAN_POINT('Ctrl Pts',(11.4598615582757,-187.96175111262,-2.06354052510241E-11));
#28926=CARTESIAN_POINT('Ctrl Pts',(8.59489616869782,-187.78675111262,-4.9622656166752));
#28927=CARTESIAN_POINT('Ctrl Pts',(5.72993077911996,-187.61175111262,-9.92453123332976));
#28928=CARTESIAN_POINT('Ctrl Pts',(-1.78726082715848E-11,-187.43675111262,
-9.92453123331945));
#28929=CARTESIAN_POINT('Ctrl Pts',(-5.7299307791557,-187.26175111262,-9.92453123330913));
#28930=CARTESIAN_POINT('Ctrl Pts',(-8.59489616871569,-187.08675111262,-4.96226561664425));
#28931=CARTESIAN_POINT('Ctrl Pts',(-11.4598615582757,-186.91175111262,2.06368086793017E-11));
#28932=CARTESIAN_POINT('Ctrl Pts',(-8.59489616869782,-186.73675111262,4.9622656166752));
#28933=CARTESIAN_POINT('Ctrl Pts',(-5.72993077911996,-186.56175111262,9.92453123332977));
#28934=CARTESIAN_POINT('Ctrl Pts',(1.7871392867044E-11,-186.38675111262,
9.92453123331945));
#28935=CARTESIAN_POINT('Ctrl Pts',(5.7299307791557,-186.21175111262,9.92453123330913));
#28936=CARTESIAN_POINT('Ctrl Pts',(8.59489616871569,-186.03675111262,4.96226561664425));
#28937=CARTESIAN_POINT('Ctrl Pts',(11.4598615582757,-185.86175111262,-2.06354052510241E-11));
#28938=CARTESIAN_POINT('Ctrl Pts',(8.59489616869782,-185.68675111262,-4.9622656166752));
#28939=CARTESIAN_POINT('Ctrl Pts',(5.72993077911996,-185.51175111262,-9.92453123332976));
#28940=CARTESIAN_POINT('Ctrl Pts',(-1.78726082715848E-11,-185.33675111262,
-9.92453123331945));
#28941=CARTESIAN_POINT('Ctrl Pts',(-5.7299307791557,-185.16175111262,-9.92453123330913));
#28942=CARTESIAN_POINT('Ctrl Pts',(-8.59489616871569,-184.98675111262,-4.96226561664425));
#28943=CARTESIAN_POINT('Ctrl Pts',(-11.4598615582757,-184.81175111262,2.06368086793017E-11));
#28944=CARTESIAN_POINT('Ctrl Pts',(-8.59489616869782,-184.63675111262,4.9622656166752));
#28945=CARTESIAN_POINT('Ctrl Pts',(-5.72993077911996,-184.46175111262,9.92453123332977));
#28946=CARTESIAN_POINT('Ctrl Pts',(1.7871392867044E-11,-184.28675111262,
9.92453123331945));
#28947=CARTESIAN_POINT('Ctrl Pts',(5.7299307791557,-184.11175111262,9.92453123330913));
#28948=CARTESIAN_POINT('Ctrl Pts',(8.59489616871569,-183.93675111262,4.96226561664425));
#28949=CARTESIAN_POINT('Ctrl Pts',(11.4598615582757,-183.76175111262,-2.06354052510241E-11));
#28950=CARTESIAN_POINT('Ctrl Pts',(8.59489616869782,-183.58675111262,-4.9622656166752));
#28951=CARTESIAN_POINT('Ctrl Pts',(5.72993077911996,-183.41175111262,-9.92453123332976));
#28952=CARTESIAN_POINT('Ctrl Pts',(-1.78726082715848E-11,-183.23675111262,
-9.92453123331945));
#28953=CARTESIAN_POINT('Ctrl Pts',(-5.7299307791557,-183.06175111262,-9.92453123330913));
#28954=CARTESIAN_POINT('Ctrl Pts',(-8.59489616871569,-182.88675111262,-4.96226561664425));
#28955=CARTESIAN_POINT('Ctrl Pts',(-11.4598615582757,-182.71175111262,2.06368086793017E-11));
#28956=CARTESIAN_POINT('Ctrl Pts',(-8.59489616869782,-182.53675111262,4.9622656166752));
#28957=CARTESIAN_POINT('Ctrl Pts',(-5.72993077911996,-182.36175111262,9.92453123332977));
#28958=CARTESIAN_POINT('Ctrl Pts',(1.7871392867044E-11,-182.18675111262,
9.92453123331945));
#28959=CARTESIAN_POINT('Ctrl Pts',(5.7299307791557,-182.01175111262,9.92453123330913));
#28960=CARTESIAN_POINT('Ctrl Pts',(8.59489616871569,-181.83675111262,4.96226561664425));
#28961=CARTESIAN_POINT('Ctrl Pts',(11.4598615582757,-181.66175111262,-2.06354052510241E-11));
#28962=CARTESIAN_POINT('Ctrl Pts',(8.59489616869782,-181.48675111262,-4.9622656166752));
#28963=CARTESIAN_POINT('Ctrl Pts',(5.72993077911996,-181.31175111262,-9.92453123332976));
#28964=CARTESIAN_POINT('Ctrl Pts',(-1.78726082715848E-11,-181.13675111262,
-9.92453123331945));
#28965=CARTESIAN_POINT('Ctrl Pts',(-5.7299307791557,-180.96175111262,-9.92453123330913));
#28966=CARTESIAN_POINT('Ctrl Pts',(-8.59489616871569,-180.78675111262,-4.96226561664425));
#28967=CARTESIAN_POINT('Ctrl Pts',(-11.4598615582757,-180.61175111262,2.06368086793017E-11));
#28968=CARTESIAN_POINT('Ctrl Pts',(-8.59489616869782,-180.43675111262,4.9622656166752));
#28969=CARTESIAN_POINT('Ctrl Pts',(-5.72993077911996,-180.26175111262,9.92453123332977));
#28970=CARTESIAN_POINT('Ctrl Pts',(1.7871392867044E-11,-180.08675111262,
9.92453123331945));
#28971=CARTESIAN_POINT('Ctrl Pts',(5.7299307791557,-179.91175111262,9.92453123330913));
#28972=CARTESIAN_POINT('Ctrl Pts',(8.59489616871569,-179.73675111262,4.96226561664425));
#28973=CARTESIAN_POINT('Ctrl Pts',(11.4598615582757,-179.56175111262,-2.06354052510241E-11));
#28974=CARTESIAN_POINT('Ctrl Pts',(8.59489616869782,-179.38675111262,-4.9622656166752));
#28975=CARTESIAN_POINT('Ctrl Pts',(5.72993077911996,-179.21175111262,-9.92453123332976));
#28976=CARTESIAN_POINT('Ctrl Pts',(-1.78726082715848E-11,-179.03675111262,
-9.92453123331945));
#28977=CARTESIAN_POINT('Ctrl Pts',(-5.7299307791557,-178.86175111262,-9.92453123330913));
#28978=CARTESIAN_POINT('Ctrl Pts',(-8.59489616871569,-178.68675111262,-4.96226561664425));
#28979=CARTESIAN_POINT('Ctrl Pts',(-11.4598615582757,-178.51175111262,2.06368086793017E-11));
#28980=CARTESIAN_POINT('Ctrl Pts',(-8.59489616869782,-178.33675111262,4.9622656166752));
#28981=CARTESIAN_POINT('Ctrl Pts',(-5.72993077911996,-178.16175111262,9.92453123332977));
#28982=CARTESIAN_POINT('Ctrl Pts',(1.7871392867044E-11,-177.98675111262,
9.92453123331945));
#28983=CARTESIAN_POINT('Ctrl Pts',(5.7299307791557,-177.81175111262,9.92453123330913));
#28984=CARTESIAN_POINT('Ctrl Pts',(8.59489616871569,-177.63675111262,4.96226561664425));
#28985=CARTESIAN_POINT('Ctrl Pts',(11.4598615582757,-177.46175111262,-2.06354052510241E-11));
#28986=CARTESIAN_POINT('Ctrl Pts',(8.59489616869782,-177.28675111262,-4.9622656166752));
#28987=CARTESIAN_POINT('Ctrl Pts',(5.72993077911996,-177.11175111262,-9.92453123332976));
#28988=CARTESIAN_POINT('Ctrl Pts',(-1.78726082715848E-11,-176.93675111262,
-9.92453123331945));
#28989=CARTESIAN_POINT('Ctrl Pts',(-5.7299307791557,-176.76175111262,-9.92453123330913));
#28990=CARTESIAN_POINT('Ctrl Pts',(-8.59489616871569,-176.58675111262,-4.96226561664425));
#28991=CARTESIAN_POINT('Ctrl Pts',(-11.4598615582757,-176.41175111262,2.06368086793017E-11));
#28992=CARTESIAN_POINT('Ctrl Pts',(-8.59489616869782,-176.23675111262,4.9622656166752));
#28993=CARTESIAN_POINT('Ctrl Pts',(-5.72993077911996,-176.06175111262,9.92453123332977));
#28994=CARTESIAN_POINT('Ctrl Pts',(1.7871392867044E-11,-175.88675111262,
9.92453123331945));
#28995=CARTESIAN_POINT('Ctrl Pts',(5.7299307791557,-175.71175111262,9.92453123330913));
#28996=CARTESIAN_POINT('Ctrl Pts',(8.59489616871569,-175.53675111262,4.96226561664425));
#28997=CARTESIAN_POINT('Ctrl Pts',(11.4598615582757,-175.36175111262,-2.06354052510241E-11));
#28998=CARTESIAN_POINT('Ctrl Pts',(8.59489616869782,-175.18675111262,-4.9622656166752));
#28999=CARTESIAN_POINT('Ctrl Pts',(5.72993077911996,-175.01175111262,-9.92453123332976));
#29000=CARTESIAN_POINT('Ctrl Pts',(-1.78726082715848E-11,-174.83675111262,
-9.92453123331945));
#29001=CARTESIAN_POINT('Ctrl Pts',(-5.7299307791557,-174.66175111262,-9.92453123330913));
#29002=CARTESIAN_POINT('Ctrl Pts',(-8.59489616871569,-174.48675111262,-4.96226561664425));
#29003=CARTESIAN_POINT('Ctrl Pts',(-11.4598615582757,-174.31175111262,2.06368086793017E-11));
#29004=CARTESIAN_POINT('Ctrl Pts',(-8.59489616869782,-174.13675111262,4.9622656166752));
#29005=CARTESIAN_POINT('Ctrl Pts',(-5.72993077911996,-173.96175111262,9.92453123332977));
#29006=CARTESIAN_POINT('Ctrl Pts',(1.7871392867044E-11,-173.78675111262,
9.92453123331945));
#29007=CARTESIAN_POINT('Ctrl Pts',(5.7299307791557,-173.61175111262,9.92453123330913));
#29008=CARTESIAN_POINT('Ctrl Pts',(8.59489616871569,-173.43675111262,4.96226561664425));
#29009=CARTESIAN_POINT('Ctrl Pts',(11.4598615582757,-173.26175111262,-2.06354052510241E-11));
#29010=CARTESIAN_POINT('Ctrl Pts',(8.59489616869782,-173.08675111262,-4.9622656166752));
#29011=CARTESIAN_POINT('Ctrl Pts',(5.72993077911996,-172.91175111262,-9.92453123332976));
#29012=CARTESIAN_POINT('Ctrl Pts',(-1.78726082715848E-11,-172.73675111262,
-9.92453123331945));
#29013=CARTESIAN_POINT('Ctrl Pts',(-5.7299307791557,-172.56175111262,-9.92453123330913));
#29014=CARTESIAN_POINT('Ctrl Pts',(-8.59489616871569,-172.38675111262,-4.96226561664425));
#29015=CARTESIAN_POINT('Ctrl Pts',(-11.4598615582757,-172.21175111262,2.06368086793017E-11));
#29016=CARTESIAN_POINT('Ctrl Pts',(-8.59489616869782,-172.03675111262,4.9622656166752));
#29017=CARTESIAN_POINT('Ctrl Pts',(-5.72993077911996,-171.86175111262,9.92453123332977));
#29018=CARTESIAN_POINT('Ctrl Pts',(1.7871392867044E-11,-171.68675111262,
9.92453123331945));
#29019=CARTESIAN_POINT('Ctrl Pts',(5.7299307791557,-171.51175111262,9.92453123330913));
#29020=CARTESIAN_POINT('Ctrl Pts',(8.59489616871569,-171.33675111262,4.96226561664425));
#29021=CARTESIAN_POINT('Ctrl Pts',(11.4598615582757,-171.16175111262,-2.06354052510241E-11));
#29022=CARTESIAN_POINT('Ctrl Pts',(8.59489616869782,-170.98675111262,-4.9622656166752));
#29023=CARTESIAN_POINT('Ctrl Pts',(5.72993077911996,-170.81175111262,-9.92453123332976));
#29024=CARTESIAN_POINT('Ctrl Pts',(-1.78726082715848E-11,-170.63675111262,
-9.92453123331945));
#29025=CARTESIAN_POINT('Ctrl Pts',(-5.7299307791557,-170.46175111262,-9.92453123330913));
#29026=CARTESIAN_POINT('Ctrl Pts',(-8.59489616871569,-170.28675111262,-4.96226561664425));
#29027=CARTESIAN_POINT('Ctrl Pts',(-11.4598615582757,-170.11175111262,2.06368086793017E-11));
#29028=CARTESIAN_POINT('Ctrl Pts',(-8.59489616869782,-169.93675111262,4.9622656166752));
#29029=CARTESIAN_POINT('Ctrl Pts',(-5.72993077911996,-169.76175111262,9.92453123332977));
#29030=CARTESIAN_POINT('Ctrl Pts',(1.7871392867044E-11,-169.58675111262,
9.92453123331945));
#29031=CARTESIAN_POINT('Ctrl Pts',(5.7299307791557,-169.41175111262,9.92453123330913));
#29032=CARTESIAN_POINT('Ctrl Pts',(8.59489616871569,-169.23675111262,4.96226561664425));
#29033=CARTESIAN_POINT('Ctrl Pts',(11.4598615582757,-169.06175111262,-2.06354052510241E-11));
#29034=CARTESIAN_POINT('Ctrl Pts',(8.59489616869782,-168.88675111262,-4.9622656166752));
#29035=CARTESIAN_POINT('Ctrl Pts',(5.72993077911996,-168.71175111262,-9.92453123332976));
#29036=CARTESIAN_POINT('Ctrl Pts',(-1.78726082715848E-11,-168.53675111262,
-9.92453123331945));
#29037=CARTESIAN_POINT('Ctrl Pts',(-5.7299307791557,-168.36175111262,-9.92453123330913));
#29038=CARTESIAN_POINT('Ctrl Pts',(-8.59489616871569,-168.18675111262,-4.96226561664425));
#29039=CARTESIAN_POINT('Ctrl Pts',(-11.4598615582757,-168.01175111262,2.06368086793017E-11));
#29040=CARTESIAN_POINT('Ctrl Pts',(-8.59489616869782,-167.83675111262,4.9622656166752));
#29041=CARTESIAN_POINT('Ctrl Pts',(-5.72993077911996,-167.66175111262,9.92453123332977));
#29042=CARTESIAN_POINT('Ctrl Pts',(1.7871392867044E-11,-167.48675111262,
9.92453123331945));
#29043=CARTESIAN_POINT('Ctrl Pts',(5.7299307791557,-167.31175111262,9.92453123330913));
#29044=CARTESIAN_POINT('Ctrl Pts',(8.59489616871569,-167.13675111262,4.96226561664425));
#29045=CARTESIAN_POINT('Ctrl Pts',(11.4598615582757,-166.96175111262,-2.06354052510241E-11));
#29046=CARTESIAN_POINT('Ctrl Pts',(8.59489616869782,-166.78675111262,-4.9622656166752));
#29047=CARTESIAN_POINT('Ctrl Pts',(5.72993077911996,-166.61175111262,-9.92453123332976));
#29048=CARTESIAN_POINT('Ctrl Pts',(-1.78726082715848E-11,-166.43675111262,
-9.92453123331945));
#29049=CARTESIAN_POINT('Ctrl Pts',(-5.7299307791557,-166.26175111262,-9.92453123330913));
#29050=CARTESIAN_POINT('Ctrl Pts',(-8.59489616871569,-166.08675111262,-4.96226561664425));
#29051=CARTESIAN_POINT('Ctrl Pts',(-11.4598615582757,-165.91175111262,2.06368086793017E-11));
#29052=CARTESIAN_POINT('Ctrl Pts',(-8.59489616869782,-165.73675111262,4.9622656166752));
#29053=CARTESIAN_POINT('Ctrl Pts',(-5.72993077911996,-165.56175111262,9.92453123332977));
#29054=CARTESIAN_POINT('Ctrl Pts',(1.7871392867044E-11,-165.38675111262,
9.92453123331945));
#29055=CARTESIAN_POINT('Ctrl Pts',(5.7299307791557,-165.21175111262,9.92453123330913));
#29056=CARTESIAN_POINT('Ctrl Pts',(8.59489616871569,-165.03675111262,4.96226561664425));
#29057=CARTESIAN_POINT('Ctrl Pts',(11.4598615582757,-164.86175111262,-2.06354052510241E-11));
#29058=CARTESIAN_POINT('Ctrl Pts',(8.59489616869782,-164.68675111262,-4.9622656166752));
#29059=CARTESIAN_POINT('Ctrl Pts',(5.72993077911996,-164.51175111262,-9.92453123332976));
#29060=CARTESIAN_POINT('Ctrl Pts',(-1.78726082715848E-11,-164.33675111262,
-9.92453123331945));
#29061=CARTESIAN_POINT('Ctrl Pts',(-5.7299307791557,-164.16175111262,-9.92453123330913));
#29062=CARTESIAN_POINT('Ctrl Pts',(-8.59489616871569,-163.98675111262,-4.96226561664425));
#29063=CARTESIAN_POINT('Ctrl Pts',(-11.4598615582757,-163.81175111262,2.06368086793017E-11));
#29064=CARTESIAN_POINT('Ctrl Pts',(-8.59489616869782,-163.63675111262,4.9622656166752));
#29065=CARTESIAN_POINT('Ctrl Pts',(-5.72993077911996,-163.46175111262,9.92453123332977));
#29066=CARTESIAN_POINT('Ctrl Pts',(1.7871392867044E-11,-163.28675111262,
9.92453123331945));
#29067=CARTESIAN_POINT('Ctrl Pts',(5.7299307791557,-163.11175111262,9.92453123330913));
#29068=CARTESIAN_POINT('Ctrl Pts',(8.59489616871569,-162.93675111262,4.96226561664425));
#29069=CARTESIAN_POINT('Ctrl Pts',(11.4598615582757,-162.76175111262,-2.06354052510241E-11));
#29070=CARTESIAN_POINT('Ctrl Pts',(8.59489616869782,-162.58675111262,-4.9622656166752));
#29071=CARTESIAN_POINT('Ctrl Pts',(5.72993077911996,-162.41175111262,-9.92453123332976));
#29072=CARTESIAN_POINT('Ctrl Pts',(-1.78726082715848E-11,-162.23675111262,
-9.92453123331945));
#29073=CARTESIAN_POINT('Ctrl Pts',(-5.7299307791557,-162.06175111262,-9.92453123330913));
#29074=CARTESIAN_POINT('Ctrl Pts',(-8.59489616871569,-161.88675111262,-4.96226561664425));
#29075=CARTESIAN_POINT('Ctrl Pts',(-11.4598615582757,-161.71175111262,2.06368086793017E-11));
#29076=CARTESIAN_POINT('Ctrl Pts',(-8.59489616869782,-161.53675111262,4.9622656166752));
#29077=CARTESIAN_POINT('Ctrl Pts',(-5.72993077911996,-161.36175111262,9.92453123332977));
#29078=CARTESIAN_POINT('Ctrl Pts',(1.7871392867044E-11,-161.18675111262,
9.92453123331945));
#29079=CARTESIAN_POINT('Ctrl Pts',(5.7299307791557,-161.01175111262,9.92453123330913));
#29080=CARTESIAN_POINT('Ctrl Pts',(8.59489616871569,-160.83675111262,4.96226561664425));
#29081=CARTESIAN_POINT('Ctrl Pts',(11.4598615582757,-160.66175111262,-2.06354052510241E-11));
#29082=CARTESIAN_POINT('Ctrl Pts',(8.59489616869782,-160.48675111262,-4.9622656166752));
#29083=CARTESIAN_POINT('Ctrl Pts',(5.72993077911996,-160.31175111262,-9.92453123332976));
#29084=CARTESIAN_POINT('Ctrl Pts',(-1.78726082715848E-11,-160.13675111262,
-9.92453123331945));
#29085=CARTESIAN_POINT('Ctrl Pts',(-5.7299307791557,-159.96175111262,-9.92453123330913));
#29086=CARTESIAN_POINT('Ctrl Pts',(-8.59489616871569,-159.78675111262,-4.96226561664425));
#29087=CARTESIAN_POINT('Ctrl Pts',(-11.4598615582757,-159.61175111262,2.06368086793017E-11));
#29088=CARTESIAN_POINT('Ctrl Pts',(-8.59489616869782,-159.43675111262,4.9622656166752));
#29089=CARTESIAN_POINT('Ctrl Pts',(-5.72993077911996,-159.26175111262,9.92453123332977));
#29090=CARTESIAN_POINT('Ctrl Pts',(1.7871392867044E-11,-159.08675111262,
9.92453123331945));
#29091=CARTESIAN_POINT('Ctrl Pts',(5.7299307791557,-158.91175111262,9.92453123330913));
#29092=CARTESIAN_POINT('Ctrl Pts',(8.59489616871569,-158.73675111262,4.96226561664425));
#29093=CARTESIAN_POINT('Ctrl Pts',(11.4598615582757,-158.56175111262,-2.06354052510241E-11));
#29094=CARTESIAN_POINT('Ctrl Pts',(8.59489616869782,-158.38675111262,-4.9622656166752));
#29095=CARTESIAN_POINT('Ctrl Pts',(5.72993077911996,-158.21175111262,-9.92453123332976));
#29096=CARTESIAN_POINT('Ctrl Pts',(-1.78726082715848E-11,-158.03675111262,
-9.92453123331945));
#29097=CARTESIAN_POINT('Ctrl Pts',(-5.7299307791557,-157.86175111262,-9.92453123330913));
#29098=CARTESIAN_POINT('Ctrl Pts',(-8.59489616871569,-157.68675111262,-4.96226561664425));
#29099=CARTESIAN_POINT('Ctrl Pts',(-11.4598615582757,-157.51175111262,2.06368086793017E-11));
#29100=CARTESIAN_POINT('Ctrl Pts',(-8.59489616869782,-157.33675111262,4.9622656166752));
#29101=CARTESIAN_POINT('Ctrl Pts',(-5.72993077911996,-157.16175111262,9.92453123332977));
#29102=CARTESIAN_POINT('Ctrl Pts',(1.7871392867044E-11,-156.98675111262,
9.92453123331945));
#29103=CARTESIAN_POINT('Ctrl Pts',(5.7299307791557,-156.81175111262,9.92453123330913));
#29104=CARTESIAN_POINT('Ctrl Pts',(8.59489616871569,-156.63675111262,4.96226561664425));
#29105=CARTESIAN_POINT('Ctrl Pts',(11.4598615582757,-156.46175111262,-2.06354052510241E-11));
#29106=CARTESIAN_POINT('Ctrl Pts',(8.59489616869782,-156.28675111262,-4.9622656166752));
#29107=CARTESIAN_POINT('Ctrl Pts',(5.72993077911996,-156.11175111262,-9.92453123332976));
#29108=CARTESIAN_POINT('Ctrl Pts',(-1.78726082715848E-11,-155.93675111262,
-9.92453123331945));
#29109=CARTESIAN_POINT('Ctrl Pts',(-5.7299307791557,-155.76175111262,-9.92453123330913));
#29110=CARTESIAN_POINT('Ctrl Pts',(-8.59489616871569,-155.58675111262,-4.96226561664425));
#29111=CARTESIAN_POINT('Ctrl Pts',(-11.4598615582757,-155.41175111262,2.06368086793017E-11));
#29112=CARTESIAN_POINT('Ctrl Pts',(-8.59489616869782,-155.23675111262,4.9622656166752));
#29113=CARTESIAN_POINT('Ctrl Pts',(-5.72993077911996,-155.06175111262,9.92453123332977));
#29114=CARTESIAN_POINT('Ctrl Pts',(1.7871392867044E-11,-154.88675111262,
9.92453123331945));
#29115=CARTESIAN_POINT('Ctrl Pts',(5.7299307791557,-154.71175111262,9.92453123330913));
#29116=CARTESIAN_POINT('Ctrl Pts',(8.59489616871569,-154.53675111262,4.96226561664425));
#29117=CARTESIAN_POINT('Ctrl Pts',(11.4598615582757,-154.36175111262,-2.06354052510241E-11));
#29118=CARTESIAN_POINT('Ctrl Pts',(8.59489616869782,-154.18675111262,-4.9622656166752));
#29119=CARTESIAN_POINT('Ctrl Pts',(5.72993077911996,-154.01175111262,-9.92453123332976));
#29120=CARTESIAN_POINT('Ctrl Pts',(-1.78726082715848E-11,-153.83675111262,
-9.92453123331945));
#29121=CARTESIAN_POINT('Ctrl Pts',(-5.7299307791557,-153.66175111262,-9.92453123330913));
#29122=CARTESIAN_POINT('Ctrl Pts',(-8.59489616871569,-153.48675111262,-4.96226561664425));
#29123=CARTESIAN_POINT('Ctrl Pts',(-11.4598615582757,-153.31175111262,2.06368086793017E-11));
#29124=CARTESIAN_POINT('Ctrl Pts',(-8.59489616869782,-153.13675111262,4.9622656166752));
#29125=CARTESIAN_POINT('Ctrl Pts',(-5.72993077911996,-152.96175111262,9.92453123332977));
#29126=CARTESIAN_POINT('Ctrl Pts',(1.7871392867044E-11,-152.78675111262,
9.92453123331945));
#29127=CARTESIAN_POINT('Ctrl Pts',(5.7299307791557,-152.61175111262,9.92453123330913));
#29128=CARTESIAN_POINT('Ctrl Pts',(8.59489616871569,-152.43675111262,4.96226561664425));
#29129=CARTESIAN_POINT('Ctrl Pts',(11.4598615582757,-152.26175111262,-2.06354052510241E-11));
#29130=CARTESIAN_POINT('Ctrl Pts',(8.59489616869782,-152.08675111262,-4.9622656166752));
#29131=CARTESIAN_POINT('Ctrl Pts',(5.72993077911996,-151.91175111262,-9.92453123332976));
#29132=CARTESIAN_POINT('Ctrl Pts',(-1.78726082715848E-11,-151.73675111262,
-9.92453123331945));
#29133=CARTESIAN_POINT('Ctrl Pts',(-5.7299307791557,-151.56175111262,-9.92453123330913));
#29134=CARTESIAN_POINT('Ctrl Pts',(-8.59489616871569,-151.38675111262,-4.96226561664425));
#29135=CARTESIAN_POINT('Ctrl Pts',(-11.4598615582757,-151.21175111262,2.06368086793017E-11));
#29136=CARTESIAN_POINT('Ctrl Pts',(-8.59489616869782,-151.03675111262,4.9622656166752));
#29137=CARTESIAN_POINT('Ctrl Pts',(-5.72993077911996,-150.86175111262,9.92453123332977));
#29138=CARTESIAN_POINT('Ctrl Pts',(1.7871392867044E-11,-150.68675111262,
9.92453123331945));
#29139=CARTESIAN_POINT('Ctrl Pts',(5.7299307791557,-150.51175111262,9.92453123330913));
#29140=CARTESIAN_POINT('Ctrl Pts',(8.59489616871569,-150.33675111262,4.96226561664425));
#29141=CARTESIAN_POINT('Ctrl Pts',(11.4598615582757,-150.16175111262,-2.06354052510241E-11));
#29142=CARTESIAN_POINT('Ctrl Pts',(8.59489616869782,-149.98675111262,-4.9622656166752));
#29143=CARTESIAN_POINT('Ctrl Pts',(5.72993077911996,-149.81175111262,-9.92453123332976));
#29144=CARTESIAN_POINT('Ctrl Pts',(-1.78726082715848E-11,-149.63675111262,
-9.92453123331945));
#29145=CARTESIAN_POINT('Ctrl Pts',(-5.7299307791557,-149.46175111262,-9.92453123330913));
#29146=CARTESIAN_POINT('Ctrl Pts',(-8.59489616871569,-149.28675111262,-4.96226561664425));
#29147=CARTESIAN_POINT('Ctrl Pts',(-11.4598615582757,-149.11175111262,2.06368086793017E-11));
#29148=CARTESIAN_POINT('Ctrl Pts',(-8.59489616869782,-148.93675111262,4.9622656166752));
#29149=CARTESIAN_POINT('Ctrl Pts',(-5.72993077911996,-148.76175111262,9.92453123332977));
#29150=CARTESIAN_POINT('Ctrl Pts',(1.7871392867044E-11,-148.58675111262,
9.92453123331945));
#29151=CARTESIAN_POINT('Ctrl Pts',(5.7299307791557,-148.41175111262,9.92453123330913));
#29152=CARTESIAN_POINT('Ctrl Pts',(8.59489616871569,-148.23675111262,4.96226561664425));
#29153=CARTESIAN_POINT('Ctrl Pts',(11.4598615582757,-148.06175111262,-2.06354052510241E-11));
#29154=CARTESIAN_POINT('Ctrl Pts',(8.59489616869782,-147.88675111262,-4.9622656166752));
#29155=CARTESIAN_POINT('Ctrl Pts',(5.72993077911996,-147.71175111262,-9.92453123332976));
#29156=CARTESIAN_POINT('Ctrl Pts',(-1.78726082715848E-11,-147.53675111262,
-9.92453123331945));
#29157=CARTESIAN_POINT('Ctrl Pts',(-5.7299307791557,-147.36175111262,-9.92453123330913));
#29158=CARTESIAN_POINT('Ctrl Pts',(-8.59489616871569,-147.18675111262,-4.96226561664425));
#29159=CARTESIAN_POINT('Ctrl Pts',(-11.4598615582757,-147.01175111262,2.06368086793017E-11));
#29160=CARTESIAN_POINT('Ctrl Pts',(-8.59489616869782,-146.83675111262,4.9622656166752));
#29161=CARTESIAN_POINT('Ctrl Pts',(-5.72993077911996,-146.66175111262,9.92453123332977));
#29162=CARTESIAN_POINT('Ctrl Pts',(1.7871392867044E-11,-146.48675111262,
9.92453123331945));
#29163=CARTESIAN_POINT('Ctrl Pts',(5.7299307791557,-146.31175111262,9.92453123330913));
#29164=CARTESIAN_POINT('Ctrl Pts',(8.59489616871569,-146.13675111262,4.96226561664425));
#29165=CARTESIAN_POINT('Ctrl Pts',(11.4598615582757,-145.96175111262,-2.06354052510241E-11));
#29166=CARTESIAN_POINT('Ctrl Pts',(8.59489616869782,-145.78675111262,-4.9622656166752));
#29167=CARTESIAN_POINT('Ctrl Pts',(5.72993077911996,-145.61175111262,-9.92453123332976));
#29168=CARTESIAN_POINT('Ctrl Pts',(-1.78726082715848E-11,-145.43675111262,
-9.92453123331945));
#29169=CARTESIAN_POINT('Ctrl Pts',(-5.7299307791557,-145.26175111262,-9.92453123330913));
#29170=CARTESIAN_POINT('Ctrl Pts',(-8.59489616871569,-145.08675111262,-4.96226561664425));
#29171=CARTESIAN_POINT('Ctrl Pts',(-11.4598615582757,-144.91175111262,2.06368086793017E-11));
#29172=CARTESIAN_POINT('Ctrl Pts',(-8.59489616869782,-144.73675111262,4.9622656166752));
#29173=CARTESIAN_POINT('Ctrl Pts',(-5.72993077911996,-144.56175111262,9.92453123332977));
#29174=CARTESIAN_POINT('Ctrl Pts',(1.7871392867044E-11,-144.38675111262,
9.92453123331945));
#29175=CARTESIAN_POINT('Ctrl Pts',(5.7299307791557,-144.21175111262,9.92453123330913));
#29176=CARTESIAN_POINT('Ctrl Pts',(8.59489616871569,-144.03675111262,4.96226561664425));
#29177=CARTESIAN_POINT('Ctrl Pts',(11.4598615582757,-143.86175111262,-2.06354052510241E-11));
#29178=CARTESIAN_POINT('Ctrl Pts',(8.59489616869782,-143.68675111262,-4.9622656166752));
#29179=CARTESIAN_POINT('Ctrl Pts',(5.72993077911996,-143.51175111262,-9.92453123332976));
#29180=CARTESIAN_POINT('Ctrl Pts',(-1.78726082715848E-11,-143.33675111262,
-9.92453123331945));
#29181=CARTESIAN_POINT('Ctrl Pts',(-5.7299307791557,-143.16175111262,-9.92453123330913));
#29182=CARTESIAN_POINT('Ctrl Pts',(-8.59489616871569,-142.98675111262,-4.96226561664425));
#29183=CARTESIAN_POINT('Ctrl Pts',(-11.4598615582757,-142.81175111262,2.06368086793017E-11));
#29184=CARTESIAN_POINT('Ctrl Pts',(-8.59489616869782,-142.63675111262,4.9622656166752));
#29185=CARTESIAN_POINT('Ctrl Pts',(-5.72993077911996,-142.46175111262,9.92453123332977));
#29186=CARTESIAN_POINT('Ctrl Pts',(1.7871392867044E-11,-142.28675111262,
9.92453123331945));
#29187=CARTESIAN_POINT('Ctrl Pts',(5.7299307791557,-142.11175111262,9.92453123330913));
#29188=CARTESIAN_POINT('Ctrl Pts',(8.59489616871569,-141.93675111262,4.96226561664425));
#29189=CARTESIAN_POINT('Ctrl Pts',(11.4598615582757,-141.76175111262,-2.06354052510241E-11));
#29190=CARTESIAN_POINT('Ctrl Pts',(8.59489616869782,-141.58675111262,-4.9622656166752));
#29191=CARTESIAN_POINT('Ctrl Pts',(5.72993077911996,-141.41175111262,-9.92453123332976));
#29192=CARTESIAN_POINT('Ctrl Pts',(-1.78726082715848E-11,-141.23675111262,
-9.92453123331945));
#29193=CARTESIAN_POINT('Ctrl Pts',(-5.7299307791557,-141.06175111262,-9.92453123330913));
#29194=CARTESIAN_POINT('Ctrl Pts',(-8.59489616871569,-140.88675111262,-4.96226561664425));
#29195=CARTESIAN_POINT('Ctrl Pts',(-11.4598615582757,-140.71175111262,2.06368086793017E-11));
#29196=CARTESIAN_POINT('Ctrl Pts',(-8.59489616869782,-140.53675111262,4.9622656166752));
#29197=CARTESIAN_POINT('Ctrl Pts',(-5.72993077911996,-140.36175111262,9.92453123332977));
#29198=CARTESIAN_POINT('Ctrl Pts',(1.7871392867044E-11,-140.18675111262,
9.92453123331945));
#29199=CARTESIAN_POINT('Ctrl Pts',(5.7299307791557,-140.01175111262,9.92453123330913));
#29200=CARTESIAN_POINT('Ctrl Pts',(8.59489616871569,-139.83675111262,4.96226561664425));
#29201=CARTESIAN_POINT('Ctrl Pts',(11.4598615582757,-139.66175111262,-2.06354052510241E-11));
#29202=CARTESIAN_POINT('Ctrl Pts',(8.59489616869782,-139.48675111262,-4.9622656166752));
#29203=CARTESIAN_POINT('Ctrl Pts',(5.72993077911996,-139.31175111262,-9.92453123332976));
#29204=CARTESIAN_POINT('Ctrl Pts',(-1.78726082715848E-11,-139.13675111262,
-9.92453123331945));
#29205=CARTESIAN_POINT('Ctrl Pts',(-5.7299307791557,-138.96175111262,-9.92453123330913));
#29206=CARTESIAN_POINT('Ctrl Pts',(-8.59489616871569,-138.78675111262,-4.96226561664425));
#29207=CARTESIAN_POINT('Ctrl Pts',(-11.4598615582757,-138.61175111262,2.06368086793017E-11));
#29208=CARTESIAN_POINT('Ctrl Pts',(-8.59489616869782,-138.43675111262,4.9622656166752));
#29209=CARTESIAN_POINT('Ctrl Pts',(-5.72993077911996,-138.26175111262,9.92453123332977));
#29210=CARTESIAN_POINT('Ctrl Pts',(1.7871392867044E-11,-138.08675111262,
9.92453123331945));
#29211=CARTESIAN_POINT('Ctrl Pts',(5.7299307791557,-137.91175111262,9.92453123330913));
#29212=CARTESIAN_POINT('Ctrl Pts',(8.59489616871569,-137.73675111262,4.96226561664425));
#29213=CARTESIAN_POINT('Ctrl Pts',(11.4598615582757,-137.56175111262,-2.06354052510241E-11));
#29214=CARTESIAN_POINT('Ctrl Pts',(8.59489616869782,-137.38675111262,-4.9622656166752));
#29215=CARTESIAN_POINT('Ctrl Pts',(5.72993077911996,-137.21175111262,-9.92453123332976));
#29216=CARTESIAN_POINT('Ctrl Pts',(-1.78726082715848E-11,-137.03675111262,
-9.92453123331945));
#29217=CARTESIAN_POINT('Ctrl Pts',(-5.7299307791557,-136.86175111262,-9.92453123330913));
#29218=CARTESIAN_POINT('Ctrl Pts',(-8.59489616871569,-136.68675111262,-4.96226561664425));
#29219=CARTESIAN_POINT('Ctrl Pts',(-11.4598615582757,-136.51175111262,2.06368086793017E-11));
#29220=CARTESIAN_POINT('Ctrl Pts',(-8.59489616869782,-136.33675111262,4.9622656166752));
#29221=CARTESIAN_POINT('Ctrl Pts',(-5.72993077911996,-136.16175111262,9.92453123332977));
#29222=CARTESIAN_POINT('Ctrl Pts',(1.7871392867044E-11,-135.98675111262,
9.92453123331945));
#29223=CARTESIAN_POINT('Ctrl Pts',(5.7299307791557,-135.81175111262,9.92453123330913));
#29224=CARTESIAN_POINT('Ctrl Pts',(8.59489616871569,-135.63675111262,4.96226561664425));
#29225=CARTESIAN_POINT('Ctrl Pts',(11.4598615582757,-135.46175111262,-2.06354052510241E-11));
#29226=CARTESIAN_POINT('Ctrl Pts',(8.59489616869782,-135.28675111262,-4.9622656166752));
#29227=CARTESIAN_POINT('Ctrl Pts',(5.72993077911996,-135.11175111262,-9.92453123332976));
#29228=CARTESIAN_POINT('Ctrl Pts',(-1.78726082715848E-11,-134.93675111262,
-9.92453123331945));
#29229=CARTESIAN_POINT('Ctrl Pts',(-5.7299307791557,-134.76175111262,-9.92453123330913));
#29230=CARTESIAN_POINT('Ctrl Pts',(-8.59489616871569,-134.58675111262,-4.96226561664425));
#29231=CARTESIAN_POINT('Ctrl Pts',(-11.4598615582757,-134.41175111262,2.06368086793017E-11));
#29232=CARTESIAN_POINT('Ctrl Pts',(-8.59489616869782,-134.23675111262,4.9622656166752));
#29233=CARTESIAN_POINT('Ctrl Pts',(-5.72993077911996,-134.06175111262,9.92453123332977));
#29234=CARTESIAN_POINT('Ctrl Pts',(1.7871392867044E-11,-133.88675111262,
9.92453123331945));
#29235=CARTESIAN_POINT('Ctrl Pts',(5.7299307791557,-133.71175111262,9.92453123330913));
#29236=CARTESIAN_POINT('Ctrl Pts',(8.59489616871569,-133.53675111262,4.96226561664425));
#29237=CARTESIAN_POINT('Ctrl Pts',(11.4598615582757,-133.36175111262,-2.06354052510241E-11));
#29238=CARTESIAN_POINT('Ctrl Pts',(8.59489616869782,-133.18675111262,-4.9622656166752));
#29239=CARTESIAN_POINT('Ctrl Pts',(5.72993077911996,-133.01175111262,-9.92453123332976));
#29240=CARTESIAN_POINT('Ctrl Pts',(-1.78726082715848E-11,-132.83675111262,
-9.92453123331945));
#29241=CARTESIAN_POINT('Ctrl Pts',(-5.7299307791557,-132.66175111262,-9.92453123330913));
#29242=CARTESIAN_POINT('Ctrl Pts',(-8.59489616871569,-132.48675111262,-4.96226561664425));
#29243=CARTESIAN_POINT('Ctrl Pts',(-11.4598615582757,-132.31175111262,2.06368086793017E-11));
#29244=CARTESIAN_POINT('Ctrl Pts',(-8.59489616869782,-132.13675111262,4.9622656166752));
#29245=CARTESIAN_POINT('Ctrl Pts',(-5.72993077911996,-131.96175111262,9.92453123332977));
#29246=CARTESIAN_POINT('Ctrl Pts',(1.7871392867044E-11,-131.78675111262,
9.92453123331945));
#29247=CARTESIAN_POINT('Ctrl Pts',(5.7299307791557,-131.61175111262,9.92453123330913));
#29248=CARTESIAN_POINT('Ctrl Pts',(8.59489616871569,-131.43675111262,4.96226561664425));
#29249=CARTESIAN_POINT('Ctrl Pts',(11.4598615582757,-131.26175111262,-2.06354052510241E-11));
#29250=CARTESIAN_POINT('Ctrl Pts',(8.59489616869782,-131.08675111262,-4.9622656166752));
#29251=CARTESIAN_POINT('Ctrl Pts',(5.72993077911996,-130.91175111262,-9.92453123332976));
#29252=CARTESIAN_POINT('Ctrl Pts',(-1.78726082715848E-11,-130.73675111262,
-9.92453123331945));
#29253=CARTESIAN_POINT('Ctrl Pts',(-5.7299307791557,-130.56175111262,-9.92453123330913));
#29254=CARTESIAN_POINT('Ctrl Pts',(-8.59489616871569,-130.38675111262,-4.96226561664425));
#29255=CARTESIAN_POINT('Ctrl Pts',(-11.4598615582757,-130.21175111262,2.06368086793017E-11));
#29256=CARTESIAN_POINT('Ctrl Pts',(-8.59489616869782,-130.03675111262,4.9622656166752));
#29257=CARTESIAN_POINT('Ctrl Pts',(-5.72993077911996,-129.86175111262,9.92453123332977));
#29258=CARTESIAN_POINT('Ctrl Pts',(1.7871392867044E-11,-129.68675111262,
9.92453123331945));
#29259=CARTESIAN_POINT('Ctrl Pts',(5.7299307791557,-129.51175111262,9.92453123330913));
#29260=CARTESIAN_POINT('Ctrl Pts',(8.59489616871569,-129.33675111262,4.96226561664425));
#29261=CARTESIAN_POINT('Ctrl Pts',(11.4598615582757,-129.16175111262,-2.06354052510241E-11));
#29262=CARTESIAN_POINT('Ctrl Pts',(8.59489616869782,-128.98675111262,-4.9622656166752));
#29263=CARTESIAN_POINT('Ctrl Pts',(5.72993077911996,-128.81175111262,-9.92453123332976));
#29264=CARTESIAN_POINT('Ctrl Pts',(-1.78726082715848E-11,-128.63675111262,
-9.92453123331945));
#29265=CARTESIAN_POINT('Ctrl Pts',(-5.7299307791557,-128.46175111262,-9.92453123330913));
#29266=CARTESIAN_POINT('Ctrl Pts',(-8.59489616871569,-128.28675111262,-4.96226561664425));
#29267=CARTESIAN_POINT('Ctrl Pts',(-11.4598615582757,-128.11175111262,2.06368086793017E-11));
#29268=CARTESIAN_POINT('Ctrl Pts',(-8.59489616869782,-127.93675111262,4.9622656166752));
#29269=CARTESIAN_POINT('Ctrl Pts',(-5.72993077911996,-127.76175111262,9.92453123332977));
#29270=CARTESIAN_POINT('Ctrl Pts',(1.7871392867044E-11,-127.58675111262,
9.92453123331945));
#29271=CARTESIAN_POINT('Ctrl Pts',(5.7299307791557,-127.41175111262,9.92453123330913));
#29272=CARTESIAN_POINT('Ctrl Pts',(8.59489616871569,-127.23675111262,4.96226561664425));
#29273=CARTESIAN_POINT('Ctrl Pts',(11.4598615582757,-127.06175111262,-2.06354052510241E-11));
#29274=CARTESIAN_POINT('Ctrl Pts',(8.59489616869782,-126.88675111262,-4.9622656166752));
#29275=CARTESIAN_POINT('Ctrl Pts',(5.72993077911996,-126.71175111262,-9.92453123332976));
#29276=CARTESIAN_POINT('Ctrl Pts',(-1.78726082715848E-11,-126.53675111262,
-9.92453123331945));
#29277=CARTESIAN_POINT('Ctrl Pts',(-5.7299307791557,-126.36175111262,-9.92453123330913));
#29278=CARTESIAN_POINT('Ctrl Pts',(-8.59489616871569,-126.18675111262,-4.96226561664425));
#29279=CARTESIAN_POINT('Ctrl Pts',(-11.4598615582757,-126.01175111262,2.06368086793017E-11));
#29280=CARTESIAN_POINT('Ctrl Pts',(-8.59489616869782,-125.83675111262,4.9622656166752));
#29281=CARTESIAN_POINT('Ctrl Pts',(-5.72993077911996,-125.66175111262,9.92453123332977));
#29282=CARTESIAN_POINT('Ctrl Pts',(1.7871392867044E-11,-125.48675111262,
9.92453123331945));
#29283=CARTESIAN_POINT('Ctrl Pts',(5.7299307791557,-125.31175111262,9.92453123330913));
#29284=CARTESIAN_POINT('Ctrl Pts',(8.59489616871569,-125.13675111262,4.96226561664425));
#29285=CARTESIAN_POINT('Ctrl Pts',(11.4598615582757,-124.96175111262,-2.06354052510241E-11));
#29286=CARTESIAN_POINT('Ctrl Pts',(8.59489616869782,-124.78675111262,-4.9622656166752));
#29287=CARTESIAN_POINT('Ctrl Pts',(5.72993077911996,-124.61175111262,-9.92453123332976));
#29288=CARTESIAN_POINT('Ctrl Pts',(-1.78726082715848E-11,-124.43675111262,
-9.92453123331945));
#29289=CARTESIAN_POINT('Ctrl Pts',(-5.7299307791557,-124.26175111262,-9.92453123330913));
#29290=CARTESIAN_POINT('Ctrl Pts',(-8.59489616871569,-124.08675111262,-4.96226561664425));
#29291=CARTESIAN_POINT('Ctrl Pts',(-11.4598615582757,-123.91175111262,2.06368086793017E-11));
#29292=CARTESIAN_POINT('Ctrl Pts',(-8.59489616869782,-123.73675111262,4.9622656166752));
#29293=CARTESIAN_POINT('Ctrl Pts',(-5.72993077911996,-123.56175111262,9.92453123332977));
#29294=CARTESIAN_POINT('Ctrl Pts',(1.7871392867044E-11,-123.38675111262,
9.92453123331945));
#29295=CARTESIAN_POINT('Ctrl Pts',(5.7299307791557,-123.21175111262,9.92453123330913));
#29296=CARTESIAN_POINT('Ctrl Pts',(8.59489616871569,-123.03675111262,4.96226561664425));
#29297=CARTESIAN_POINT('Ctrl Pts',(11.4598615582757,-122.86175111262,-2.06354052510241E-11));
#29298=CARTESIAN_POINT('Ctrl Pts',(8.59489616869782,-122.68675111262,-4.9622656166752));
#29299=CARTESIAN_POINT('Ctrl Pts',(5.72993077911996,-122.51175111262,-9.92453123332976));
#29300=CARTESIAN_POINT('Ctrl Pts',(-1.78726082715848E-11,-122.33675111262,
-9.92453123331945));
#29301=CARTESIAN_POINT('Ctrl Pts',(-5.7299307791557,-122.16175111262,-9.92453123330913));
#29302=CARTESIAN_POINT('Ctrl Pts',(-8.59489616871569,-121.98675111262,-4.96226561664425));
#29303=CARTESIAN_POINT('Ctrl Pts',(-11.4598615582757,-121.81175111262,2.06368086793017E-11));
#29304=CARTESIAN_POINT('Ctrl Pts',(-8.59489616869782,-121.63675111262,4.9622656166752));
#29305=CARTESIAN_POINT('Ctrl Pts',(-5.72993077911996,-121.46175111262,9.92453123332977));
#29306=CARTESIAN_POINT('Ctrl Pts',(1.7871392867044E-11,-121.28675111262,
9.92453123331945));
#29307=CARTESIAN_POINT('Ctrl Pts',(5.7299307791557,-121.11175111262,9.92453123330913));
#29308=CARTESIAN_POINT('Ctrl Pts',(8.59489616871569,-120.93675111262,4.96226561664425));
#29309=CARTESIAN_POINT('Ctrl Pts',(11.4598615582757,-120.76175111262,-2.06354052510241E-11));
#29310=CARTESIAN_POINT('Ctrl Pts',(8.59489616869782,-120.58675111262,-4.9622656166752));
#29311=CARTESIAN_POINT('Ctrl Pts',(5.72993077911996,-120.41175111262,-9.92453123332976));
#29312=CARTESIAN_POINT('Ctrl Pts',(-1.78726082715848E-11,-120.23675111262,
-9.92453123331945));
#29313=CARTESIAN_POINT('Ctrl Pts',(-5.7299307791557,-120.06175111262,-9.92453123330913));
#29314=CARTESIAN_POINT('Ctrl Pts',(-8.59489616871569,-119.88675111262,-4.96226561664425));
#29315=CARTESIAN_POINT('Ctrl Pts',(-11.4598615582757,-119.71175111262,2.06368086793017E-11));
#29316=CARTESIAN_POINT('Ctrl Pts',(-8.59489616869782,-119.53675111262,4.9622656166752));
#29317=CARTESIAN_POINT('Ctrl Pts',(-5.72993077911996,-119.36175111262,9.92453123332977));
#29318=CARTESIAN_POINT('Ctrl Pts',(1.7871392867044E-11,-119.18675111262,
9.92453123331945));
#29319=CARTESIAN_POINT('Ctrl Pts',(5.7299307791557,-119.01175111262,9.92453123330913));
#29320=CARTESIAN_POINT('Ctrl Pts',(8.59489616871569,-118.83675111262,4.96226561664425));
#29321=CARTESIAN_POINT('Ctrl Pts',(11.4598615582757,-118.66175111262,-2.06354052510241E-11));
#29322=CARTESIAN_POINT('Ctrl Pts',(8.59489616869782,-118.48675111262,-4.9622656166752));
#29323=CARTESIAN_POINT('Ctrl Pts',(5.72993077911996,-118.31175111262,-9.92453123332976));
#29324=CARTESIAN_POINT('Ctrl Pts',(-1.78726082715848E-11,-118.13675111262,
-9.92453123331945));
#29325=CARTESIAN_POINT('Ctrl Pts',(-5.7299307791557,-117.96175111262,-9.92453123330913));
#29326=CARTESIAN_POINT('Ctrl Pts',(-8.59489616871569,-117.78675111262,-4.96226561664425));
#29327=CARTESIAN_POINT('Ctrl Pts',(-11.4598615582757,-117.61175111262,2.06368086793017E-11));
#29328=CARTESIAN_POINT('Ctrl Pts',(-8.59489616869782,-117.43675111262,4.9622656166752));
#29329=CARTESIAN_POINT('Ctrl Pts',(-5.72993077911996,-117.26175111262,9.92453123332977));
#29330=CARTESIAN_POINT('Ctrl Pts',(1.7871392867044E-11,-117.08675111262,
9.92453123331945));
#29331=CARTESIAN_POINT('Ctrl Pts',(5.7299307791557,-116.91175111262,9.92453123330913));
#29332=CARTESIAN_POINT('Ctrl Pts',(8.59489616871569,-116.73675111262,4.96226561664425));
#29333=CARTESIAN_POINT('Ctrl Pts',(11.4598615582757,-116.56175111262,-2.06354052510241E-11));
#29334=CARTESIAN_POINT('Ctrl Pts',(8.59489616869782,-116.38675111262,-4.9622656166752));
#29335=CARTESIAN_POINT('Ctrl Pts',(5.72993077911996,-116.21175111262,-9.92453123332976));
#29336=CARTESIAN_POINT('Ctrl Pts',(-1.78726082715848E-11,-116.03675111262,
-9.92453123331945));
#29337=CARTESIAN_POINT('Ctrl Pts',(-5.7299307791557,-115.86175111262,-9.92453123330913));
#29338=CARTESIAN_POINT('Ctrl Pts',(-8.59489616871569,-115.68675111262,-4.96226561664425));
#29339=CARTESIAN_POINT('Ctrl Pts',(-11.4598615582757,-115.51175111262,2.06368086793017E-11));
#29340=CARTESIAN_POINT('Ctrl Pts',(-8.59489616869782,-115.33675111262,4.9622656166752));
#29341=CARTESIAN_POINT('Ctrl Pts',(-5.72993077911996,-115.16175111262,9.92453123332977));
#29342=CARTESIAN_POINT('Ctrl Pts',(1.7871392867044E-11,-114.98675111262,
9.92453123331945));
#29343=CARTESIAN_POINT('Ctrl Pts',(5.7299307791557,-114.81175111262,9.92453123330913));
#29344=CARTESIAN_POINT('Ctrl Pts',(8.59489616871569,-114.63675111262,4.96226561664425));
#29345=CARTESIAN_POINT('Ctrl Pts',(11.4598615582757,-114.46175111262,-2.06354052510241E-11));
#29346=CARTESIAN_POINT('Ctrl Pts',(8.59489616869782,-114.28675111262,-4.9622656166752));
#29347=CARTESIAN_POINT('Ctrl Pts',(5.72993077911996,-114.11175111262,-9.92453123332976));
#29348=CARTESIAN_POINT('Ctrl Pts',(-1.78726082715848E-11,-113.93675111262,
-9.92453123331945));
#29349=CARTESIAN_POINT('Ctrl Pts',(-5.7299307791557,-113.76175111262,-9.92453123330913));
#29350=CARTESIAN_POINT('Ctrl Pts',(-8.59489616871569,-113.58675111262,-4.96226561664425));
#29351=CARTESIAN_POINT('Ctrl Pts',(-11.4598615582757,-113.41175111262,2.06368086793017E-11));
#29352=CARTESIAN_POINT('Ctrl Pts',(-8.59489616869782,-113.23675111262,4.9622656166752));
#29353=CARTESIAN_POINT('Ctrl Pts',(-5.72993077911996,-113.06175111262,9.92453123332977));
#29354=CARTESIAN_POINT('Ctrl Pts',(1.7871392867044E-11,-112.88675111262,
9.92453123331945));
#29355=CARTESIAN_POINT('Ctrl Pts',(5.7299307791557,-112.71175111262,9.92453123330913));
#29356=CARTESIAN_POINT('Ctrl Pts',(8.59489616871569,-112.53675111262,4.96226561664425));
#29357=CARTESIAN_POINT('Ctrl Pts',(11.4598615582757,-112.36175111262,-2.06354052510241E-11));
#29358=CARTESIAN_POINT('Ctrl Pts',(8.59489616869782,-112.18675111262,-4.9622656166752));
#29359=CARTESIAN_POINT('Ctrl Pts',(5.72993077911996,-112.01175111262,-9.92453123332976));
#29360=CARTESIAN_POINT('Ctrl Pts',(-1.78726082715848E-11,-111.83675111262,
-9.92453123331945));
#29361=CARTESIAN_POINT('Ctrl Pts',(-5.7299307791557,-111.66175111262,-9.92453123330913));
#29362=CARTESIAN_POINT('Ctrl Pts',(-8.59489616871569,-111.48675111262,-4.96226561664425));
#29363=CARTESIAN_POINT('Ctrl Pts',(-11.4598615582757,-111.31175111262,2.06368086793017E-11));
#29364=CARTESIAN_POINT('Ctrl Pts',(-8.59489616869782,-111.13675111262,4.9622656166752));
#29365=CARTESIAN_POINT('Ctrl Pts',(-5.72993077911996,-110.96175111262,9.92453123332977));
#29366=CARTESIAN_POINT('Ctrl Pts',(1.7871392867044E-11,-110.78675111262,
9.92453123331945));
#29367=CARTESIAN_POINT('Ctrl Pts',(5.7299307791557,-110.61175111262,9.92453123330913));
#29368=CARTESIAN_POINT('Ctrl Pts',(8.59489616871569,-110.43675111262,4.96226561664425));
#29369=CARTESIAN_POINT('Ctrl Pts',(11.4598615582757,-110.26175111262,-2.06354052510241E-11));
#29370=CARTESIAN_POINT('Ctrl Pts',(8.59489616869782,-110.08675111262,-4.9622656166752));
#29371=CARTESIAN_POINT('Ctrl Pts',(5.72993077911996,-109.91175111262,-9.92453123332976));
#29372=CARTESIAN_POINT('Ctrl Pts',(-1.78726082715848E-11,-109.73675111262,
-9.92453123331945));
#29373=CARTESIAN_POINT('Ctrl Pts',(-5.7299307791557,-109.56175111262,-9.92453123330913));
#29374=CARTESIAN_POINT('Ctrl Pts',(-8.59489616871569,-109.38675111262,-4.96226561664425));
#29375=CARTESIAN_POINT('Ctrl Pts',(-11.4598615582757,-109.21175111262,2.06368086793017E-11));
#29376=CARTESIAN_POINT('Ctrl Pts',(-8.59489616869782,-109.03675111262,4.9622656166752));
#29377=CARTESIAN_POINT('Ctrl Pts',(-5.72993077911996,-108.86175111262,9.92453123332977));
#29378=CARTESIAN_POINT('Ctrl Pts',(1.7871392867044E-11,-108.68675111262,
9.92453123331945));
#29379=CARTESIAN_POINT('Ctrl Pts',(5.7299307791557,-108.51175111262,9.92453123330913));
#29380=CARTESIAN_POINT('Ctrl Pts',(8.59489616871569,-108.33675111262,4.96226561664425));
#29381=CARTESIAN_POINT('Ctrl Pts',(11.4598615582757,-108.16175111262,-2.06354052510241E-11));
#29382=CARTESIAN_POINT('Ctrl Pts',(8.59489616869782,-107.98675111262,-4.9622656166752));
#29383=CARTESIAN_POINT('Ctrl Pts',(5.72993077911996,-107.81175111262,-9.92453123332976));
#29384=CARTESIAN_POINT('Ctrl Pts',(-1.78726082715848E-11,-107.63675111262,
-9.92453123331945));
#29385=CARTESIAN_POINT('Ctrl Pts',(-5.7299307791557,-107.46175111262,-9.92453123330913));
#29386=CARTESIAN_POINT('Ctrl Pts',(-8.59489616871569,-107.28675111262,-4.96226561664425));
#29387=CARTESIAN_POINT('Ctrl Pts',(-11.4598615582757,-107.11175111262,2.06368086793017E-11));
#29388=CARTESIAN_POINT('Ctrl Pts',(-8.59489616869782,-106.93675111262,4.9622656166752));
#29389=CARTESIAN_POINT('Ctrl Pts',(-5.72993077911996,-106.76175111262,9.92453123332977));
#29390=CARTESIAN_POINT('Ctrl Pts',(1.7871392867044E-11,-106.58675111262,
9.92453123331945));
#29391=CARTESIAN_POINT('Ctrl Pts',(5.7299307791557,-106.41175111262,9.92453123330913));
#29392=CARTESIAN_POINT('Ctrl Pts',(8.59489616871569,-106.23675111262,4.96226561664425));
#29393=CARTESIAN_POINT('Ctrl Pts',(11.4598615582757,-106.06175111262,-2.06354052510241E-11));
#29394=CARTESIAN_POINT('Ctrl Pts',(8.59489616869782,-105.88675111262,-4.9622656166752));
#29395=CARTESIAN_POINT('Ctrl Pts',(5.72993077911996,-105.71175111262,-9.92453123332976));
#29396=CARTESIAN_POINT('Ctrl Pts',(-1.78726082715848E-11,-105.53675111262,
-9.92453123331945));
#29397=CARTESIAN_POINT('Ctrl Pts',(-5.7299307791557,-105.36175111262,-9.92453123330913));
#29398=CARTESIAN_POINT('Ctrl Pts',(-8.59489616871569,-105.18675111262,-4.96226561664425));
#29399=CARTESIAN_POINT('Ctrl Pts',(-11.4598615582757,-105.01175111262,2.06368086793017E-11));
#29400=CARTESIAN_POINT('Ctrl Pts',(-8.59489616869782,-104.83675111262,4.9622656166752));
#29401=CARTESIAN_POINT('Ctrl Pts',(-5.72993077911996,-104.66175111262,9.92453123332977));
#29402=CARTESIAN_POINT('Ctrl Pts',(1.7871392867044E-11,-104.48675111262,
9.92453123331945));
#29403=CARTESIAN_POINT('Ctrl Pts',(5.7299307791557,-104.31175111262,9.92453123330913));
#29404=CARTESIAN_POINT('Ctrl Pts',(8.59489616871569,-104.13675111262,4.96226561664425));
#29405=CARTESIAN_POINT('Ctrl Pts',(11.4598615582757,-103.96175111262,-2.06354052510241E-11));
#29406=CARTESIAN_POINT('Ctrl Pts',(8.59489616869782,-103.78675111262,-4.9622656166752));
#29407=CARTESIAN_POINT('Ctrl Pts',(5.72993077911996,-103.61175111262,-9.92453123332976));
#29408=CARTESIAN_POINT('Ctrl Pts',(-1.78726082715848E-11,-103.43675111262,
-9.92453123331945));
#29409=CARTESIAN_POINT('Ctrl Pts',(-5.7299307791557,-103.26175111262,-9.92453123330913));
#29410=CARTESIAN_POINT('Ctrl Pts',(-8.59489616871569,-103.08675111262,-4.96226561664425));
#29411=CARTESIAN_POINT('Ctrl Pts',(-11.4598615582757,-102.91175111262,2.06368086793017E-11));
#29412=CARTESIAN_POINT('Ctrl Pts',(-8.59489616869782,-102.73675111262,4.9622656166752));
#29413=CARTESIAN_POINT('Ctrl Pts',(-5.72993077911996,-102.56175111262,9.92453123332977));
#29414=CARTESIAN_POINT('Ctrl Pts',(1.7871392867044E-11,-102.38675111262,
9.92453123331945));
#29415=CARTESIAN_POINT('Ctrl Pts',(5.7299307791557,-102.21175111262,9.92453123330913));
#29416=CARTESIAN_POINT('Ctrl Pts',(8.59489616871569,-102.03675111262,4.96226561664425));
#29417=CARTESIAN_POINT('Ctrl Pts',(11.4598615582757,-101.86175111262,-2.06354052510241E-11));
#29418=CARTESIAN_POINT('Ctrl Pts',(8.59489616869782,-101.68675111262,-4.9622656166752));
#29419=CARTESIAN_POINT('Ctrl Pts',(5.72993077911996,-101.51175111262,-9.92453123332976));
#29420=CARTESIAN_POINT('Ctrl Pts',(-1.78726082715848E-11,-101.33675111262,
-9.92453123331945));
#29421=CARTESIAN_POINT('Ctrl Pts',(-5.7299307791557,-101.16175111262,-9.92453123330913));
#29422=CARTESIAN_POINT('Ctrl Pts',(-8.59489616871569,-100.98675111262,-4.96226561664425));
#29423=CARTESIAN_POINT('Ctrl Pts',(-11.4598615582757,-100.81175111262,2.06368086793017E-11));
#29424=CARTESIAN_POINT('Ctrl Pts',(-8.59489616869782,-100.63675111262,4.9622656166752));
#29425=CARTESIAN_POINT('Ctrl Pts',(-5.72993077911996,-100.46175111262,9.92453123332977));
#29426=CARTESIAN_POINT('Ctrl Pts',(1.7871392867044E-11,-100.28675111262,
9.92453123331945));
#29427=CARTESIAN_POINT('Ctrl Pts',(5.7299307791557,-100.11175111262,9.92453123330913));
#29428=CARTESIAN_POINT('Ctrl Pts',(8.59489616871569,-99.9367511126202,4.96226561664425));
#29429=CARTESIAN_POINT('Ctrl Pts',(11.4598615582757,-99.7617511126202,-2.06354052510241E-11));
#29430=CARTESIAN_POINT('Ctrl Pts',(8.59489616869782,-99.5867511126202,-4.9622656166752));
#29431=CARTESIAN_POINT('Ctrl Pts',(5.72993077911996,-99.4117511126202,-9.92453123332976));
#29432=CARTESIAN_POINT('Ctrl Pts',(-1.78726082715848E-11,-99.2367511126202,
-9.92453123331945));
#29433=CARTESIAN_POINT('Ctrl Pts',(-5.7299307791557,-99.0617511126202,-9.92453123330913));
#29434=CARTESIAN_POINT('Ctrl Pts',(-8.59489616871569,-98.8867511126202,
-4.96226561664425));
#29435=CARTESIAN_POINT('Ctrl Pts',(-11.4598615582757,-98.7117511126202,
2.06368086793017E-11));
#29436=CARTESIAN_POINT('Ctrl Pts',(-8.59489616869782,-98.5367511126202,
4.9622656166752));
#29437=CARTESIAN_POINT('Ctrl Pts',(-5.72993077911996,-98.3617511126202,
9.92453123332977));
#29438=CARTESIAN_POINT('Ctrl Pts',(1.7871392867044E-11,-98.1867511126202,
9.92453123331945));
#29439=CARTESIAN_POINT('Ctrl Pts',(5.7299307791557,-98.0117511126202,9.92453123330913));
#29440=CARTESIAN_POINT('Ctrl Pts',(8.59489616871569,-97.8367511126202,4.96226561664425));
#29441=CARTESIAN_POINT('Ctrl Pts',(11.4598615582757,-97.6617511126202,-2.06354052510241E-11));
#29442=CARTESIAN_POINT('Ctrl Pts',(8.59489616869782,-97.4867511126202,-4.9622656166752));
#29443=CARTESIAN_POINT('Ctrl Pts',(5.72993077911996,-97.3117511126202,-9.92453123332976));
#29444=CARTESIAN_POINT('Ctrl Pts',(-1.78726082715848E-11,-97.1367511126202,
-9.92453123331945));
#29445=CARTESIAN_POINT('Ctrl Pts',(-5.7299307791557,-96.9617511126202,-9.92453123330913));
#29446=CARTESIAN_POINT('Ctrl Pts',(-8.59489616871569,-96.7867511126202,
-4.96226561664425));
#29447=CARTESIAN_POINT('Ctrl Pts',(-11.4598615582757,-96.6117511126202,
2.06368086793017E-11));
#29448=CARTESIAN_POINT('Ctrl Pts',(-8.59489616869782,-96.4367511126202,
4.9622656166752));
#29449=CARTESIAN_POINT('Ctrl Pts',(-5.72993077911996,-96.2617511126202,
9.92453123332977));
#29450=CARTESIAN_POINT('Ctrl Pts',(1.7871392867044E-11,-96.0867511126202,
9.92453123331945));
#29451=CARTESIAN_POINT('Ctrl Pts',(5.7299307791557,-95.9117511126202,9.92453123330913));
#29452=CARTESIAN_POINT('Ctrl Pts',(8.59489616871569,-95.7367511126202,4.96226561664425));
#29453=CARTESIAN_POINT('Ctrl Pts',(11.4598615582757,-95.5617511126202,-2.06354052510241E-11));
#29454=CARTESIAN_POINT('Ctrl Pts',(8.59489616869782,-95.3867511126202,-4.9622656166752));
#29455=CARTESIAN_POINT('Ctrl Pts',(5.72993077911996,-95.2117511126202,-9.92453123332976));
#29456=CARTESIAN_POINT('Ctrl Pts',(-1.78726082715848E-11,-95.0367511126202,
-9.92453123331945));
#29457=CARTESIAN_POINT('Ctrl Pts',(-5.7299307791557,-94.8617511126203,-9.92453123330913));
#29458=CARTESIAN_POINT('Ctrl Pts',(-8.59489616871569,-94.6867511126202,
-4.96226561664425));
#29459=CARTESIAN_POINT('Ctrl Pts',(-11.4598615582757,-94.5117511126202,
2.06368086793017E-11));
#29460=CARTESIAN_POINT('Ctrl Pts',(-8.59489616869782,-94.3367511126202,
4.9622656166752));
#29461=CARTESIAN_POINT('Ctrl Pts',(-5.72993077911996,-94.1617511126202,
9.92453123332977));
#29462=CARTESIAN_POINT('Ctrl Pts',(1.7871392867044E-11,-93.9867511126202,
9.92453123331945));
#29463=CARTESIAN_POINT('Ctrl Pts',(5.7299307791557,-93.8117511126202,9.92453123330913));
#29464=CARTESIAN_POINT('Ctrl Pts',(8.59489616871569,-93.6367511126202,4.96226561664425));
#29465=CARTESIAN_POINT('Ctrl Pts',(11.4598615582757,-93.4617511126202,-2.06354052510241E-11));
#29466=CARTESIAN_POINT('Ctrl Pts',(8.59489616869782,-93.2867511126202,-4.9622656166752));
#29467=CARTESIAN_POINT('Ctrl Pts',(5.72993077911996,-93.1117511126202,-9.92453123332976));
#29468=CARTESIAN_POINT('Ctrl Pts',(-1.78726082715848E-11,-92.9367511126202,
-9.92453123331945));
#29469=CARTESIAN_POINT('Ctrl Pts',(-5.7299307791557,-92.7617511126202,-9.92453123330913));
#29470=CARTESIAN_POINT('Ctrl Pts',(-8.59489616871569,-92.5867511126202,
-4.96226561664425));
#29471=CARTESIAN_POINT('Ctrl Pts',(-11.4598615582757,-92.4117511126202,
2.06368086793017E-11));
#29472=CARTESIAN_POINT('Ctrl Pts',(-8.59489616869782,-92.2367511126202,
4.9622656166752));
#29473=CARTESIAN_POINT('Ctrl Pts',(-5.72993077911996,-92.0617511126202,
9.92453123332977));
#29474=CARTESIAN_POINT('Ctrl Pts',(1.7871392867044E-11,-91.8867511126202,
9.92453123331945));
#29475=CARTESIAN_POINT('Ctrl Pts',(5.7299307791557,-91.7117511126202,9.92453123330913));
#29476=CARTESIAN_POINT('Ctrl Pts',(8.59489616871569,-91.5367511126202,4.96226561664425));
#29477=CARTESIAN_POINT('Ctrl Pts',(11.4598615582757,-91.3617511126203,-2.06354052510241E-11));
#29478=CARTESIAN_POINT('Ctrl Pts',(8.59489616869782,-91.1867511126202,-4.9622656166752));
#29479=CARTESIAN_POINT('Ctrl Pts',(5.72993077911996,-91.0117511126202,-9.92453123332976));
#29480=CARTESIAN_POINT('Ctrl Pts',(-1.78726082715848E-11,-90.8367511126202,
-9.92453123331945));
#29481=CARTESIAN_POINT('Ctrl Pts',(-5.7299307791557,-90.6617511126203,-9.92453123330913));
#29482=CARTESIAN_POINT('Ctrl Pts',(-8.59489616871569,-90.4867511126203,
-4.96226561664425));
#29483=CARTESIAN_POINT('Ctrl Pts',(-11.4598615582757,-90.3117511126202,
2.06368086793017E-11));
#29484=CARTESIAN_POINT('Ctrl Pts',(-8.59489616869782,-90.1367511126202,
4.9622656166752));
#29485=CARTESIAN_POINT('Ctrl Pts',(-5.72993077911996,-89.9617511126202,
9.92453123332977));
#29486=CARTESIAN_POINT('Ctrl Pts',(1.7871392867044E-11,-89.7867511126202,
9.92453123331945));
#29487=CARTESIAN_POINT('Ctrl Pts',(5.7299307791557,-89.6117511126202,9.92453123330913));
#29488=CARTESIAN_POINT('Ctrl Pts',(8.59489616871569,-89.4367511126202,4.96226561664425));
#29489=CARTESIAN_POINT('Ctrl Pts',(11.4598615582757,-89.2617511126202,-2.06354052510241E-11));
#29490=CARTESIAN_POINT('Ctrl Pts',(8.59489616869782,-89.0867511126202,-4.9622656166752));
#29491=CARTESIAN_POINT('Ctrl Pts',(5.72993077911996,-88.9117511126202,-9.92453123332976));
#29492=CARTESIAN_POINT('Ctrl Pts',(-1.78726082715848E-11,-88.7367511126203,
-9.92453123331945));
#29493=CARTESIAN_POINT('Ctrl Pts',(-5.7299307791557,-88.5617511126202,-9.92453123330913));
#29494=CARTESIAN_POINT('Ctrl Pts',(-8.59489616871569,-88.3867511126202,
-4.96226561664425));
#29495=CARTESIAN_POINT('Ctrl Pts',(-11.4598615582757,-88.2117511126203,
2.06368086793017E-11));
#29496=CARTESIAN_POINT('Ctrl Pts',(-8.59489616869782,-88.0367511126202,
4.9622656166752));
#29497=CARTESIAN_POINT('Ctrl Pts',(-5.72993077911996,-87.8617511126202,
9.92453123332977));
#29498=CARTESIAN_POINT('Ctrl Pts',(1.7871392867044E-11,-87.6867511126203,
9.92453123331945));
#29499=CARTESIAN_POINT('Ctrl Pts',(5.7299307791557,-87.5117511126203,9.92453123330913));
#29500=CARTESIAN_POINT('Ctrl Pts',(8.59489616871569,-87.3367511126202,4.96226561664425));
#29501=CARTESIAN_POINT('Ctrl Pts',(11.4598615582757,-87.1617511126203,-2.06354052510241E-11));
#29502=CARTESIAN_POINT('Ctrl Pts',(8.59489616869782,-86.9867511126203,-4.9622656166752));
#29503=CARTESIAN_POINT('Ctrl Pts',(5.72993077911996,-86.8117511126202,-9.92453123332976));
#29504=CARTESIAN_POINT('Ctrl Pts',(-1.78726082715848E-11,-86.6367511126202,
-9.92453123331945));
#29505=CARTESIAN_POINT('Ctrl Pts',(-5.7299307791557,-86.4617511126202,-9.92453123330913));
#29506=CARTESIAN_POINT('Ctrl Pts',(-8.59489616871569,-86.2867511126203,
-4.96226561664425));
#29507=CARTESIAN_POINT('Ctrl Pts',(-11.4598615582757,-86.1117511126202,
2.06368086793017E-11));
#29508=CARTESIAN_POINT('Ctrl Pts',(-8.59489616869782,-85.9367511126203,
4.9622656166752));
#29509=CARTESIAN_POINT('Ctrl Pts',(-5.72993077911996,-85.7617511126202,
9.92453123332977));
#29510=CARTESIAN_POINT('Ctrl Pts',(1.7871392867044E-11,-85.5867511126202,
9.92453123331945));
#29511=CARTESIAN_POINT('Ctrl Pts',(5.7299307791557,-85.4117511126203,9.92453123330913));
#29512=CARTESIAN_POINT('Ctrl Pts',(8.59489616871569,-85.2367511126202,4.96226561664425));
#29513=CARTESIAN_POINT('Ctrl Pts',(11.4598615582757,-85.0617511126202,-2.06354052510241E-11));
#29514=CARTESIAN_POINT('Ctrl Pts',(8.59489616869782,-84.8867511126203,-4.9622656166752));
#29515=CARTESIAN_POINT('Ctrl Pts',(5.72993077911996,-84.7117511126202,-9.92453123332976));
#29516=CARTESIAN_POINT('Ctrl Pts',(-1.78726082715848E-11,-84.5367511126202,
-9.92453123331945));
#29517=CARTESIAN_POINT('Ctrl Pts',(-5.7299307791557,-84.3617511126203,-9.92453123330913));
#29518=CARTESIAN_POINT('Ctrl Pts',(-8.59489616871569,-84.1867511126203,
-4.96226561664425));
#29519=CARTESIAN_POINT('Ctrl Pts',(-11.4598615582757,-84.0117511126203,
2.06368086793017E-11));
#29520=CARTESIAN_POINT('Ctrl Pts',(-8.59489616869782,-83.8367511126203,
4.9622656166752));
#29521=CARTESIAN_POINT('Ctrl Pts',(-5.72993077911996,-83.6617511126203,
9.92453123332977));
#29522=CARTESIAN_POINT('Ctrl Pts',(1.7871392867044E-11,-83.4867511126202,
9.92453123331945));
#29523=CARTESIAN_POINT('Ctrl Pts',(5.7299307791557,-83.3117511126203,9.92453123330913));
#29524=CARTESIAN_POINT('Ctrl Pts',(8.59489616871569,-83.1367511126203,4.96226561664425));
#29525=CARTESIAN_POINT('Ctrl Pts',(11.4598615582757,-82.9617511126203,-2.06354052510241E-11));
#29526=CARTESIAN_POINT('Ctrl Pts',(8.59489616869782,-82.7867511126203,-4.9622656166752));
#29527=CARTESIAN_POINT('Ctrl Pts',(5.72993077911996,-82.6117511126203,-9.92453123332976));
#29528=CARTESIAN_POINT('Ctrl Pts',(-1.78726082715848E-11,-82.4367511126202,
-9.92453123331945));
#29529=CARTESIAN_POINT('Ctrl Pts',(-5.7299307791557,-82.2617511126202,-9.92453123330913));
#29530=CARTESIAN_POINT('Ctrl Pts',(-8.59489616871569,-82.0867511126203,
-4.96226561664425));
#29531=CARTESIAN_POINT('Ctrl Pts',(-11.4598615582757,-81.9117511126203,
2.06368086793017E-11));
#29532=CARTESIAN_POINT('Ctrl Pts',(-8.59489616869782,-81.7367511126203,
4.9622656166752));
#29533=CARTESIAN_POINT('Ctrl Pts',(-5.72993077911996,-81.5617511126202,
9.92453123332977));
#29534=CARTESIAN_POINT('Ctrl Pts',(1.7871392867044E-11,-81.3867511126203,
9.92453123331945));
#29535=CARTESIAN_POINT('Ctrl Pts',(5.7299307791557,-81.2117511126202,9.92453123330913));
#29536=CARTESIAN_POINT('Ctrl Pts',(8.59489616871569,-81.0367511126203,4.96226561664425));
#29537=CARTESIAN_POINT('Ctrl Pts',(11.4598615582757,-80.8617511126203,-2.06354052510241E-11));
#29538=CARTESIAN_POINT('Ctrl Pts',(8.59489616869782,-80.6867511126202,-4.9622656166752));
#29539=CARTESIAN_POINT('Ctrl Pts',(5.72993077911996,-80.5117511126203,-9.92453123332976));
#29540=CARTESIAN_POINT('Ctrl Pts',(-1.78726082715848E-11,-80.3367511126203,
-9.92453123331945));
#29541=CARTESIAN_POINT('Ctrl Pts',(-5.7299307791557,-80.1617511126202,-9.92453123330913));
#29542=CARTESIAN_POINT('Ctrl Pts',(-8.59489616871569,-79.9867511126203,
-4.96226561664425));
#29543=CARTESIAN_POINT('Ctrl Pts',(-11.4598615582757,-79.8117511126203,
2.06368086793017E-11));
#29544=CARTESIAN_POINT('Ctrl Pts',(-8.59489616869782,-79.6367511126202,
4.9622656166752));
#29545=CARTESIAN_POINT('Ctrl Pts',(-5.72993077911996,-79.4617511126203,
9.92453123332977));
#29546=CARTESIAN_POINT('Ctrl Pts',(1.7871392867044E-11,-79.2867511126203,
9.92453123331945));
#29547=CARTESIAN_POINT('Ctrl Pts',(5.7299307791557,-79.1117511126203,9.92453123330913));
#29548=CARTESIAN_POINT('Ctrl Pts',(8.59489616871569,-78.9367511126203,4.96226561664425));
#29549=CARTESIAN_POINT('Ctrl Pts',(11.4598615582757,-78.7617511126203,-2.06354052510241E-11));
#29550=CARTESIAN_POINT('Ctrl Pts',(8.59489616869782,-78.5867511126203,-4.9622656166752));
#29551=CARTESIAN_POINT('Ctrl Pts',(5.72993077911996,-78.4117511126203,-9.92453123332976));
#29552=CARTESIAN_POINT('Ctrl Pts',(-1.78726082715848E-11,-78.2367511126203,
-9.92453123331945));
#29553=CARTESIAN_POINT('Ctrl Pts',(-5.7299307791557,-78.0617511126203,-9.92453123330913));
#29554=CARTESIAN_POINT('Ctrl Pts',(-8.59489616871569,-77.8867511126202,
-4.96226561664425));
#29555=CARTESIAN_POINT('Ctrl Pts',(-11.4598615582757,-77.7117511126203,
2.06368086793017E-11));
#29556=CARTESIAN_POINT('Ctrl Pts',(-8.59489616869782,-77.5367511126203,
4.9622656166752));
#29557=CARTESIAN_POINT('Ctrl Pts',(-5.72993077911996,-77.3617511126203,
9.92453123332977));
#29558=CARTESIAN_POINT('Ctrl Pts',(1.7871392867044E-11,-77.1867511126203,
9.92453123331945));
#29559=CARTESIAN_POINT('Ctrl Pts',(5.7299307791557,-77.0117511126203,9.92453123330913));
#29560=CARTESIAN_POINT('Ctrl Pts',(8.59489616871569,-76.8367511126202,4.96226561664425));
#29561=CARTESIAN_POINT('Ctrl Pts',(11.4598615582757,-76.6617511126203,-2.06354052510241E-11));
#29562=CARTESIAN_POINT('Ctrl Pts',(8.59489616869782,-76.4867511126203,-4.9622656166752));
#29563=CARTESIAN_POINT('Ctrl Pts',(5.72993077911996,-76.3117511126203,-9.92453123332976));
#29564=CARTESIAN_POINT('Ctrl Pts',(-1.78726082715848E-11,-76.1367511126203,
-9.92453123331945));
#29565=CARTESIAN_POINT('Ctrl Pts',(-5.7299307791557,-75.9617511126203,-9.92453123330913));
#29566=CARTESIAN_POINT('Ctrl Pts',(-8.59489616871569,-75.7867511126203,
-4.96226561664425));
#29567=CARTESIAN_POINT('Ctrl Pts',(-11.4598615582757,-75.6117511126203,
2.06368086793017E-11));
#29568=CARTESIAN_POINT('Ctrl Pts',(-8.59489616869782,-75.4367511126203,
4.9622656166752));
#29569=CARTESIAN_POINT('Ctrl Pts',(-5.72993077911996,-75.2617511126203,
9.92453123332977));
#29570=CARTESIAN_POINT('Ctrl Pts',(1.7871392867044E-11,-75.0867511126203,
9.92453123331945));
#29571=CARTESIAN_POINT('Ctrl Pts',(5.7299307791557,-74.9117511126203,9.92453123330913));
#29572=CARTESIAN_POINT('Ctrl Pts',(8.59489616871569,-74.7367511126203,4.96226561664425));
#29573=CARTESIAN_POINT('Ctrl Pts',(11.4598615582757,-74.5617511126203,-2.06354052510241E-11));
#29574=CARTESIAN_POINT('Ctrl Pts',(8.59489616869782,-74.3867511126203,-4.9622656166752));
#29575=CARTESIAN_POINT('Ctrl Pts',(5.72993077911996,-74.2117511126203,-9.92453123332976));
#29576=CARTESIAN_POINT('Ctrl Pts',(-1.78726082715848E-11,-74.0367511126203,
-9.92453123331945));
#29577=CARTESIAN_POINT('Ctrl Pts',(-5.7299307791557,-73.8617511126203,-9.92453123330913));
#29578=CARTESIAN_POINT('Ctrl Pts',(-8.59489616871569,-73.6867511126203,
-4.96226561664425));
#29579=CARTESIAN_POINT('Ctrl Pts',(-11.4598615582757,-73.5117511126203,
2.06368086793017E-11));
#29580=CARTESIAN_POINT('Ctrl Pts',(-8.59489616869782,-73.3367511126203,
4.9622656166752));
#29581=CARTESIAN_POINT('Ctrl Pts',(-5.72993077911996,-73.1617511126203,
9.92453123332977));
#29582=CARTESIAN_POINT('Ctrl Pts',(1.7871392867044E-11,-72.9867511126203,
9.92453123331945));
#29583=CARTESIAN_POINT('Ctrl Pts',(5.7299307791557,-72.8117511126203,9.92453123330913));
#29584=CARTESIAN_POINT('Ctrl Pts',(8.59489616871569,-72.6367511126203,4.96226561664425));
#29585=CARTESIAN_POINT('Ctrl Pts',(11.4598615582757,-72.4617511126203,-2.06354052510241E-11));
#29586=CARTESIAN_POINT('Ctrl Pts',(8.59489616869782,-72.2867511126203,-4.9622656166752));
#29587=CARTESIAN_POINT('Ctrl Pts',(5.72993077911996,-72.1117511126203,-9.92453123332976));
#29588=CARTESIAN_POINT('Ctrl Pts',(-1.78726082715848E-11,-71.9367511126203,
-9.92453123331945));
#29589=CARTESIAN_POINT('Ctrl Pts',(-5.7299307791557,-71.7617511126203,-9.92453123330913));
#29590=CARTESIAN_POINT('Ctrl Pts',(-8.59489616871569,-71.5867511126203,
-4.96226561664425));
#29591=CARTESIAN_POINT('Ctrl Pts',(-11.4598615582757,-71.4117511126203,
2.06368086793017E-11));
#29592=CARTESIAN_POINT('Ctrl Pts',(-8.59489616869782,-71.2367511126203,
4.9622656166752));
#29593=CARTESIAN_POINT('Ctrl Pts',(-5.72993077911996,-71.0617511126203,
9.92453123332977));
#29594=CARTESIAN_POINT('Ctrl Pts',(1.7871392867044E-11,-70.8867511126203,
9.92453123331945));
#29595=CARTESIAN_POINT('Ctrl Pts',(5.7299307791557,-70.7117511126203,9.92453123330913));
#29596=CARTESIAN_POINT('Ctrl Pts',(8.59489616871569,-70.5367511126203,4.96226561664425));
#29597=CARTESIAN_POINT('Ctrl Pts',(11.4598615582757,-70.3617511126203,-2.06354052510241E-11));
#29598=CARTESIAN_POINT('Ctrl Pts',(8.59489616869782,-70.1867511126203,-4.9622656166752));
#29599=CARTESIAN_POINT('Ctrl Pts',(5.72993077911996,-70.0117511126203,-9.92453123332976));
#29600=CARTESIAN_POINT('Ctrl Pts',(-1.78726082715848E-11,-69.8367511126203,
-9.92453123331945));
#29601=CARTESIAN_POINT('Ctrl Pts',(-5.7299307791557,-69.6617511126203,-9.92453123330913));
#29602=CARTESIAN_POINT('Ctrl Pts',(-8.59489616871569,-69.4867511126203,
-4.96226561664425));
#29603=CARTESIAN_POINT('Ctrl Pts',(-11.4598615582757,-69.3117511126203,
2.06368086793017E-11));
#29604=CARTESIAN_POINT('Ctrl Pts',(-8.59489616869782,-69.1367511126203,
4.9622656166752));
#29605=CARTESIAN_POINT('Ctrl Pts',(-5.72993077911996,-68.9617511126203,
9.92453123332977));
#29606=CARTESIAN_POINT('Ctrl Pts',(1.7871392867044E-11,-68.7867511126203,
9.92453123331945));
#29607=CARTESIAN_POINT('Ctrl Pts',(5.7299307791557,-68.6117511126203,9.92453123330913));
#29608=CARTESIAN_POINT('Ctrl Pts',(8.59489616871569,-68.4367511126203,4.96226561664425));
#29609=CARTESIAN_POINT('Ctrl Pts',(11.4598615582757,-68.2617511126203,-2.06354052510241E-11));
#29610=CARTESIAN_POINT('Ctrl Pts',(8.59489616869782,-68.0867511126203,-4.9622656166752));
#29611=CARTESIAN_POINT('Ctrl Pts',(5.72993077911996,-67.9117511126203,-9.92453123332976));
#29612=CARTESIAN_POINT('Ctrl Pts',(-1.78726082715848E-11,-67.7367511126203,
-9.92453123331945));
#29613=CARTESIAN_POINT('Ctrl Pts',(-5.7299307791557,-67.5617511126203,-9.92453123330913));
#29614=CARTESIAN_POINT('Ctrl Pts',(-8.59489616871569,-67.3867511126203,
-4.96226561664425));
#29615=CARTESIAN_POINT('Ctrl Pts',(-11.4598615582757,-67.2117511126203,
2.06368086793017E-11));
#29616=CARTESIAN_POINT('Ctrl Pts',(-8.59489616869782,-67.0367511126203,
4.9622656166752));
#29617=CARTESIAN_POINT('Ctrl Pts',(-5.72993077911996,-66.8617511126203,
9.92453123332977));
#29618=CARTESIAN_POINT('Ctrl Pts',(1.7871392867044E-11,-66.6867511126203,
9.92453123331945));
#29619=CARTESIAN_POINT('Ctrl Pts',(5.7299307791557,-66.5117511126203,9.92453123330913));
#29620=CARTESIAN_POINT('Ctrl Pts',(8.59489616871569,-66.3367511126203,4.96226561664425));
#29621=CARTESIAN_POINT('Ctrl Pts',(11.4598615582757,-66.1617511126203,-2.06354052510241E-11));
#29622=CARTESIAN_POINT('Ctrl Pts',(8.59489616869782,-65.9867511126203,-4.9622656166752));
#29623=CARTESIAN_POINT('Ctrl Pts',(5.72993077911996,-65.8117511126203,-9.92453123332976));
#29624=CARTESIAN_POINT('Ctrl Pts',(-1.78726082715848E-11,-65.6367511126203,
-9.92453123331945));
#29625=CARTESIAN_POINT('Ctrl Pts',(-5.7299307791557,-65.4617511126203,-9.92453123330913));
#29626=CARTESIAN_POINT('Ctrl Pts',(-8.59489616871569,-65.2867511126203,
-4.96226561664425));
#29627=CARTESIAN_POINT('Ctrl Pts',(-11.4598615582757,-65.1117511126203,
2.06368086793017E-11));
#29628=CARTESIAN_POINT('Ctrl Pts',(-8.59489616869782,-64.9367511126203,
4.9622656166752));
#29629=CARTESIAN_POINT('Ctrl Pts',(-5.72993077911996,-64.7617511126203,
9.92453123332977));
#29630=CARTESIAN_POINT('Ctrl Pts',(1.7871392867044E-11,-64.5867511126203,
9.92453123331945));
#29631=CARTESIAN_POINT('Ctrl Pts',(5.7299307791557,-64.4117511126203,9.92453123330913));
#29632=CARTESIAN_POINT('Ctrl Pts',(8.59489616871569,-64.2367511126203,4.96226561664425));
#29633=CARTESIAN_POINT('Ctrl Pts',(11.4598615582757,-64.0617511126203,-2.06354052510241E-11));
#29634=CARTESIAN_POINT('Ctrl Pts',(8.59489616869782,-63.8867511126203,-4.9622656166752));
#29635=CARTESIAN_POINT('Ctrl Pts',(5.72993077911996,-63.7117511126203,-9.92453123332976));
#29636=CARTESIAN_POINT('Ctrl Pts',(-1.78726082715848E-11,-63.5367511126203,
-9.92453123331945));
#29637=CARTESIAN_POINT('Ctrl Pts',(-5.7299307791557,-63.3617511126203,-9.92453123330913));
#29638=CARTESIAN_POINT('Ctrl Pts',(-8.59489616871569,-63.1867511126203,
-4.96226561664425));
#29639=CARTESIAN_POINT('Ctrl Pts',(-11.4598615582757,-63.0117511126203,
2.06368086793017E-11));
#29640=CARTESIAN_POINT('Ctrl Pts',(-8.59489616869782,-62.8367511126203,
4.9622656166752));
#29641=CARTESIAN_POINT('Ctrl Pts',(-5.72993077911996,-62.6617511126203,
9.92453123332977));
#29642=CARTESIAN_POINT('Ctrl Pts',(1.7871392867044E-11,-62.4867511126203,
9.92453123331945));
#29643=CARTESIAN_POINT('Ctrl Pts',(5.7299307791557,-62.3117511126203,9.92453123330913));
#29644=CARTESIAN_POINT('Ctrl Pts',(8.59489616871569,-62.1367511126203,4.96226561664425));
#29645=CARTESIAN_POINT('Ctrl Pts',(11.4598615582757,-61.9617511126203,-2.06354052510241E-11));
#29646=CARTESIAN_POINT('Ctrl Pts',(8.59489616869782,-61.7867511126203,-4.9622656166752));
#29647=CARTESIAN_POINT('Ctrl Pts',(5.72993077911996,-61.6117511126203,-9.92453123332976));
#29648=CARTESIAN_POINT('Ctrl Pts',(-1.78726082715848E-11,-61.4367511126203,
-9.92453123331945));
#29649=CARTESIAN_POINT('Ctrl Pts',(-5.7299307791557,-61.2617511126203,-9.92453123330913));
#29650=CARTESIAN_POINT('Ctrl Pts',(-8.59489616871569,-61.0867511126203,
-4.96226561664425));
#29651=CARTESIAN_POINT('Ctrl Pts',(-11.4598615582757,-60.9117511126203,
2.06368086793017E-11));
#29652=CARTESIAN_POINT('Ctrl Pts',(-8.59489616869782,-60.7367511126203,
4.9622656166752));
#29653=CARTESIAN_POINT('Ctrl Pts',(-5.72993077911996,-60.5617511126203,
9.92453123332977));
#29654=CARTESIAN_POINT('Ctrl Pts',(1.7871392867044E-11,-60.3867511126203,
9.92453123331945));
#29655=CARTESIAN_POINT('Ctrl Pts',(5.7299307791557,-60.2117511126203,9.92453123330913));
#29656=CARTESIAN_POINT('Ctrl Pts',(8.59489616871569,-60.0367511126203,4.96226561664425));
#29657=CARTESIAN_POINT('Ctrl Pts',(11.4598615582757,-59.8617511126203,-2.06354052510241E-11));
#29658=CARTESIAN_POINT('Ctrl Pts',(8.59489616869782,-59.6867511126203,-4.9622656166752));
#29659=CARTESIAN_POINT('Ctrl Pts',(5.72993077911996,-59.5117511126203,-9.92453123332976));
#29660=CARTESIAN_POINT('Ctrl Pts',(-1.78726082715848E-11,-59.3367511126203,
-9.92453123331945));
#29661=CARTESIAN_POINT('Ctrl Pts',(-5.7299307791557,-59.1617511126203,-9.92453123330913));
#29662=CARTESIAN_POINT('Ctrl Pts',(-8.59489616871569,-58.9867511126203,
-4.96226561664425));
#29663=CARTESIAN_POINT('Ctrl Pts',(-11.4598615582757,-58.8117511126203,
2.06368086793017E-11));
#29664=CARTESIAN_POINT('Ctrl Pts',(-8.59489616869782,-58.6367511126203,
4.9622656166752));
#29665=CARTESIAN_POINT('Ctrl Pts',(-5.72993077911996,-58.4617511126203,
9.92453123332977));
#29666=CARTESIAN_POINT('Ctrl Pts',(1.7871392867044E-11,-58.2867511126203,
9.92453123331945));
#29667=CARTESIAN_POINT('Ctrl Pts',(5.7299307791557,-58.1117511126203,9.92453123330913));
#29668=CARTESIAN_POINT('Ctrl Pts',(8.59489616871569,-57.9367511126203,4.96226561664425));
#29669=CARTESIAN_POINT('Ctrl Pts',(11.4598615582757,-57.7617511126203,-2.06354052510241E-11));
#29670=CARTESIAN_POINT('Ctrl Pts',(8.59489616869782,-57.5867511126203,-4.9622656166752));
#29671=CARTESIAN_POINT('Ctrl Pts',(5.72993077911996,-57.4117511126203,-9.92453123332976));
#29672=CARTESIAN_POINT('Ctrl Pts',(-1.78726082715848E-11,-57.2367511126203,
-9.92453123331945));
#29673=CARTESIAN_POINT('Ctrl Pts',(-5.7299307791557,-57.0617511126203,-9.92453123330913));
#29674=CARTESIAN_POINT('Ctrl Pts',(-8.59489616871569,-56.8867511126203,
-4.96226561664425));
#29675=CARTESIAN_POINT('Ctrl Pts',(-11.4598615582757,-56.7117511126203,
2.06368086793017E-11));
#29676=CARTESIAN_POINT('Ctrl Pts',(-8.59489616869782,-56.5367511126203,
4.9622656166752));
#29677=CARTESIAN_POINT('Ctrl Pts',(-5.72993077911996,-56.3617511126203,
9.92453123332977));
#29678=CARTESIAN_POINT('Ctrl Pts',(1.7871392867044E-11,-56.1867511126203,
9.92453123331945));
#29679=CARTESIAN_POINT('Ctrl Pts',(5.7299307791557,-56.0117511126203,9.92453123330913));
#29680=CARTESIAN_POINT('Ctrl Pts',(8.59489616871569,-55.8367511126203,4.96226561664425));
#29681=CARTESIAN_POINT('Ctrl Pts',(11.4598615582757,-55.6617511126203,-2.06354052510241E-11));
#29682=CARTESIAN_POINT('Ctrl Pts',(8.59489616869782,-55.4867511126203,-4.9622656166752));
#29683=CARTESIAN_POINT('Ctrl Pts',(5.72993077911996,-55.3117511126203,-9.92453123332976));
#29684=CARTESIAN_POINT('Ctrl Pts',(-1.78726082715848E-11,-55.1367511126203,
-9.92453123331945));
#29685=CARTESIAN_POINT('Ctrl Pts',(-5.7299307791557,-54.9617511126203,-9.92453123330913));
#29686=CARTESIAN_POINT('Ctrl Pts',(-8.59489616871569,-54.7867511126203,
-4.96226561664425));
#29687=CARTESIAN_POINT('Ctrl Pts',(-11.4598615582757,-54.6117511126203,
2.06368086793017E-11));
#29688=CARTESIAN_POINT('Ctrl Pts',(-8.59489616869782,-54.4367511126203,
4.9622656166752));
#29689=CARTESIAN_POINT('Ctrl Pts',(-5.72993077911996,-54.2617511126203,
9.92453123332977));
#29690=CARTESIAN_POINT('Ctrl Pts',(1.7871392867044E-11,-54.0867511126203,
9.92453123331945));
#29691=CARTESIAN_POINT('Ctrl Pts',(5.7299307791557,-53.9117511126203,9.92453123330913));
#29692=CARTESIAN_POINT('Ctrl Pts',(8.59489616871569,-53.7367511126203,4.96226561664425));
#29693=CARTESIAN_POINT('Ctrl Pts',(11.4598615582757,-53.5617511126203,-2.06354052510241E-11));
#29694=CARTESIAN_POINT('Ctrl Pts',(8.59489616869782,-53.3867511126203,-4.9622656166752));
#29695=CARTESIAN_POINT('Ctrl Pts',(5.72993077911996,-53.2117511126203,-9.92453123332976));
#29696=CARTESIAN_POINT('Ctrl Pts',(-1.78726082715848E-11,-53.0367511126203,
-9.92453123331945));
#29697=CARTESIAN_POINT('Ctrl Pts',(-5.7299307791557,-52.8617511126203,-9.92453123330913));
#29698=CARTESIAN_POINT('Ctrl Pts',(-8.59489616871569,-52.6867511126203,
-4.96226561664425));
#29699=CARTESIAN_POINT('Ctrl Pts',(-11.4598615582757,-52.5117511126203,
2.06368086793017E-11));
#29700=CARTESIAN_POINT('Ctrl Pts',(-8.59489616869782,-52.3367511126203,
4.9622656166752));
#29701=CARTESIAN_POINT('Ctrl Pts',(-5.72993077911996,-52.1617511126203,
9.92453123332977));
#29702=CARTESIAN_POINT('Ctrl Pts',(1.7871392867044E-11,-51.9867511126203,
9.92453123331945));
#29703=CARTESIAN_POINT('Ctrl Pts',(5.7299307791557,-51.8117511126203,9.92453123330913));
#29704=CARTESIAN_POINT('Ctrl Pts',(8.59489616871569,-51.6367511126203,4.96226561664425));
#29705=CARTESIAN_POINT('Ctrl Pts',(11.4598615582757,-51.4617511126203,-2.06354052510241E-11));
#29706=CARTESIAN_POINT('Ctrl Pts',(8.59489616869782,-51.2867511126203,-4.9622656166752));
#29707=CARTESIAN_POINT('Ctrl Pts',(5.72993077911996,-51.1117511126203,-9.92453123332976));
#29708=CARTESIAN_POINT('Ctrl Pts',(-1.78726082715848E-11,-50.9367511126203,
-9.92453123331945));
#29709=CARTESIAN_POINT('Ctrl Pts',(-5.7299307791557,-50.7617511126203,-9.92453123330913));
#29710=CARTESIAN_POINT('Ctrl Pts',(-8.59489616871569,-50.5867511126203,
-4.96226561664425));
#29711=CARTESIAN_POINT('Ctrl Pts',(-11.4598615582757,-50.4117511126203,
2.06368086793017E-11));
#29712=CARTESIAN_POINT('Ctrl Pts',(-8.59489616869782,-50.2367511126203,
4.9622656166752));
#29713=CARTESIAN_POINT('Ctrl Pts',(-5.72993077911996,-50.0617511126203,
9.92453123332977));
#29714=CARTESIAN_POINT('Ctrl Pts',(1.7871392867044E-11,-49.8867511126203,
9.92453123331945));
#29715=CARTESIAN_POINT('Ctrl Pts',(5.7299307791557,-49.7117511126203,9.92453123330913));
#29716=CARTESIAN_POINT('Ctrl Pts',(8.59489616871569,-49.5367511126203,4.96226561664425));
#29717=CARTESIAN_POINT('Ctrl Pts',(11.4598615582757,-49.3617511126203,-2.06354052510241E-11));
#29718=CARTESIAN_POINT('Ctrl Pts',(8.59489616869782,-49.1867511126203,-4.9622656166752));
#29719=CARTESIAN_POINT('Ctrl Pts',(5.72993077911996,-49.0117511126203,-9.92453123332976));
#29720=CARTESIAN_POINT('Ctrl Pts',(-1.78726082715848E-11,-48.8367511126203,
-9.92453123331945));
#29721=CARTESIAN_POINT('Ctrl Pts',(-5.7299307791557,-48.6617511126203,-9.92453123330913));
#29722=CARTESIAN_POINT('Ctrl Pts',(-8.59489616871569,-48.4867511126203,
-4.96226561664425));
#29723=CARTESIAN_POINT('Ctrl Pts',(-11.4598615582757,-48.3117511126203,
2.06368086793017E-11));
#29724=CARTESIAN_POINT('Ctrl Pts',(-8.59489616869782,-48.1367511126203,
4.9622656166752));
#29725=CARTESIAN_POINT('Ctrl Pts',(-5.72993077911996,-47.9617511126203,
9.92453123332977));
#29726=CARTESIAN_POINT('Ctrl Pts',(1.7871392867044E-11,-47.7867511126204,
9.92453123331945));
#29727=CARTESIAN_POINT('Ctrl Pts',(5.7299307791557,-47.6117511126203,9.92453123330913));
#29728=CARTESIAN_POINT('Ctrl Pts',(8.59489616871569,-47.4367511126203,4.96226561664425));
#29729=CARTESIAN_POINT('Ctrl Pts',(11.4598615582757,-47.2617511126203,-2.06354052510241E-11));
#29730=CARTESIAN_POINT('Ctrl Pts',(8.59489616869782,-47.0867511126203,-4.9622656166752));
#29731=CARTESIAN_POINT('Ctrl Pts',(5.72993077911996,-46.9117511126203,-9.92453123332976));
#29732=CARTESIAN_POINT('Ctrl Pts',(-1.78726082715848E-11,-46.7367511126204,
-9.92453123331945));
#29733=CARTESIAN_POINT('Ctrl Pts',(-5.7299307791557,-46.5617511126203,-9.92453123330913));
#29734=CARTESIAN_POINT('Ctrl Pts',(-8.59489616871569,-46.3867511126203,
-4.96226561664425));
#29735=CARTESIAN_POINT('Ctrl Pts',(-11.4598615582757,-46.2117511126203,
2.06368086793017E-11));
#29736=CARTESIAN_POINT('Ctrl Pts',(-8.59489616869782,-46.0367511126203,
4.9622656166752));
#29737=CARTESIAN_POINT('Ctrl Pts',(-5.72993077911996,-45.8617511126203,
9.92453123332977));
#29738=CARTESIAN_POINT('Ctrl Pts',(1.7871392867044E-11,-45.6867511126203,
9.92453123331945));
#29739=CARTESIAN_POINT('Ctrl Pts',(5.7299307791557,-45.5117511126203,9.92453123330913));
#29740=CARTESIAN_POINT('Ctrl Pts',(8.59489616871569,-45.3367511126203,4.96226561664425));
#29741=CARTESIAN_POINT('Ctrl Pts',(11.4598615582757,-45.1617511126203,-2.06354052510241E-11));
#29742=CARTESIAN_POINT('Ctrl Pts',(8.59489616869782,-44.9867511126203,-4.9622656166752));
#29743=CARTESIAN_POINT('Ctrl Pts',(5.72993077911996,-44.8117511126203,-9.92453123332976));
#29744=CARTESIAN_POINT('Ctrl Pts',(-1.78726082715848E-11,-44.6367511126203,
-9.92453123331945));
#29745=CARTESIAN_POINT('Ctrl Pts',(-1.51301075899711E-11,-213.943984254242,
-8.40164026751963));
#29746=CARTESIAN_POINT('Ctrl Pts',(-4.85068927010198,-213.768984254242,
-8.40164026751089));
#29747=CARTESIAN_POINT('Ctrl Pts',(-7.27603390513785,-213.593984254242,
-4.20082013374671));
#29748=CARTESIAN_POINT('Ctrl Pts',(-9.70137854017371,-213.418984254242,
1.74701493417668E-11));
#29749=CARTESIAN_POINT('Ctrl Pts',(-7.27603390512272,-213.243984254242,
4.20082013377291));
#29750=CARTESIAN_POINT('Ctrl Pts',(-4.85068927007173,-213.068984254242,
8.40164026752836));
#29751=CARTESIAN_POINT('Ctrl Pts',(1.5129078685785E-11,-212.893984254242,
8.40164026751963));
#29752=CARTESIAN_POINT('Ctrl Pts',(4.85068927010198,-212.718984254242,8.40164026751089));
#29753=CARTESIAN_POINT('Ctrl Pts',(7.27603390513785,-212.543984254242,4.20082013374671));
#29754=CARTESIAN_POINT('Ctrl Pts',(9.70137854017371,-212.368984254242,-1.74689612655491E-11));
#29755=CARTESIAN_POINT('Ctrl Pts',(7.27603390512272,-212.193984254242,-4.20082013377291));
#29756=CARTESIAN_POINT('Ctrl Pts',(4.85068927007173,-212.018984254242,-8.40164026752836));
#29757=CARTESIAN_POINT('Ctrl Pts',(-1.51301075899711E-11,-211.843984254242,
-8.40164026751963));
#29758=CARTESIAN_POINT('Ctrl Pts',(-4.85068927010198,-211.668984254242,
-8.40164026751089));
#29759=CARTESIAN_POINT('Ctrl Pts',(-7.27603390513785,-211.493984254242,
-4.20082013374671));
#29760=CARTESIAN_POINT('Ctrl Pts',(-9.70137854017371,-211.318984254242,
1.74701493417668E-11));
#29761=CARTESIAN_POINT('Ctrl Pts',(-7.27603390512272,-211.143984254242,
4.20082013377291));
#29762=CARTESIAN_POINT('Ctrl Pts',(-4.85068927007173,-210.968984254242,
8.40164026752836));
#29763=CARTESIAN_POINT('Ctrl Pts',(1.5129078685785E-11,-210.793984254242,
8.40164026751963));
#29764=CARTESIAN_POINT('Ctrl Pts',(4.85068927010198,-210.618984254242,8.40164026751089));
#29765=CARTESIAN_POINT('Ctrl Pts',(7.27603390513785,-210.443984254242,4.20082013374671));
#29766=CARTESIAN_POINT('Ctrl Pts',(9.70137854017371,-210.268984254242,-1.74689612655491E-11));
#29767=CARTESIAN_POINT('Ctrl Pts',(7.27603390512272,-210.093984254242,-4.20082013377291));
#29768=CARTESIAN_POINT('Ctrl Pts',(4.85068927007173,-209.918984254242,-8.40164026752836));
#29769=CARTESIAN_POINT('Ctrl Pts',(-1.51301075899711E-11,-209.743984254242,
-8.40164026751963));
#29770=CARTESIAN_POINT('Ctrl Pts',(-4.85068927010198,-209.568984254242,
-8.40164026751089));
#29771=CARTESIAN_POINT('Ctrl Pts',(-7.27603390513785,-209.393984254242,
-4.20082013374671));
#29772=CARTESIAN_POINT('Ctrl Pts',(-9.70137854017371,-209.218984254242,
1.74701493417668E-11));
#29773=CARTESIAN_POINT('Ctrl Pts',(-7.27603390512272,-209.043984254242,
4.20082013377291));
#29774=CARTESIAN_POINT('Ctrl Pts',(-4.85068927007173,-208.868984254242,
8.40164026752836));
#29775=CARTESIAN_POINT('Ctrl Pts',(1.5129078685785E-11,-208.693984254242,
8.40164026751963));
#29776=CARTESIAN_POINT('Ctrl Pts',(4.85068927010198,-208.518984254242,8.40164026751089));
#29777=CARTESIAN_POINT('Ctrl Pts',(7.27603390513785,-208.343984254242,4.20082013374671));
#29778=CARTESIAN_POINT('Ctrl Pts',(9.70137854017371,-208.168984254242,-1.74689612655491E-11));
#29779=CARTESIAN_POINT('Ctrl Pts',(7.27603390512272,-207.993984254242,-4.20082013377291));
#29780=CARTESIAN_POINT('Ctrl Pts',(4.85068927007173,-207.818984254242,-8.40164026752836));
#29781=CARTESIAN_POINT('Ctrl Pts',(-1.51301075899711E-11,-207.643984254242,
-8.40164026751963));
#29782=CARTESIAN_POINT('Ctrl Pts',(-4.85068927010198,-207.468984254242,
-8.40164026751089));
#29783=CARTESIAN_POINT('Ctrl Pts',(-7.27603390513785,-207.293984254242,
-4.20082013374671));
#29784=CARTESIAN_POINT('Ctrl Pts',(-9.70137854017371,-207.118984254242,
1.74701493417668E-11));
#29785=CARTESIAN_POINT('Ctrl Pts',(-7.27603390512272,-206.943984254242,
4.20082013377291));
#29786=CARTESIAN_POINT('Ctrl Pts',(-4.85068927007173,-206.768984254242,
8.40164026752836));
#29787=CARTESIAN_POINT('Ctrl Pts',(1.5129078685785E-11,-206.593984254242,
8.40164026751963));
#29788=CARTESIAN_POINT('Ctrl Pts',(4.85068927010198,-206.418984254242,8.40164026751089));
#29789=CARTESIAN_POINT('Ctrl Pts',(7.27603390513785,-206.243984254242,4.20082013374671));
#29790=CARTESIAN_POINT('Ctrl Pts',(9.70137854017371,-206.068984254242,-1.74689612655491E-11));
#29791=CARTESIAN_POINT('Ctrl Pts',(7.27603390512272,-205.893984254242,-4.20082013377291));
#29792=CARTESIAN_POINT('Ctrl Pts',(4.85068927007173,-205.718984254242,-8.40164026752836));
#29793=CARTESIAN_POINT('Ctrl Pts',(-1.51301075899711E-11,-205.543984254242,
-8.40164026751963));
#29794=CARTESIAN_POINT('Ctrl Pts',(-4.85068927010198,-205.368984254242,
-8.40164026751089));
#29795=CARTESIAN_POINT('Ctrl Pts',(-7.27603390513785,-205.193984254242,
-4.20082013374671));
#29796=CARTESIAN_POINT('Ctrl Pts',(-9.70137854017371,-205.018984254242,
1.74701493417668E-11));
#29797=CARTESIAN_POINT('Ctrl Pts',(-7.27603390512272,-204.843984254242,
4.20082013377291));
#29798=CARTESIAN_POINT('Ctrl Pts',(-4.85068927007173,-204.668984254242,
8.40164026752836));
#29799=CARTESIAN_POINT('Ctrl Pts',(1.5129078685785E-11,-204.493984254242,
8.40164026751963));
#29800=CARTESIAN_POINT('Ctrl Pts',(4.85068927010198,-204.318984254242,8.40164026751089));
#29801=CARTESIAN_POINT('Ctrl Pts',(7.27603390513785,-204.143984254242,4.20082013374671));
#29802=CARTESIAN_POINT('Ctrl Pts',(9.70137854017371,-203.968984254242,-1.74689612655491E-11));
#29803=CARTESIAN_POINT('Ctrl Pts',(7.27603390512272,-203.793984254242,-4.20082013377291));
#29804=CARTESIAN_POINT('Ctrl Pts',(4.85068927007173,-203.618984254242,-8.40164026752836));
#29805=CARTESIAN_POINT('Ctrl Pts',(-1.51301075899711E-11,-203.443984254242,
-8.40164026751963));
#29806=CARTESIAN_POINT('Ctrl Pts',(-4.85068927010198,-203.268984254242,
-8.40164026751089));
#29807=CARTESIAN_POINT('Ctrl Pts',(-7.27603390513785,-203.093984254242,
-4.20082013374671));
#29808=CARTESIAN_POINT('Ctrl Pts',(-9.70137854017371,-202.918984254242,
1.74701493417668E-11));
#29809=CARTESIAN_POINT('Ctrl Pts',(-7.27603390512272,-202.743984254242,
4.20082013377291));
#29810=CARTESIAN_POINT('Ctrl Pts',(-4.85068927007173,-202.568984254242,
8.40164026752836));
#29811=CARTESIAN_POINT('Ctrl Pts',(1.5129078685785E-11,-202.393984254242,
8.40164026751963));
#29812=CARTESIAN_POINT('Ctrl Pts',(4.85068927010198,-202.218984254242,8.40164026751089));
#29813=CARTESIAN_POINT('Ctrl Pts',(7.27603390513785,-202.043984254242,4.20082013374671));
#29814=CARTESIAN_POINT('Ctrl Pts',(9.70137854017371,-201.868984254242,-1.74689612655491E-11));
#29815=CARTESIAN_POINT('Ctrl Pts',(7.27603390512272,-201.693984254242,-4.20082013377291));
#29816=CARTESIAN_POINT('Ctrl Pts',(4.85068927007173,-201.518984254242,-8.40164026752836));
#29817=CARTESIAN_POINT('Ctrl Pts',(-1.51301075899711E-11,-201.343984254242,
-8.40164026751963));
#29818=CARTESIAN_POINT('Ctrl Pts',(-4.85068927010198,-201.168984254242,
-8.40164026751089));
#29819=CARTESIAN_POINT('Ctrl Pts',(-7.27603390513785,-200.993984254242,
-4.20082013374671));
#29820=CARTESIAN_POINT('Ctrl Pts',(-9.70137854017371,-200.818984254242,
1.74701493417668E-11));
#29821=CARTESIAN_POINT('Ctrl Pts',(-7.27603390512272,-200.643984254242,
4.20082013377291));
#29822=CARTESIAN_POINT('Ctrl Pts',(-4.85068927007173,-200.468984254242,
8.40164026752836));
#29823=CARTESIAN_POINT('Ctrl Pts',(1.5129078685785E-11,-200.293984254242,
8.40164026751963));
#29824=CARTESIAN_POINT('Ctrl Pts',(4.85068927010198,-200.118984254242,8.40164026751089));
#29825=CARTESIAN_POINT('Ctrl Pts',(7.27603390513785,-199.943984254242,4.20082013374671));
#29826=CARTESIAN_POINT('Ctrl Pts',(9.70137854017371,-199.768984254242,-1.74689612655491E-11));
#29827=CARTESIAN_POINT('Ctrl Pts',(7.27603390512272,-199.593984254242,-4.20082013377291));
#29828=CARTESIAN_POINT('Ctrl Pts',(4.85068927007173,-199.418984254242,-8.40164026752836));
#29829=CARTESIAN_POINT('Ctrl Pts',(-1.51301075899711E-11,-199.243984254242,
-8.40164026751963));
#29830=CARTESIAN_POINT('Ctrl Pts',(-4.85068927010198,-199.068984254242,
-8.40164026751089));
#29831=CARTESIAN_POINT('Ctrl Pts',(-7.27603390513785,-198.893984254242,
-4.20082013374671));
#29832=CARTESIAN_POINT('Ctrl Pts',(-9.70137854017371,-198.718984254242,
1.74701493417668E-11));
#29833=CARTESIAN_POINT('Ctrl Pts',(-7.27603390512272,-198.543984254242,
4.20082013377291));
#29834=CARTESIAN_POINT('Ctrl Pts',(-4.85068927007173,-198.368984254242,
8.40164026752836));
#29835=CARTESIAN_POINT('Ctrl Pts',(1.5129078685785E-11,-198.193984254242,
8.40164026751963));
#29836=CARTESIAN_POINT('Ctrl Pts',(4.85068927010198,-198.018984254242,8.40164026751089));
#29837=CARTESIAN_POINT('Ctrl Pts',(7.27603390513785,-197.843984254242,4.20082013374671));
#29838=CARTESIAN_POINT('Ctrl Pts',(9.70137854017371,-197.668984254242,-1.74689612655491E-11));
#29839=CARTESIAN_POINT('Ctrl Pts',(7.27603390512272,-197.493984254242,-4.20082013377291));
#29840=CARTESIAN_POINT('Ctrl Pts',(4.85068927007173,-197.318984254242,-8.40164026752836));
#29841=CARTESIAN_POINT('Ctrl Pts',(-1.51301075899711E-11,-197.143984254242,
-8.40164026751963));
#29842=CARTESIAN_POINT('Ctrl Pts',(-4.85068927010198,-196.968984254242,
-8.40164026751089));
#29843=CARTESIAN_POINT('Ctrl Pts',(-7.27603390513785,-196.793984254242,
-4.20082013374671));
#29844=CARTESIAN_POINT('Ctrl Pts',(-9.70137854017371,-196.618984254242,
1.74701493417668E-11));
#29845=CARTESIAN_POINT('Ctrl Pts',(-7.27603390512272,-196.443984254242,
4.20082013377291));
#29846=CARTESIAN_POINT('Ctrl Pts',(-4.85068927007173,-196.268984254242,
8.40164026752836));
#29847=CARTESIAN_POINT('Ctrl Pts',(1.5129078685785E-11,-196.093984254242,
8.40164026751963));
#29848=CARTESIAN_POINT('Ctrl Pts',(4.85068927010198,-195.918984254242,8.40164026751089));
#29849=CARTESIAN_POINT('Ctrl Pts',(7.27603390513785,-195.743984254242,4.20082013374671));
#29850=CARTESIAN_POINT('Ctrl Pts',(9.70137854017371,-195.568984254242,-1.74689612655491E-11));
#29851=CARTESIAN_POINT('Ctrl Pts',(7.27603390512272,-195.393984254242,-4.20082013377291));
#29852=CARTESIAN_POINT('Ctrl Pts',(4.85068927007173,-195.218984254242,-8.40164026752836));
#29853=CARTESIAN_POINT('Ctrl Pts',(-1.51301075899711E-11,-195.043984254242,
-8.40164026751963));
#29854=CARTESIAN_POINT('Ctrl Pts',(-4.85068927010198,-194.868984254242,
-8.40164026751089));
#29855=CARTESIAN_POINT('Ctrl Pts',(-7.27603390513785,-194.693984254242,
-4.20082013374671));
#29856=CARTESIAN_POINT('Ctrl Pts',(-9.70137854017371,-194.518984254242,
1.74701493417668E-11));
#29857=CARTESIAN_POINT('Ctrl Pts',(-7.27603390512272,-194.343984254242,
4.20082013377291));
#29858=CARTESIAN_POINT('Ctrl Pts',(-4.85068927007173,-194.168984254242,
8.40164026752836));
#29859=CARTESIAN_POINT('Ctrl Pts',(1.5129078685785E-11,-193.993984254242,
8.40164026751963));
#29860=CARTESIAN_POINT('Ctrl Pts',(4.85068927010198,-193.818984254242,8.40164026751089));
#29861=CARTESIAN_POINT('Ctrl Pts',(7.27603390513785,-193.643984254242,4.20082013374671));
#29862=CARTESIAN_POINT('Ctrl Pts',(9.70137854017371,-193.468984254242,-1.74689612655491E-11));
#29863=CARTESIAN_POINT('Ctrl Pts',(7.27603390512272,-193.293984254242,-4.20082013377291));
#29864=CARTESIAN_POINT('Ctrl Pts',(4.85068927007173,-193.118984254242,-8.40164026752836));
#29865=CARTESIAN_POINT('Ctrl Pts',(-1.51301075899711E-11,-192.943984254242,
-8.40164026751963));
#29866=CARTESIAN_POINT('Ctrl Pts',(-4.85068927010198,-192.768984254242,
-8.40164026751089));
#29867=CARTESIAN_POINT('Ctrl Pts',(-7.27603390513785,-192.593984254242,
-4.20082013374671));
#29868=CARTESIAN_POINT('Ctrl Pts',(-9.70137854017371,-192.418984254242,
1.74701493417668E-11));
#29869=CARTESIAN_POINT('Ctrl Pts',(-7.27603390512272,-192.243984254242,
4.20082013377291));
#29870=CARTESIAN_POINT('Ctrl Pts',(-4.85068927007173,-192.068984254242,
8.40164026752836));
#29871=CARTESIAN_POINT('Ctrl Pts',(1.5129078685785E-11,-191.893984254242,
8.40164026751963));
#29872=CARTESIAN_POINT('Ctrl Pts',(4.85068927010198,-191.718984254242,8.40164026751089));
#29873=CARTESIAN_POINT('Ctrl Pts',(7.27603390513785,-191.543984254242,4.20082013374671));
#29874=CARTESIAN_POINT('Ctrl Pts',(9.70137854017371,-191.368984254242,-1.74689612655491E-11));
#29875=CARTESIAN_POINT('Ctrl Pts',(7.27603390512272,-191.193984254242,-4.20082013377291));
#29876=CARTESIAN_POINT('Ctrl Pts',(4.85068927007173,-191.018984254242,-8.40164026752836));
#29877=CARTESIAN_POINT('Ctrl Pts',(-1.51301075899711E-11,-190.843984254242,
-8.40164026751963));
#29878=CARTESIAN_POINT('Ctrl Pts',(-4.85068927010198,-190.668984254242,
-8.40164026751089));
#29879=CARTESIAN_POINT('Ctrl Pts',(-7.27603390513785,-190.493984254242,
-4.20082013374671));
#29880=CARTESIAN_POINT('Ctrl Pts',(-9.70137854017371,-190.318984254242,
1.74701493417668E-11));
#29881=CARTESIAN_POINT('Ctrl Pts',(-7.27603390512272,-190.143984254242,
4.20082013377291));
#29882=CARTESIAN_POINT('Ctrl Pts',(-4.85068927007173,-189.968984254242,
8.40164026752836));
#29883=CARTESIAN_POINT('Ctrl Pts',(1.5129078685785E-11,-189.793984254242,
8.40164026751963));
#29884=CARTESIAN_POINT('Ctrl Pts',(4.85068927010198,-189.618984254242,8.40164026751089));
#29885=CARTESIAN_POINT('Ctrl Pts',(7.27603390513785,-189.443984254242,4.20082013374671));
#29886=CARTESIAN_POINT('Ctrl Pts',(9.70137854017371,-189.268984254242,-1.74689612655491E-11));
#29887=CARTESIAN_POINT('Ctrl Pts',(7.27603390512272,-189.093984254242,-4.20082013377291));
#29888=CARTESIAN_POINT('Ctrl Pts',(4.85068927007173,-188.918984254242,-8.40164026752836));
#29889=CARTESIAN_POINT('Ctrl Pts',(-1.51301075899711E-11,-188.743984254242,
-8.40164026751963));
#29890=CARTESIAN_POINT('Ctrl Pts',(-4.85068927010198,-188.568984254242,
-8.40164026751089));
#29891=CARTESIAN_POINT('Ctrl Pts',(-7.27603390513785,-188.393984254242,
-4.20082013374671));
#29892=CARTESIAN_POINT('Ctrl Pts',(-9.70137854017371,-188.218984254242,
1.74701493417668E-11));
#29893=CARTESIAN_POINT('Ctrl Pts',(-7.27603390512272,-188.043984254242,
4.20082013377291));
#29894=CARTESIAN_POINT('Ctrl Pts',(-4.85068927007173,-187.868984254242,
8.40164026752836));
#29895=CARTESIAN_POINT('Ctrl Pts',(1.5129078685785E-11,-187.693984254242,
8.40164026751963));
#29896=CARTESIAN_POINT('Ctrl Pts',(4.85068927010198,-187.518984254242,8.40164026751089));
#29897=CARTESIAN_POINT('Ctrl Pts',(7.27603390513785,-187.343984254242,4.20082013374671));
#29898=CARTESIAN_POINT('Ctrl Pts',(9.70137854017371,-187.168984254242,-1.74689612655491E-11));
#29899=CARTESIAN_POINT('Ctrl Pts',(7.27603390512272,-186.993984254242,-4.20082013377291));
#29900=CARTESIAN_POINT('Ctrl Pts',(4.85068927007173,-186.818984254242,-8.40164026752836));
#29901=CARTESIAN_POINT('Ctrl Pts',(-1.51301075899711E-11,-186.643984254242,
-8.40164026751963));
#29902=CARTESIAN_POINT('Ctrl Pts',(-4.85068927010198,-186.468984254242,
-8.40164026751089));
#29903=CARTESIAN_POINT('Ctrl Pts',(-7.27603390513785,-186.293984254242,
-4.20082013374671));
#29904=CARTESIAN_POINT('Ctrl Pts',(-9.70137854017371,-186.118984254242,
1.74701493417668E-11));
#29905=CARTESIAN_POINT('Ctrl Pts',(-7.27603390512272,-185.943984254242,
4.20082013377291));
#29906=CARTESIAN_POINT('Ctrl Pts',(-4.85068927007173,-185.768984254242,
8.40164026752836));
#29907=CARTESIAN_POINT('Ctrl Pts',(1.5129078685785E-11,-185.593984254242,
8.40164026751963));
#29908=CARTESIAN_POINT('Ctrl Pts',(4.85068927010198,-185.418984254242,8.40164026751089));
#29909=CARTESIAN_POINT('Ctrl Pts',(7.27603390513785,-185.243984254242,4.20082013374671));
#29910=CARTESIAN_POINT('Ctrl Pts',(9.70137854017371,-185.068984254242,-1.74689612655491E-11));
#29911=CARTESIAN_POINT('Ctrl Pts',(7.27603390512272,-184.893984254242,-4.20082013377291));
#29912=CARTESIAN_POINT('Ctrl Pts',(4.85068927007173,-184.718984254242,-8.40164026752836));
#29913=CARTESIAN_POINT('Ctrl Pts',(-1.51301075899711E-11,-184.543984254242,
-8.40164026751963));
#29914=CARTESIAN_POINT('Ctrl Pts',(-4.85068927010198,-184.368984254242,
-8.40164026751089));
#29915=CARTESIAN_POINT('Ctrl Pts',(-7.27603390513785,-184.193984254242,
-4.20082013374671));
#29916=CARTESIAN_POINT('Ctrl Pts',(-9.70137854017371,-184.018984254242,
1.74701493417668E-11));
#29917=CARTESIAN_POINT('Ctrl Pts',(-7.27603390512272,-183.843984254242,
4.20082013377291));
#29918=CARTESIAN_POINT('Ctrl Pts',(-4.85068927007173,-183.668984254242,
8.40164026752836));
#29919=CARTESIAN_POINT('Ctrl Pts',(1.5129078685785E-11,-183.493984254242,
8.40164026751963));
#29920=CARTESIAN_POINT('Ctrl Pts',(4.85068927010198,-183.318984254242,8.40164026751089));
#29921=CARTESIAN_POINT('Ctrl Pts',(7.27603390513785,-183.143984254242,4.20082013374671));
#29922=CARTESIAN_POINT('Ctrl Pts',(9.70137854017371,-182.968984254242,-1.74689612655491E-11));
#29923=CARTESIAN_POINT('Ctrl Pts',(7.27603390512272,-182.793984254242,-4.20082013377291));
#29924=CARTESIAN_POINT('Ctrl Pts',(4.85068927007173,-182.618984254242,-8.40164026752836));
#29925=CARTESIAN_POINT('Ctrl Pts',(-1.51301075899711E-11,-182.443984254242,
-8.40164026751963));
#29926=CARTESIAN_POINT('Ctrl Pts',(-4.85068927010198,-182.268984254242,
-8.40164026751089));
#29927=CARTESIAN_POINT('Ctrl Pts',(-7.27603390513785,-182.093984254242,
-4.20082013374671));
#29928=CARTESIAN_POINT('Ctrl Pts',(-9.70137854017371,-181.918984254242,
1.74701493417668E-11));
#29929=CARTESIAN_POINT('Ctrl Pts',(-7.27603390512272,-181.743984254242,
4.20082013377291));
#29930=CARTESIAN_POINT('Ctrl Pts',(-4.85068927007173,-181.568984254242,
8.40164026752836));
#29931=CARTESIAN_POINT('Ctrl Pts',(1.5129078685785E-11,-181.393984254242,
8.40164026751963));
#29932=CARTESIAN_POINT('Ctrl Pts',(4.85068927010198,-181.218984254242,8.40164026751089));
#29933=CARTESIAN_POINT('Ctrl Pts',(7.27603390513785,-181.043984254242,4.20082013374671));
#29934=CARTESIAN_POINT('Ctrl Pts',(9.70137854017371,-180.868984254242,-1.74689612655491E-11));
#29935=CARTESIAN_POINT('Ctrl Pts',(7.27603390512272,-180.693984254242,-4.20082013377291));
#29936=CARTESIAN_POINT('Ctrl Pts',(4.85068927007173,-180.518984254242,-8.40164026752836));
#29937=CARTESIAN_POINT('Ctrl Pts',(-1.51301075899711E-11,-180.343984254242,
-8.40164026751963));
#29938=CARTESIAN_POINT('Ctrl Pts',(-4.85068927010198,-180.168984254242,
-8.40164026751089));
#29939=CARTESIAN_POINT('Ctrl Pts',(-7.27603390513785,-179.993984254242,
-4.20082013374671));
#29940=CARTESIAN_POINT('Ctrl Pts',(-9.70137854017371,-179.818984254242,
1.74701493417668E-11));
#29941=CARTESIAN_POINT('Ctrl Pts',(-7.27603390512272,-179.643984254242,
4.20082013377291));
#29942=CARTESIAN_POINT('Ctrl Pts',(-4.85068927007173,-179.468984254242,
8.40164026752836));
#29943=CARTESIAN_POINT('Ctrl Pts',(1.5129078685785E-11,-179.293984254242,
8.40164026751963));
#29944=CARTESIAN_POINT('Ctrl Pts',(4.85068927010198,-179.118984254242,8.40164026751089));
#29945=CARTESIAN_POINT('Ctrl Pts',(7.27603390513785,-178.943984254242,4.20082013374671));
#29946=CARTESIAN_POINT('Ctrl Pts',(9.70137854017371,-178.768984254242,-1.74689612655491E-11));
#29947=CARTESIAN_POINT('Ctrl Pts',(7.27603390512272,-178.593984254242,-4.20082013377291));
#29948=CARTESIAN_POINT('Ctrl Pts',(4.85068927007173,-178.418984254242,-8.40164026752836));
#29949=CARTESIAN_POINT('Ctrl Pts',(-1.51301075899711E-11,-178.243984254242,
-8.40164026751963));
#29950=CARTESIAN_POINT('Ctrl Pts',(-4.85068927010198,-178.068984254242,
-8.40164026751089));
#29951=CARTESIAN_POINT('Ctrl Pts',(-7.27603390513785,-177.893984254242,
-4.20082013374671));
#29952=CARTESIAN_POINT('Ctrl Pts',(-9.70137854017371,-177.718984254242,
1.74701493417668E-11));
#29953=CARTESIAN_POINT('Ctrl Pts',(-7.27603390512272,-177.543984254242,
4.20082013377291));
#29954=CARTESIAN_POINT('Ctrl Pts',(-4.85068927007173,-177.368984254242,
8.40164026752836));
#29955=CARTESIAN_POINT('Ctrl Pts',(1.5129078685785E-11,-177.193984254242,
8.40164026751963));
#29956=CARTESIAN_POINT('Ctrl Pts',(4.85068927010198,-177.018984254242,8.40164026751089));
#29957=CARTESIAN_POINT('Ctrl Pts',(7.27603390513785,-176.843984254242,4.20082013374671));
#29958=CARTESIAN_POINT('Ctrl Pts',(9.70137854017371,-176.668984254242,-1.74689612655491E-11));
#29959=CARTESIAN_POINT('Ctrl Pts',(7.27603390512272,-176.493984254242,-4.20082013377291));
#29960=CARTESIAN_POINT('Ctrl Pts',(4.85068927007173,-176.318984254242,-8.40164026752836));
#29961=CARTESIAN_POINT('Ctrl Pts',(-1.51301075899711E-11,-176.143984254242,
-8.40164026751963));
#29962=CARTESIAN_POINT('Ctrl Pts',(-4.85068927010198,-175.968984254242,
-8.40164026751089));
#29963=CARTESIAN_POINT('Ctrl Pts',(-7.27603390513785,-175.793984254242,
-4.20082013374671));
#29964=CARTESIAN_POINT('Ctrl Pts',(-9.70137854017371,-175.618984254242,
1.74701493417668E-11));
#29965=CARTESIAN_POINT('Ctrl Pts',(-7.27603390512272,-175.443984254242,
4.20082013377291));
#29966=CARTESIAN_POINT('Ctrl Pts',(-4.85068927007173,-175.268984254242,
8.40164026752836));
#29967=CARTESIAN_POINT('Ctrl Pts',(1.5129078685785E-11,-175.093984254242,
8.40164026751963));
#29968=CARTESIAN_POINT('Ctrl Pts',(4.85068927010198,-174.918984254242,8.40164026751089));
#29969=CARTESIAN_POINT('Ctrl Pts',(7.27603390513785,-174.743984254242,4.20082013374671));
#29970=CARTESIAN_POINT('Ctrl Pts',(9.70137854017371,-174.568984254242,-1.74689612655491E-11));
#29971=CARTESIAN_POINT('Ctrl Pts',(7.27603390512272,-174.393984254242,-4.20082013377291));
#29972=CARTESIAN_POINT('Ctrl Pts',(4.85068927007173,-174.218984254242,-8.40164026752836));
#29973=CARTESIAN_POINT('Ctrl Pts',(-1.51301075899711E-11,-174.043984254242,
-8.40164026751963));
#29974=CARTESIAN_POINT('Ctrl Pts',(-4.85068927010198,-173.868984254242,
-8.40164026751089));
#29975=CARTESIAN_POINT('Ctrl Pts',(-7.27603390513785,-173.693984254242,
-4.20082013374671));
#29976=CARTESIAN_POINT('Ctrl Pts',(-9.70137854017371,-173.518984254242,
1.74701493417668E-11));
#29977=CARTESIAN_POINT('Ctrl Pts',(-7.27603390512272,-173.343984254242,
4.20082013377291));
#29978=CARTESIAN_POINT('Ctrl Pts',(-4.85068927007173,-173.168984254242,
8.40164026752836));
#29979=CARTESIAN_POINT('Ctrl Pts',(1.5129078685785E-11,-172.993984254242,
8.40164026751963));
#29980=CARTESIAN_POINT('Ctrl Pts',(4.85068927010198,-172.818984254242,8.40164026751089));
#29981=CARTESIAN_POINT('Ctrl Pts',(7.27603390513785,-172.643984254242,4.20082013374671));
#29982=CARTESIAN_POINT('Ctrl Pts',(9.70137854017371,-172.468984254242,-1.74689612655491E-11));
#29983=CARTESIAN_POINT('Ctrl Pts',(7.27603390512272,-172.293984254242,-4.20082013377291));
#29984=CARTESIAN_POINT('Ctrl Pts',(4.85068927007173,-172.118984254242,-8.40164026752836));
#29985=CARTESIAN_POINT('Ctrl Pts',(-1.51301075899711E-11,-171.943984254242,
-8.40164026751963));
#29986=CARTESIAN_POINT('Ctrl Pts',(-4.85068927010198,-171.768984254242,
-8.40164026751089));
#29987=CARTESIAN_POINT('Ctrl Pts',(-7.27603390513785,-171.593984254242,
-4.20082013374671));
#29988=CARTESIAN_POINT('Ctrl Pts',(-9.70137854017371,-171.418984254242,
1.74701493417668E-11));
#29989=CARTESIAN_POINT('Ctrl Pts',(-7.27603390512272,-171.243984254242,
4.20082013377291));
#29990=CARTESIAN_POINT('Ctrl Pts',(-4.85068927007173,-171.068984254242,
8.40164026752836));
#29991=CARTESIAN_POINT('Ctrl Pts',(1.5129078685785E-11,-170.893984254242,
8.40164026751963));
#29992=CARTESIAN_POINT('Ctrl Pts',(4.85068927010198,-170.718984254242,8.40164026751089));
#29993=CARTESIAN_POINT('Ctrl Pts',(7.27603390513785,-170.543984254242,4.20082013374671));
#29994=CARTESIAN_POINT('Ctrl Pts',(9.70137854017371,-170.368984254242,-1.74689612655491E-11));
#29995=CARTESIAN_POINT('Ctrl Pts',(7.27603390512272,-170.193984254242,-4.20082013377291));
#29996=CARTESIAN_POINT('Ctrl Pts',(4.85068927007173,-170.018984254242,-8.40164026752836));
#29997=CARTESIAN_POINT('Ctrl Pts',(-1.51301075899711E-11,-169.843984254242,
-8.40164026751963));
#29998=CARTESIAN_POINT('Ctrl Pts',(-4.85068927010198,-169.668984254242,
-8.40164026751089));
#29999=CARTESIAN_POINT('Ctrl Pts',(-7.27603390513785,-169.493984254242,
-4.20082013374671));
#30000=CARTESIAN_POINT('Ctrl Pts',(-9.70137854017371,-169.318984254242,
1.74701493417668E-11));
#30001=CARTESIAN_POINT('Ctrl Pts',(-7.27603390512272,-169.143984254242,
4.20082013377291));
#30002=CARTESIAN_POINT('Ctrl Pts',(-4.85068927007173,-168.968984254242,
8.40164026752836));
#30003=CARTESIAN_POINT('Ctrl Pts',(1.5129078685785E-11,-168.793984254242,
8.40164026751963));
#30004=CARTESIAN_POINT('Ctrl Pts',(4.85068927010198,-168.618984254242,8.40164026751089));
#30005=CARTESIAN_POINT('Ctrl Pts',(7.27603390513785,-168.443984254242,4.20082013374671));
#30006=CARTESIAN_POINT('Ctrl Pts',(9.70137854017371,-168.268984254242,-1.74689612655491E-11));
#30007=CARTESIAN_POINT('Ctrl Pts',(7.27603390512272,-168.093984254242,-4.20082013377291));
#30008=CARTESIAN_POINT('Ctrl Pts',(4.85068927007173,-167.918984254242,-8.40164026752836));
#30009=CARTESIAN_POINT('Ctrl Pts',(-1.51301075899711E-11,-167.743984254242,
-8.40164026751963));
#30010=CARTESIAN_POINT('Ctrl Pts',(-4.85068927010198,-167.568984254242,
-8.40164026751089));
#30011=CARTESIAN_POINT('Ctrl Pts',(-7.27603390513785,-167.393984254242,
-4.20082013374671));
#30012=CARTESIAN_POINT('Ctrl Pts',(-9.70137854017371,-167.218984254242,
1.74701493417668E-11));
#30013=CARTESIAN_POINT('Ctrl Pts',(-7.27603390512272,-167.043984254242,
4.20082013377291));
#30014=CARTESIAN_POINT('Ctrl Pts',(-4.85068927007173,-166.868984254242,
8.40164026752836));
#30015=CARTESIAN_POINT('Ctrl Pts',(1.5129078685785E-11,-166.693984254242,
8.40164026751963));
#30016=CARTESIAN_POINT('Ctrl Pts',(4.85068927010198,-166.518984254242,8.40164026751089));
#30017=CARTESIAN_POINT('Ctrl Pts',(7.27603390513785,-166.343984254242,4.20082013374671));
#30018=CARTESIAN_POINT('Ctrl Pts',(9.70137854017371,-166.168984254242,-1.74689612655491E-11));
#30019=CARTESIAN_POINT('Ctrl Pts',(7.27603390512272,-165.993984254242,-4.20082013377291));
#30020=CARTESIAN_POINT('Ctrl Pts',(4.85068927007173,-165.818984254242,-8.40164026752836));
#30021=CARTESIAN_POINT('Ctrl Pts',(-1.51301075899711E-11,-165.643984254242,
-8.40164026751963));
#30022=CARTESIAN_POINT('Ctrl Pts',(-4.85068927010198,-165.468984254242,
-8.40164026751089));
#30023=CARTESIAN_POINT('Ctrl Pts',(-7.27603390513785,-165.293984254242,
-4.20082013374671));
#30024=CARTESIAN_POINT('Ctrl Pts',(-9.70137854017371,-165.118984254242,
1.74701493417668E-11));
#30025=CARTESIAN_POINT('Ctrl Pts',(-7.27603390512272,-164.943984254242,
4.20082013377291));
#30026=CARTESIAN_POINT('Ctrl Pts',(-4.85068927007173,-164.768984254242,
8.40164026752836));
#30027=CARTESIAN_POINT('Ctrl Pts',(1.5129078685785E-11,-164.593984254242,
8.40164026751963));
#30028=CARTESIAN_POINT('Ctrl Pts',(4.85068927010198,-164.418984254242,8.40164026751089));
#30029=CARTESIAN_POINT('Ctrl Pts',(7.27603390513785,-164.243984254242,4.20082013374671));
#30030=CARTESIAN_POINT('Ctrl Pts',(9.70137854017371,-164.068984254242,-1.74689612655491E-11));
#30031=CARTESIAN_POINT('Ctrl Pts',(7.27603390512272,-163.893984254242,-4.20082013377291));
#30032=CARTESIAN_POINT('Ctrl Pts',(4.85068927007173,-163.718984254242,-8.40164026752836));
#30033=CARTESIAN_POINT('Ctrl Pts',(-1.51301075899711E-11,-163.543984254242,
-8.40164026751963));
#30034=CARTESIAN_POINT('Ctrl Pts',(-4.85068927010198,-163.368984254242,
-8.40164026751089));
#30035=CARTESIAN_POINT('Ctrl Pts',(-7.27603390513785,-163.193984254242,
-4.20082013374671));
#30036=CARTESIAN_POINT('Ctrl Pts',(-9.70137854017371,-163.018984254242,
1.74701493417668E-11));
#30037=CARTESIAN_POINT('Ctrl Pts',(-7.27603390512272,-162.843984254242,
4.20082013377291));
#30038=CARTESIAN_POINT('Ctrl Pts',(-4.85068927007173,-162.668984254242,
8.40164026752836));
#30039=CARTESIAN_POINT('Ctrl Pts',(1.5129078685785E-11,-162.493984254242,
8.40164026751963));
#30040=CARTESIAN_POINT('Ctrl Pts',(4.85068927010198,-162.318984254242,8.40164026751089));
#30041=CARTESIAN_POINT('Ctrl Pts',(7.27603390513785,-162.143984254242,4.20082013374671));
#30042=CARTESIAN_POINT('Ctrl Pts',(9.70137854017371,-161.968984254242,-1.74689612655491E-11));
#30043=CARTESIAN_POINT('Ctrl Pts',(7.27603390512272,-161.793984254242,-4.20082013377291));
#30044=CARTESIAN_POINT('Ctrl Pts',(4.85068927007173,-161.618984254242,-8.40164026752836));
#30045=CARTESIAN_POINT('Ctrl Pts',(-1.51301075899711E-11,-161.443984254242,
-8.40164026751963));
#30046=CARTESIAN_POINT('Ctrl Pts',(-4.85068927010198,-161.268984254242,
-8.40164026751089));
#30047=CARTESIAN_POINT('Ctrl Pts',(-7.27603390513785,-161.093984254242,
-4.20082013374671));
#30048=CARTESIAN_POINT('Ctrl Pts',(-9.70137854017371,-160.918984254242,
1.74701493417668E-11));
#30049=CARTESIAN_POINT('Ctrl Pts',(-7.27603390512272,-160.743984254242,
4.20082013377291));
#30050=CARTESIAN_POINT('Ctrl Pts',(-4.85068927007173,-160.568984254242,
8.40164026752836));
#30051=CARTESIAN_POINT('Ctrl Pts',(1.5129078685785E-11,-160.393984254242,
8.40164026751963));
#30052=CARTESIAN_POINT('Ctrl Pts',(4.85068927010198,-160.218984254242,8.40164026751089));
#30053=CARTESIAN_POINT('Ctrl Pts',(7.27603390513785,-160.043984254242,4.20082013374671));
#30054=CARTESIAN_POINT('Ctrl Pts',(9.70137854017371,-159.868984254242,-1.74689612655491E-11));
#30055=CARTESIAN_POINT('Ctrl Pts',(7.27603390512272,-159.693984254242,-4.20082013377291));
#30056=CARTESIAN_POINT('Ctrl Pts',(4.85068927007173,-159.518984254242,-8.40164026752836));
#30057=CARTESIAN_POINT('Ctrl Pts',(-1.51301075899711E-11,-159.343984254242,
-8.40164026751963));
#30058=CARTESIAN_POINT('Ctrl Pts',(-4.85068927010198,-159.168984254242,
-8.40164026751089));
#30059=CARTESIAN_POINT('Ctrl Pts',(-7.27603390513785,-158.993984254242,
-4.20082013374671));
#30060=CARTESIAN_POINT('Ctrl Pts',(-9.70137854017371,-158.818984254242,
1.74701493417668E-11));
#30061=CARTESIAN_POINT('Ctrl Pts',(-7.27603390512272,-158.643984254242,
4.20082013377291));
#30062=CARTESIAN_POINT('Ctrl Pts',(-4.85068927007173,-158.468984254242,
8.40164026752836));
#30063=CARTESIAN_POINT('Ctrl Pts',(1.5129078685785E-11,-158.293984254242,
8.40164026751963));
#30064=CARTESIAN_POINT('Ctrl Pts',(4.85068927010198,-158.118984254242,8.40164026751089));
#30065=CARTESIAN_POINT('Ctrl Pts',(7.27603390513785,-157.943984254242,4.20082013374671));
#30066=CARTESIAN_POINT('Ctrl Pts',(9.70137854017371,-157.768984254242,-1.74689612655491E-11));
#30067=CARTESIAN_POINT('Ctrl Pts',(7.27603390512272,-157.593984254242,-4.20082013377291));
#30068=CARTESIAN_POINT('Ctrl Pts',(4.85068927007173,-157.418984254242,-8.40164026752836));
#30069=CARTESIAN_POINT('Ctrl Pts',(-1.51301075899711E-11,-157.243984254242,
-8.40164026751963));
#30070=CARTESIAN_POINT('Ctrl Pts',(-4.85068927010198,-157.068984254242,
-8.40164026751089));
#30071=CARTESIAN_POINT('Ctrl Pts',(-7.27603390513785,-156.893984254242,
-4.20082013374671));
#30072=CARTESIAN_POINT('Ctrl Pts',(-9.70137854017371,-156.718984254242,
1.74701493417668E-11));
#30073=CARTESIAN_POINT('Ctrl Pts',(-7.27603390512272,-156.543984254242,
4.20082013377291));
#30074=CARTESIAN_POINT('Ctrl Pts',(-4.85068927007173,-156.368984254242,
8.40164026752836));
#30075=CARTESIAN_POINT('Ctrl Pts',(1.5129078685785E-11,-156.193984254242,
8.40164026751963));
#30076=CARTESIAN_POINT('Ctrl Pts',(4.85068927010198,-156.018984254242,8.40164026751089));
#30077=CARTESIAN_POINT('Ctrl Pts',(7.27603390513785,-155.843984254242,4.20082013374671));
#30078=CARTESIAN_POINT('Ctrl Pts',(9.70137854017371,-155.668984254242,-1.74689612655491E-11));
#30079=CARTESIAN_POINT('Ctrl Pts',(7.27603390512272,-155.493984254242,-4.20082013377291));
#30080=CARTESIAN_POINT('Ctrl Pts',(4.85068927007173,-155.318984254242,-8.40164026752836));
#30081=CARTESIAN_POINT('Ctrl Pts',(-1.51301075899711E-11,-155.143984254242,
-8.40164026751963));
#30082=CARTESIAN_POINT('Ctrl Pts',(-4.85068927010198,-154.968984254242,
-8.40164026751089));
#30083=CARTESIAN_POINT('Ctrl Pts',(-7.27603390513785,-154.793984254242,
-4.20082013374671));
#30084=CARTESIAN_POINT('Ctrl Pts',(-9.70137854017371,-154.618984254242,
1.74701493417668E-11));
#30085=CARTESIAN_POINT('Ctrl Pts',(-7.27603390512272,-154.443984254242,
4.20082013377291));
#30086=CARTESIAN_POINT('Ctrl Pts',(-4.85068927007173,-154.268984254242,
8.40164026752836));
#30087=CARTESIAN_POINT('Ctrl Pts',(1.5129078685785E-11,-154.093984254242,
8.40164026751963));
#30088=CARTESIAN_POINT('Ctrl Pts',(4.85068927010198,-153.918984254242,8.40164026751089));
#30089=CARTESIAN_POINT('Ctrl Pts',(7.27603390513785,-153.743984254242,4.20082013374671));
#30090=CARTESIAN_POINT('Ctrl Pts',(9.70137854017371,-153.568984254242,-1.74689612655491E-11));
#30091=CARTESIAN_POINT('Ctrl Pts',(7.27603390512272,-153.393984254242,-4.20082013377291));
#30092=CARTESIAN_POINT('Ctrl Pts',(4.85068927007173,-153.218984254242,-8.40164026752836));
#30093=CARTESIAN_POINT('Ctrl Pts',(-1.51301075899711E-11,-153.043984254242,
-8.40164026751963));
#30094=CARTESIAN_POINT('Ctrl Pts',(-4.85068927010198,-152.868984254242,
-8.40164026751089));
#30095=CARTESIAN_POINT('Ctrl Pts',(-7.27603390513785,-152.693984254242,
-4.20082013374671));
#30096=CARTESIAN_POINT('Ctrl Pts',(-9.70137854017371,-152.518984254242,
1.74701493417668E-11));
#30097=CARTESIAN_POINT('Ctrl Pts',(-7.27603390512272,-152.343984254242,
4.20082013377291));
#30098=CARTESIAN_POINT('Ctrl Pts',(-4.85068927007173,-152.168984254242,
8.40164026752836));
#30099=CARTESIAN_POINT('Ctrl Pts',(1.5129078685785E-11,-151.993984254242,
8.40164026751963));
#30100=CARTESIAN_POINT('Ctrl Pts',(4.85068927010198,-151.818984254242,8.40164026751089));
#30101=CARTESIAN_POINT('Ctrl Pts',(7.27603390513785,-151.643984254242,4.20082013374671));
#30102=CARTESIAN_POINT('Ctrl Pts',(9.70137854017371,-151.468984254242,-1.74689612655491E-11));
#30103=CARTESIAN_POINT('Ctrl Pts',(7.27603390512272,-151.293984254242,-4.20082013377291));
#30104=CARTESIAN_POINT('Ctrl Pts',(4.85068927007173,-151.118984254242,-8.40164026752836));
#30105=CARTESIAN_POINT('Ctrl Pts',(-1.51301075899711E-11,-150.943984254242,
-8.40164026751963));
#30106=CARTESIAN_POINT('Ctrl Pts',(-4.85068927010198,-150.768984254242,
-8.40164026751089));
#30107=CARTESIAN_POINT('Ctrl Pts',(-7.27603390513785,-150.593984254242,
-4.20082013374671));
#30108=CARTESIAN_POINT('Ctrl Pts',(-9.70137854017371,-150.418984254242,
1.74701493417668E-11));
#30109=CARTESIAN_POINT('Ctrl Pts',(-7.27603390512272,-150.243984254242,
4.20082013377291));
#30110=CARTESIAN_POINT('Ctrl Pts',(-4.85068927007173,-150.068984254242,
8.40164026752836));
#30111=CARTESIAN_POINT('Ctrl Pts',(1.5129078685785E-11,-149.893984254242,
8.40164026751963));
#30112=CARTESIAN_POINT('Ctrl Pts',(4.85068927010198,-149.718984254242,8.40164026751089));
#30113=CARTESIAN_POINT('Ctrl Pts',(7.27603390513785,-149.543984254242,4.20082013374671));
#30114=CARTESIAN_POINT('Ctrl Pts',(9.70137854017371,-149.368984254242,-1.74689612655491E-11));
#30115=CARTESIAN_POINT('Ctrl Pts',(7.27603390512272,-149.193984254242,-4.20082013377291));
#30116=CARTESIAN_POINT('Ctrl Pts',(4.85068927007173,-149.018984254242,-8.40164026752836));
#30117=CARTESIAN_POINT('Ctrl Pts',(-1.51301075899711E-11,-148.843984254242,
-8.40164026751963));
#30118=CARTESIAN_POINT('Ctrl Pts',(-4.85068927010198,-148.668984254242,
-8.40164026751089));
#30119=CARTESIAN_POINT('Ctrl Pts',(-7.27603390513785,-148.493984254242,
-4.20082013374671));
#30120=CARTESIAN_POINT('Ctrl Pts',(-9.70137854017371,-148.318984254242,
1.74701493417668E-11));
#30121=CARTESIAN_POINT('Ctrl Pts',(-7.27603390512272,-148.143984254242,
4.20082013377291));
#30122=CARTESIAN_POINT('Ctrl Pts',(-4.85068927007173,-147.968984254242,
8.40164026752836));
#30123=CARTESIAN_POINT('Ctrl Pts',(1.5129078685785E-11,-147.793984254242,
8.40164026751963));
#30124=CARTESIAN_POINT('Ctrl Pts',(4.85068927010198,-147.618984254242,8.40164026751089));
#30125=CARTESIAN_POINT('Ctrl Pts',(7.27603390513785,-147.443984254242,4.20082013374671));
#30126=CARTESIAN_POINT('Ctrl Pts',(9.70137854017371,-147.268984254242,-1.74689612655491E-11));
#30127=CARTESIAN_POINT('Ctrl Pts',(7.27603390512272,-147.093984254242,-4.20082013377291));
#30128=CARTESIAN_POINT('Ctrl Pts',(4.85068927007173,-146.918984254242,-8.40164026752836));
#30129=CARTESIAN_POINT('Ctrl Pts',(-1.51301075899711E-11,-146.743984254242,
-8.40164026751963));
#30130=CARTESIAN_POINT('Ctrl Pts',(-4.85068927010198,-146.568984254242,
-8.40164026751089));
#30131=CARTESIAN_POINT('Ctrl Pts',(-7.27603390513785,-146.393984254242,
-4.20082013374671));
#30132=CARTESIAN_POINT('Ctrl Pts',(-9.70137854017371,-146.218984254242,
1.74701493417668E-11));
#30133=CARTESIAN_POINT('Ctrl Pts',(-7.27603390512272,-146.043984254242,
4.20082013377291));
#30134=CARTESIAN_POINT('Ctrl Pts',(-4.85068927007173,-145.868984254242,
8.40164026752836));
#30135=CARTESIAN_POINT('Ctrl Pts',(1.5129078685785E-11,-145.693984254242,
8.40164026751963));
#30136=CARTESIAN_POINT('Ctrl Pts',(4.85068927010198,-145.518984254242,8.40164026751089));
#30137=CARTESIAN_POINT('Ctrl Pts',(7.27603390513785,-145.343984254242,4.20082013374671));
#30138=CARTESIAN_POINT('Ctrl Pts',(9.70137854017371,-145.168984254242,-1.74689612655491E-11));
#30139=CARTESIAN_POINT('Ctrl Pts',(7.27603390512272,-144.993984254242,-4.20082013377291));
#30140=CARTESIAN_POINT('Ctrl Pts',(4.85068927007173,-144.818984254242,-8.40164026752836));
#30141=CARTESIAN_POINT('Ctrl Pts',(-1.51301075899711E-11,-144.643984254242,
-8.40164026751963));
#30142=CARTESIAN_POINT('Ctrl Pts',(-4.85068927010198,-144.468984254242,
-8.40164026751089));
#30143=CARTESIAN_POINT('Ctrl Pts',(-7.27603390513785,-144.293984254242,
-4.20082013374671));
#30144=CARTESIAN_POINT('Ctrl Pts',(-9.70137854017371,-144.118984254242,
1.74701493417668E-11));
#30145=CARTESIAN_POINT('Ctrl Pts',(-7.27603390512272,-143.943984254242,
4.20082013377291));
#30146=CARTESIAN_POINT('Ctrl Pts',(-4.85068927007173,-143.768984254242,
8.40164026752836));
#30147=CARTESIAN_POINT('Ctrl Pts',(1.5129078685785E-11,-143.593984254242,
8.40164026751963));
#30148=CARTESIAN_POINT('Ctrl Pts',(4.85068927010198,-143.418984254242,8.40164026751089));
#30149=CARTESIAN_POINT('Ctrl Pts',(7.27603390513785,-143.243984254242,4.20082013374671));
#30150=CARTESIAN_POINT('Ctrl Pts',(9.70137854017371,-143.068984254242,-1.74689612655491E-11));
#30151=CARTESIAN_POINT('Ctrl Pts',(7.27603390512272,-142.893984254242,-4.20082013377291));
#30152=CARTESIAN_POINT('Ctrl Pts',(4.85068927007173,-142.718984254242,-8.40164026752836));
#30153=CARTESIAN_POINT('Ctrl Pts',(-1.51301075899711E-11,-142.543984254242,
-8.40164026751963));
#30154=CARTESIAN_POINT('Ctrl Pts',(-4.85068927010198,-142.368984254242,
-8.40164026751089));
#30155=CARTESIAN_POINT('Ctrl Pts',(-7.27603390513785,-142.193984254242,
-4.20082013374671));
#30156=CARTESIAN_POINT('Ctrl Pts',(-9.70137854017371,-142.018984254242,
1.74701493417668E-11));
#30157=CARTESIAN_POINT('Ctrl Pts',(-7.27603390512272,-141.843984254242,
4.20082013377291));
#30158=CARTESIAN_POINT('Ctrl Pts',(-4.85068927007173,-141.668984254242,
8.40164026752836));
#30159=CARTESIAN_POINT('Ctrl Pts',(1.5129078685785E-11,-141.493984254242,
8.40164026751963));
#30160=CARTESIAN_POINT('Ctrl Pts',(4.85068927010198,-141.318984254242,8.40164026751089));
#30161=CARTESIAN_POINT('Ctrl Pts',(7.27603390513785,-141.143984254242,4.20082013374671));
#30162=CARTESIAN_POINT('Ctrl Pts',(9.70137854017371,-140.968984254242,-1.74689612655491E-11));
#30163=CARTESIAN_POINT('Ctrl Pts',(7.27603390512272,-140.793984254242,-4.20082013377291));
#30164=CARTESIAN_POINT('Ctrl Pts',(4.85068927007173,-140.618984254242,-8.40164026752836));
#30165=CARTESIAN_POINT('Ctrl Pts',(-1.51301075899711E-11,-140.443984254242,
-8.40164026751963));
#30166=CARTESIAN_POINT('Ctrl Pts',(-4.85068927010198,-140.268984254242,
-8.40164026751089));
#30167=CARTESIAN_POINT('Ctrl Pts',(-7.27603390513785,-140.093984254242,
-4.20082013374671));
#30168=CARTESIAN_POINT('Ctrl Pts',(-9.70137854017371,-139.918984254242,
1.74701493417668E-11));
#30169=CARTESIAN_POINT('Ctrl Pts',(-7.27603390512272,-139.743984254242,
4.20082013377291));
#30170=CARTESIAN_POINT('Ctrl Pts',(-4.85068927007173,-139.568984254242,
8.40164026752836));
#30171=CARTESIAN_POINT('Ctrl Pts',(1.5129078685785E-11,-139.393984254242,
8.40164026751963));
#30172=CARTESIAN_POINT('Ctrl Pts',(4.85068927010198,-139.218984254242,8.40164026751089));
#30173=CARTESIAN_POINT('Ctrl Pts',(7.27603390513785,-139.043984254242,4.20082013374671));
#30174=CARTESIAN_POINT('Ctrl Pts',(9.70137854017371,-138.868984254242,-1.74689612655491E-11));
#30175=CARTESIAN_POINT('Ctrl Pts',(7.27603390512272,-138.693984254242,-4.20082013377291));
#30176=CARTESIAN_POINT('Ctrl Pts',(4.85068927007173,-138.518984254242,-8.40164026752836));
#30177=CARTESIAN_POINT('Ctrl Pts',(-1.51301075899711E-11,-138.343984254242,
-8.40164026751963));
#30178=CARTESIAN_POINT('Ctrl Pts',(-4.85068927010198,-138.168984254242,
-8.40164026751089));
#30179=CARTESIAN_POINT('Ctrl Pts',(-7.27603390513785,-137.993984254242,
-4.20082013374671));
#30180=CARTESIAN_POINT('Ctrl Pts',(-9.70137854017371,-137.818984254242,
1.74701493417668E-11));
#30181=CARTESIAN_POINT('Ctrl Pts',(-7.27603390512272,-137.643984254242,
4.20082013377291));
#30182=CARTESIAN_POINT('Ctrl Pts',(-4.85068927007173,-137.468984254242,
8.40164026752836));
#30183=CARTESIAN_POINT('Ctrl Pts',(1.5129078685785E-11,-137.293984254242,
8.40164026751963));
#30184=CARTESIAN_POINT('Ctrl Pts',(4.85068927010198,-137.118984254242,8.40164026751089));
#30185=CARTESIAN_POINT('Ctrl Pts',(7.27603390513785,-136.943984254242,4.20082013374671));
#30186=CARTESIAN_POINT('Ctrl Pts',(9.70137854017371,-136.768984254242,-1.74689612655491E-11));
#30187=CARTESIAN_POINT('Ctrl Pts',(7.27603390512272,-136.593984254242,-4.20082013377291));
#30188=CARTESIAN_POINT('Ctrl Pts',(4.85068927007173,-136.418984254242,-8.40164026752836));
#30189=CARTESIAN_POINT('Ctrl Pts',(-1.51301075899711E-11,-136.243984254242,
-8.40164026751963));
#30190=CARTESIAN_POINT('Ctrl Pts',(-4.85068927010198,-136.068984254242,
-8.40164026751089));
#30191=CARTESIAN_POINT('Ctrl Pts',(-7.27603390513785,-135.893984254242,
-4.20082013374671));
#30192=CARTESIAN_POINT('Ctrl Pts',(-9.70137854017371,-135.718984254242,
1.74701493417668E-11));
#30193=CARTESIAN_POINT('Ctrl Pts',(-7.27603390512272,-135.543984254242,
4.20082013377291));
#30194=CARTESIAN_POINT('Ctrl Pts',(-4.85068927007173,-135.368984254242,
8.40164026752836));
#30195=CARTESIAN_POINT('Ctrl Pts',(1.5129078685785E-11,-135.193984254242,
8.40164026751963));
#30196=CARTESIAN_POINT('Ctrl Pts',(4.85068927010198,-135.018984254242,8.40164026751089));
#30197=CARTESIAN_POINT('Ctrl Pts',(7.27603390513785,-134.843984254242,4.20082013374671));
#30198=CARTESIAN_POINT('Ctrl Pts',(9.70137854017371,-134.668984254242,-1.74689612655491E-11));
#30199=CARTESIAN_POINT('Ctrl Pts',(7.27603390512272,-134.493984254242,-4.20082013377291));
#30200=CARTESIAN_POINT('Ctrl Pts',(4.85068927007173,-134.318984254242,-8.40164026752836));
#30201=CARTESIAN_POINT('Ctrl Pts',(-1.51301075899711E-11,-134.143984254242,
-8.40164026751963));
#30202=CARTESIAN_POINT('Ctrl Pts',(-4.85068927010198,-133.968984254242,
-8.40164026751089));
#30203=CARTESIAN_POINT('Ctrl Pts',(-7.27603390513785,-133.793984254242,
-4.20082013374671));
#30204=CARTESIAN_POINT('Ctrl Pts',(-9.70137854017371,-133.618984254242,
1.74701493417668E-11));
#30205=CARTESIAN_POINT('Ctrl Pts',(-7.27603390512272,-133.443984254242,
4.20082013377291));
#30206=CARTESIAN_POINT('Ctrl Pts',(-4.85068927007173,-133.268984254242,
8.40164026752836));
#30207=CARTESIAN_POINT('Ctrl Pts',(1.5129078685785E-11,-133.093984254242,
8.40164026751963));
#30208=CARTESIAN_POINT('Ctrl Pts',(4.85068927010198,-132.918984254242,8.40164026751089));
#30209=CARTESIAN_POINT('Ctrl Pts',(7.27603390513785,-132.743984254242,4.20082013374671));
#30210=CARTESIAN_POINT('Ctrl Pts',(9.70137854017371,-132.568984254242,-1.74689612655491E-11));
#30211=CARTESIAN_POINT('Ctrl Pts',(7.27603390512272,-132.393984254242,-4.20082013377291));
#30212=CARTESIAN_POINT('Ctrl Pts',(4.85068927007173,-132.218984254242,-8.40164026752836));
#30213=CARTESIAN_POINT('Ctrl Pts',(-1.51301075899711E-11,-132.043984254242,
-8.40164026751963));
#30214=CARTESIAN_POINT('Ctrl Pts',(-4.85068927010198,-131.868984254242,
-8.40164026751089));
#30215=CARTESIAN_POINT('Ctrl Pts',(-7.27603390513785,-131.693984254242,
-4.20082013374671));
#30216=CARTESIAN_POINT('Ctrl Pts',(-9.70137854017371,-131.518984254242,
1.74701493417668E-11));
#30217=CARTESIAN_POINT('Ctrl Pts',(-7.27603390512272,-131.343984254242,
4.20082013377291));
#30218=CARTESIAN_POINT('Ctrl Pts',(-4.85068927007173,-131.168984254242,
8.40164026752836));
#30219=CARTESIAN_POINT('Ctrl Pts',(1.5129078685785E-11,-130.993984254242,
8.40164026751963));
#30220=CARTESIAN_POINT('Ctrl Pts',(4.85068927010198,-130.818984254242,8.40164026751089));
#30221=CARTESIAN_POINT('Ctrl Pts',(7.27603390513785,-130.643984254242,4.20082013374671));
#30222=CARTESIAN_POINT('Ctrl Pts',(9.70137854017371,-130.468984254242,-1.74689612655491E-11));
#30223=CARTESIAN_POINT('Ctrl Pts',(7.27603390512272,-130.293984254242,-4.20082013377291));
#30224=CARTESIAN_POINT('Ctrl Pts',(4.85068927007173,-130.118984254242,-8.40164026752836));
#30225=CARTESIAN_POINT('Ctrl Pts',(-1.51301075899711E-11,-129.943984254242,
-8.40164026751963));
#30226=CARTESIAN_POINT('Ctrl Pts',(-4.85068927010198,-129.768984254242,
-8.40164026751089));
#30227=CARTESIAN_POINT('Ctrl Pts',(-7.27603390513785,-129.593984254242,
-4.20082013374671));
#30228=CARTESIAN_POINT('Ctrl Pts',(-9.70137854017371,-129.418984254242,
1.74701493417668E-11));
#30229=CARTESIAN_POINT('Ctrl Pts',(-7.27603390512272,-129.243984254242,
4.20082013377291));
#30230=CARTESIAN_POINT('Ctrl Pts',(-4.85068927007173,-129.068984254242,
8.40164026752836));
#30231=CARTESIAN_POINT('Ctrl Pts',(1.5129078685785E-11,-128.893984254242,
8.40164026751963));
#30232=CARTESIAN_POINT('Ctrl Pts',(4.85068927010198,-128.718984254242,8.40164026751089));
#30233=CARTESIAN_POINT('Ctrl Pts',(7.27603390513785,-128.543984254242,4.20082013374671));
#30234=CARTESIAN_POINT('Ctrl Pts',(9.70137854017371,-128.368984254242,-1.74689612655491E-11));
#30235=CARTESIAN_POINT('Ctrl Pts',(7.27603390512272,-128.193984254242,-4.20082013377291));
#30236=CARTESIAN_POINT('Ctrl Pts',(4.85068927007173,-128.018984254242,-8.40164026752836));
#30237=CARTESIAN_POINT('Ctrl Pts',(-1.51301075899711E-11,-127.843984254242,
-8.40164026751963));
#30238=CARTESIAN_POINT('Ctrl Pts',(-4.85068927010198,-127.668984254242,
-8.40164026751089));
#30239=CARTESIAN_POINT('Ctrl Pts',(-7.27603390513785,-127.493984254242,
-4.20082013374671));
#30240=CARTESIAN_POINT('Ctrl Pts',(-9.70137854017371,-127.318984254242,
1.74701493417668E-11));
#30241=CARTESIAN_POINT('Ctrl Pts',(-7.27603390512272,-127.143984254242,
4.20082013377291));
#30242=CARTESIAN_POINT('Ctrl Pts',(-4.85068927007173,-126.968984254242,
8.40164026752836));
#30243=CARTESIAN_POINT('Ctrl Pts',(1.5129078685785E-11,-126.793984254242,
8.40164026751963));
#30244=CARTESIAN_POINT('Ctrl Pts',(4.85068927010198,-126.618984254242,8.40164026751089));
#30245=CARTESIAN_POINT('Ctrl Pts',(7.27603390513785,-126.443984254242,4.20082013374671));
#30246=CARTESIAN_POINT('Ctrl Pts',(9.70137854017371,-126.268984254242,-1.74689612655491E-11));
#30247=CARTESIAN_POINT('Ctrl Pts',(7.27603390512272,-126.093984254242,-4.20082013377291));
#30248=CARTESIAN_POINT('Ctrl Pts',(4.85068927007173,-125.918984254242,-8.40164026752836));
#30249=CARTESIAN_POINT('Ctrl Pts',(-1.51301075899711E-11,-125.743984254242,
-8.40164026751963));
#30250=CARTESIAN_POINT('Ctrl Pts',(-4.85068927010198,-125.568984254242,
-8.40164026751089));
#30251=CARTESIAN_POINT('Ctrl Pts',(-7.27603390513785,-125.393984254242,
-4.20082013374671));
#30252=CARTESIAN_POINT('Ctrl Pts',(-9.70137854017371,-125.218984254242,
1.74701493417668E-11));
#30253=CARTESIAN_POINT('Ctrl Pts',(-7.27603390512272,-125.043984254242,
4.20082013377291));
#30254=CARTESIAN_POINT('Ctrl Pts',(-4.85068927007173,-124.868984254242,
8.40164026752836));
#30255=CARTESIAN_POINT('Ctrl Pts',(1.5129078685785E-11,-124.693984254242,
8.40164026751963));
#30256=CARTESIAN_POINT('Ctrl Pts',(4.85068927010198,-124.518984254242,8.40164026751089));
#30257=CARTESIAN_POINT('Ctrl Pts',(7.27603390513785,-124.343984254242,4.20082013374671));
#30258=CARTESIAN_POINT('Ctrl Pts',(9.70137854017371,-124.168984254242,-1.74689612655491E-11));
#30259=CARTESIAN_POINT('Ctrl Pts',(7.27603390512272,-123.993984254242,-4.20082013377291));
#30260=CARTESIAN_POINT('Ctrl Pts',(4.85068927007173,-123.818984254242,-8.40164026752836));
#30261=CARTESIAN_POINT('Ctrl Pts',(-1.51301075899711E-11,-123.643984254242,
-8.40164026751963));
#30262=CARTESIAN_POINT('Ctrl Pts',(-4.85068927010198,-123.468984254242,
-8.40164026751089));
#30263=CARTESIAN_POINT('Ctrl Pts',(-7.27603390513785,-123.293984254242,
-4.20082013374671));
#30264=CARTESIAN_POINT('Ctrl Pts',(-9.70137854017371,-123.118984254242,
1.74701493417668E-11));
#30265=CARTESIAN_POINT('Ctrl Pts',(-7.27603390512272,-122.943984254242,
4.20082013377291));
#30266=CARTESIAN_POINT('Ctrl Pts',(-4.85068927007173,-122.768984254242,
8.40164026752836));
#30267=CARTESIAN_POINT('Ctrl Pts',(1.5129078685785E-11,-122.593984254242,
8.40164026751963));
#30268=CARTESIAN_POINT('Ctrl Pts',(4.85068927010198,-122.418984254242,8.40164026751089));
#30269=CARTESIAN_POINT('Ctrl Pts',(7.27603390513785,-122.243984254242,4.20082013374671));
#30270=CARTESIAN_POINT('Ctrl Pts',(9.70137854017371,-122.068984254242,-1.74689612655491E-11));
#30271=CARTESIAN_POINT('Ctrl Pts',(7.27603390512272,-121.893984254242,-4.20082013377291));
#30272=CARTESIAN_POINT('Ctrl Pts',(4.85068927007173,-121.718984254242,-8.40164026752836));
#30273=CARTESIAN_POINT('Ctrl Pts',(-1.51301075899711E-11,-121.543984254242,
-8.40164026751963));
#30274=CARTESIAN_POINT('Ctrl Pts',(-4.85068927010198,-121.368984254242,
-8.40164026751089));
#30275=CARTESIAN_POINT('Ctrl Pts',(-7.27603390513785,-121.193984254242,
-4.20082013374671));
#30276=CARTESIAN_POINT('Ctrl Pts',(-9.70137854017371,-121.018984254242,
1.74701493417668E-11));
#30277=CARTESIAN_POINT('Ctrl Pts',(-7.27603390512272,-120.843984254242,
4.20082013377291));
#30278=CARTESIAN_POINT('Ctrl Pts',(-4.85068927007173,-120.668984254242,
8.40164026752836));
#30279=CARTESIAN_POINT('Ctrl Pts',(1.5129078685785E-11,-120.493984254242,
8.40164026751963));
#30280=CARTESIAN_POINT('Ctrl Pts',(4.85068927010198,-120.318984254242,8.40164026751089));
#30281=CARTESIAN_POINT('Ctrl Pts',(7.27603390513785,-120.143984254242,4.20082013374671));
#30282=CARTESIAN_POINT('Ctrl Pts',(9.70137854017371,-119.968984254242,-1.74689612655491E-11));
#30283=CARTESIAN_POINT('Ctrl Pts',(7.27603390512272,-119.793984254242,-4.20082013377291));
#30284=CARTESIAN_POINT('Ctrl Pts',(4.85068927007173,-119.618984254242,-8.40164026752836));
#30285=CARTESIAN_POINT('Ctrl Pts',(-1.51301075899711E-11,-119.443984254242,
-8.40164026751963));
#30286=CARTESIAN_POINT('Ctrl Pts',(-4.85068927010198,-119.268984254242,
-8.40164026751089));
#30287=CARTESIAN_POINT('Ctrl Pts',(-7.27603390513785,-119.093984254242,
-4.20082013374671));
#30288=CARTESIAN_POINT('Ctrl Pts',(-9.70137854017371,-118.918984254242,
1.74701493417668E-11));
#30289=CARTESIAN_POINT('Ctrl Pts',(-7.27603390512272,-118.743984254242,
4.20082013377291));
#30290=CARTESIAN_POINT('Ctrl Pts',(-4.85068927007173,-118.568984254242,
8.40164026752836));
#30291=CARTESIAN_POINT('Ctrl Pts',(1.5129078685785E-11,-118.393984254242,
8.40164026751963));
#30292=CARTESIAN_POINT('Ctrl Pts',(4.85068927010198,-118.218984254242,8.40164026751089));
#30293=CARTESIAN_POINT('Ctrl Pts',(7.27603390513785,-118.043984254242,4.20082013374671));
#30294=CARTESIAN_POINT('Ctrl Pts',(9.70137854017371,-117.868984254242,-1.74689612655491E-11));
#30295=CARTESIAN_POINT('Ctrl Pts',(7.27603390512272,-117.693984254242,-4.20082013377291));
#30296=CARTESIAN_POINT('Ctrl Pts',(4.85068927007173,-117.518984254242,-8.40164026752836));
#30297=CARTESIAN_POINT('Ctrl Pts',(-1.51301075899711E-11,-117.343984254242,
-8.40164026751963));
#30298=CARTESIAN_POINT('Ctrl Pts',(-4.85068927010198,-117.168984254242,
-8.40164026751089));
#30299=CARTESIAN_POINT('Ctrl Pts',(-7.27603390513785,-116.993984254242,
-4.20082013374671));
#30300=CARTESIAN_POINT('Ctrl Pts',(-9.70137854017371,-116.818984254242,
1.74701493417668E-11));
#30301=CARTESIAN_POINT('Ctrl Pts',(-7.27603390512272,-116.643984254242,
4.20082013377291));
#30302=CARTESIAN_POINT('Ctrl Pts',(-4.85068927007173,-116.468984254242,
8.40164026752836));
#30303=CARTESIAN_POINT('Ctrl Pts',(1.5129078685785E-11,-116.293984254242,
8.40164026751963));
#30304=CARTESIAN_POINT('Ctrl Pts',(4.85068927010198,-116.118984254242,8.40164026751089));
#30305=CARTESIAN_POINT('Ctrl Pts',(7.27603390513785,-115.943984254242,4.20082013374671));
#30306=CARTESIAN_POINT('Ctrl Pts',(9.70137854017371,-115.768984254242,-1.74689612655491E-11));
#30307=CARTESIAN_POINT('Ctrl Pts',(7.27603390512272,-115.593984254242,-4.20082013377291));
#30308=CARTESIAN_POINT('Ctrl Pts',(4.85068927007173,-115.418984254242,-8.40164026752836));
#30309=CARTESIAN_POINT('Ctrl Pts',(-1.51301075899711E-11,-115.243984254242,
-8.40164026751963));
#30310=CARTESIAN_POINT('Ctrl Pts',(-4.85068927010198,-115.068984254242,
-8.40164026751089));
#30311=CARTESIAN_POINT('Ctrl Pts',(-7.27603390513785,-114.893984254242,
-4.20082013374671));
#30312=CARTESIAN_POINT('Ctrl Pts',(-9.70137854017371,-114.718984254242,
1.74701493417668E-11));
#30313=CARTESIAN_POINT('Ctrl Pts',(-7.27603390512272,-114.543984254242,
4.20082013377291));
#30314=CARTESIAN_POINT('Ctrl Pts',(-4.85068927007173,-114.368984254242,
8.40164026752836));
#30315=CARTESIAN_POINT('Ctrl Pts',(1.5129078685785E-11,-114.193984254242,
8.40164026751963));
#30316=CARTESIAN_POINT('Ctrl Pts',(4.85068927010198,-114.018984254242,8.40164026751089));
#30317=CARTESIAN_POINT('Ctrl Pts',(7.27603390513785,-113.843984254242,4.20082013374671));
#30318=CARTESIAN_POINT('Ctrl Pts',(9.70137854017371,-113.668984254242,-1.74689612655491E-11));
#30319=CARTESIAN_POINT('Ctrl Pts',(7.27603390512272,-113.493984254242,-4.20082013377291));
#30320=CARTESIAN_POINT('Ctrl Pts',(4.85068927007173,-113.318984254242,-8.40164026752836));
#30321=CARTESIAN_POINT('Ctrl Pts',(-1.51301075899711E-11,-113.143984254242,
-8.40164026751963));
#30322=CARTESIAN_POINT('Ctrl Pts',(-4.85068927010198,-112.968984254242,
-8.40164026751089));
#30323=CARTESIAN_POINT('Ctrl Pts',(-7.27603390513785,-112.793984254242,
-4.20082013374671));
#30324=CARTESIAN_POINT('Ctrl Pts',(-9.70137854017371,-112.618984254242,
1.74701493417668E-11));
#30325=CARTESIAN_POINT('Ctrl Pts',(-7.27603390512272,-112.443984254242,
4.20082013377291));
#30326=CARTESIAN_POINT('Ctrl Pts',(-4.85068927007173,-112.268984254242,
8.40164026752836));
#30327=CARTESIAN_POINT('Ctrl Pts',(1.5129078685785E-11,-112.093984254242,
8.40164026751963));
#30328=CARTESIAN_POINT('Ctrl Pts',(4.85068927010198,-111.918984254242,8.40164026751089));
#30329=CARTESIAN_POINT('Ctrl Pts',(7.27603390513785,-111.743984254242,4.20082013374671));
#30330=CARTESIAN_POINT('Ctrl Pts',(9.70137854017371,-111.568984254242,-1.74689612655491E-11));
#30331=CARTESIAN_POINT('Ctrl Pts',(7.27603390512272,-111.393984254242,-4.20082013377291));
#30332=CARTESIAN_POINT('Ctrl Pts',(4.85068927007173,-111.218984254242,-8.40164026752836));
#30333=CARTESIAN_POINT('Ctrl Pts',(-1.51301075899711E-11,-111.043984254242,
-8.40164026751963));
#30334=CARTESIAN_POINT('Ctrl Pts',(-4.85068927010198,-110.868984254242,
-8.40164026751089));
#30335=CARTESIAN_POINT('Ctrl Pts',(-7.27603390513785,-110.693984254242,
-4.20082013374671));
#30336=CARTESIAN_POINT('Ctrl Pts',(-9.70137854017371,-110.518984254242,
1.74701493417668E-11));
#30337=CARTESIAN_POINT('Ctrl Pts',(-7.27603390512272,-110.343984254242,
4.20082013377291));
#30338=CARTESIAN_POINT('Ctrl Pts',(-4.85068927007173,-110.168984254242,
8.40164026752836));
#30339=CARTESIAN_POINT('Ctrl Pts',(1.5129078685785E-11,-109.993984254242,
8.40164026751963));
#30340=CARTESIAN_POINT('Ctrl Pts',(4.85068927010198,-109.818984254242,8.40164026751089));
#30341=CARTESIAN_POINT('Ctrl Pts',(7.27603390513785,-109.643984254242,4.20082013374671));
#30342=CARTESIAN_POINT('Ctrl Pts',(9.70137854017371,-109.468984254242,-1.74689612655491E-11));
#30343=CARTESIAN_POINT('Ctrl Pts',(7.27603390512272,-109.293984254242,-4.20082013377291));
#30344=CARTESIAN_POINT('Ctrl Pts',(4.85068927007173,-109.118984254242,-8.40164026752836));
#30345=CARTESIAN_POINT('Ctrl Pts',(-1.51301075899711E-11,-108.943984254242,
-8.40164026751963));
#30346=CARTESIAN_POINT('Ctrl Pts',(-4.85068927010198,-108.768984254242,
-8.40164026751089));
#30347=CARTESIAN_POINT('Ctrl Pts',(-7.27603390513785,-108.593984254242,
-4.20082013374671));
#30348=CARTESIAN_POINT('Ctrl Pts',(-9.70137854017371,-108.418984254242,
1.74701493417668E-11));
#30349=CARTESIAN_POINT('Ctrl Pts',(-7.27603390512272,-108.243984254242,
4.20082013377291));
#30350=CARTESIAN_POINT('Ctrl Pts',(-4.85068927007173,-108.068984254242,
8.40164026752836));
#30351=CARTESIAN_POINT('Ctrl Pts',(1.5129078685785E-11,-107.893984254242,
8.40164026751963));
#30352=CARTESIAN_POINT('Ctrl Pts',(4.85068927010198,-107.718984254242,8.40164026751089));
#30353=CARTESIAN_POINT('Ctrl Pts',(7.27603390513785,-107.543984254242,4.20082013374671));
#30354=CARTESIAN_POINT('Ctrl Pts',(9.70137854017371,-107.368984254242,-1.74689612655491E-11));
#30355=CARTESIAN_POINT('Ctrl Pts',(7.27603390512272,-107.193984254242,-4.20082013377291));
#30356=CARTESIAN_POINT('Ctrl Pts',(4.85068927007173,-107.018984254242,-8.40164026752836));
#30357=CARTESIAN_POINT('Ctrl Pts',(-1.51301075899711E-11,-106.843984254242,
-8.40164026751963));
#30358=CARTESIAN_POINT('Ctrl Pts',(-4.85068927010198,-106.668984254242,
-8.40164026751089));
#30359=CARTESIAN_POINT('Ctrl Pts',(-7.27603390513785,-106.493984254242,
-4.20082013374671));
#30360=CARTESIAN_POINT('Ctrl Pts',(-9.70137854017371,-106.318984254242,
1.74701493417668E-11));
#30361=CARTESIAN_POINT('Ctrl Pts',(-7.27603390512272,-106.143984254242,
4.20082013377291));
#30362=CARTESIAN_POINT('Ctrl Pts',(-4.85068927007173,-105.968984254242,
8.40164026752836));
#30363=CARTESIAN_POINT('Ctrl Pts',(1.5129078685785E-11,-105.793984254242,
8.40164026751963));
#30364=CARTESIAN_POINT('Ctrl Pts',(4.85068927010198,-105.618984254242,8.40164026751089));
#30365=CARTESIAN_POINT('Ctrl Pts',(7.27603390513785,-105.443984254242,4.20082013374671));
#30366=CARTESIAN_POINT('Ctrl Pts',(9.70137854017371,-105.268984254242,-1.74689612655491E-11));
#30367=CARTESIAN_POINT('Ctrl Pts',(7.27603390512272,-105.093984254242,-4.20082013377291));
#30368=CARTESIAN_POINT('Ctrl Pts',(4.85068927007173,-104.918984254242,-8.40164026752836));
#30369=CARTESIAN_POINT('Ctrl Pts',(-1.51301075899711E-11,-104.743984254242,
-8.40164026751963));
#30370=CARTESIAN_POINT('Ctrl Pts',(-4.85068927010198,-104.568984254242,
-8.40164026751089));
#30371=CARTESIAN_POINT('Ctrl Pts',(-7.27603390513785,-104.393984254242,
-4.20082013374671));
#30372=CARTESIAN_POINT('Ctrl Pts',(-9.70137854017371,-104.218984254242,
1.74701493417668E-11));
#30373=CARTESIAN_POINT('Ctrl Pts',(-7.27603390512272,-104.043984254242,
4.20082013377291));
#30374=CARTESIAN_POINT('Ctrl Pts',(-4.85068927007173,-103.868984254242,
8.40164026752836));
#30375=CARTESIAN_POINT('Ctrl Pts',(1.5129078685785E-11,-103.693984254242,
8.40164026751963));
#30376=CARTESIAN_POINT('Ctrl Pts',(4.85068927010198,-103.518984254242,8.40164026751089));
#30377=CARTESIAN_POINT('Ctrl Pts',(7.27603390513785,-103.343984254242,4.20082013374671));
#30378=CARTESIAN_POINT('Ctrl Pts',(9.70137854017371,-103.168984254242,-1.74689612655491E-11));
#30379=CARTESIAN_POINT('Ctrl Pts',(7.27603390512272,-102.993984254242,-4.20082013377291));
#30380=CARTESIAN_POINT('Ctrl Pts',(4.85068927007173,-102.818984254242,-8.40164026752836));
#30381=CARTESIAN_POINT('Ctrl Pts',(-1.51301075899711E-11,-102.643984254242,
-8.40164026751963));
#30382=CARTESIAN_POINT('Ctrl Pts',(-4.85068927010198,-102.468984254242,
-8.40164026751089));
#30383=CARTESIAN_POINT('Ctrl Pts',(-7.27603390513785,-102.293984254242,
-4.20082013374671));
#30384=CARTESIAN_POINT('Ctrl Pts',(-9.70137854017371,-102.118984254242,
1.74701493417668E-11));
#30385=CARTESIAN_POINT('Ctrl Pts',(-7.27603390512272,-101.943984254242,
4.20082013377291));
#30386=CARTESIAN_POINT('Ctrl Pts',(-4.85068927007173,-101.768984254242,
8.40164026752836));
#30387=CARTESIAN_POINT('Ctrl Pts',(1.5129078685785E-11,-101.593984254242,
8.40164026751963));
#30388=CARTESIAN_POINT('Ctrl Pts',(4.85068927010198,-101.418984254242,8.40164026751089));
#30389=CARTESIAN_POINT('Ctrl Pts',(7.27603390513785,-101.243984254242,4.20082013374671));
#30390=CARTESIAN_POINT('Ctrl Pts',(9.70137854017371,-101.068984254242,-1.74689612655491E-11));
#30391=CARTESIAN_POINT('Ctrl Pts',(7.27603390512272,-100.893984254242,-4.20082013377291));
#30392=CARTESIAN_POINT('Ctrl Pts',(4.85068927007173,-100.718984254242,-8.40164026752836));
#30393=CARTESIAN_POINT('Ctrl Pts',(-1.51301075899711E-11,-100.543984254242,
-8.40164026751963));
#30394=CARTESIAN_POINT('Ctrl Pts',(-4.85068927010198,-100.368984254242,
-8.40164026751089));
#30395=CARTESIAN_POINT('Ctrl Pts',(-7.27603390513785,-100.193984254242,
-4.20082013374671));
#30396=CARTESIAN_POINT('Ctrl Pts',(-9.70137854017371,-100.018984254242,
1.74701493417668E-11));
#30397=CARTESIAN_POINT('Ctrl Pts',(-7.27603390512272,-99.8439842542419,
4.20082013377291));
#30398=CARTESIAN_POINT('Ctrl Pts',(-4.85068927007173,-99.6689842542419,
8.40164026752836));
#30399=CARTESIAN_POINT('Ctrl Pts',(1.5129078685785E-11,-99.4939842542419,
8.40164026751963));
#30400=CARTESIAN_POINT('Ctrl Pts',(4.85068927010198,-99.3189842542419,8.40164026751089));
#30401=CARTESIAN_POINT('Ctrl Pts',(7.27603390513785,-99.1439842542419,4.20082013374671));
#30402=CARTESIAN_POINT('Ctrl Pts',(9.70137854017371,-98.9689842542419,-1.74689612655491E-11));
#30403=CARTESIAN_POINT('Ctrl Pts',(7.27603390512272,-98.7939842542419,-4.20082013377291));
#30404=CARTESIAN_POINT('Ctrl Pts',(4.85068927007173,-98.6189842542419,-8.40164026752836));
#30405=CARTESIAN_POINT('Ctrl Pts',(-1.51301075899711E-11,-98.4439842542419,
-8.40164026751963));
#30406=CARTESIAN_POINT('Ctrl Pts',(-4.85068927010198,-98.2689842542419,
-8.40164026751089));
#30407=CARTESIAN_POINT('Ctrl Pts',(-7.27603390513785,-98.0939842542419,
-4.20082013374671));
#30408=CARTESIAN_POINT('Ctrl Pts',(-9.70137854017371,-97.9189842542419,
1.74701493417668E-11));
#30409=CARTESIAN_POINT('Ctrl Pts',(-7.27603390512272,-97.7439842542419,
4.20082013377291));
#30410=CARTESIAN_POINT('Ctrl Pts',(-4.85068927007173,-97.5689842542419,
8.40164026752836));
#30411=CARTESIAN_POINT('Ctrl Pts',(1.5129078685785E-11,-97.3939842542419,
8.40164026751963));
#30412=CARTESIAN_POINT('Ctrl Pts',(4.85068927010198,-97.2189842542419,8.40164026751089));
#30413=CARTESIAN_POINT('Ctrl Pts',(7.27603390513785,-97.0439842542419,4.20082013374671));
#30414=CARTESIAN_POINT('Ctrl Pts',(9.70137854017371,-96.8689842542419,-1.74689612655491E-11));
#30415=CARTESIAN_POINT('Ctrl Pts',(7.27603390512272,-96.6939842542419,-4.20082013377291));
#30416=CARTESIAN_POINT('Ctrl Pts',(4.85068927007173,-96.5189842542419,-8.40164026752836));
#30417=CARTESIAN_POINT('Ctrl Pts',(-1.51301075899711E-11,-96.3439842542419,
-8.40164026751963));
#30418=CARTESIAN_POINT('Ctrl Pts',(-4.85068927010198,-96.1689842542419,
-8.40164026751089));
#30419=CARTESIAN_POINT('Ctrl Pts',(-7.27603390513785,-95.9939842542419,
-4.20082013374671));
#30420=CARTESIAN_POINT('Ctrl Pts',(-9.70137854017371,-95.8189842542419,
1.74701493417668E-11));
#30421=CARTESIAN_POINT('Ctrl Pts',(-7.27603390512272,-95.6439842542419,
4.20082013377291));
#30422=CARTESIAN_POINT('Ctrl Pts',(-4.85068927007173,-95.4689842542419,
8.40164026752836));
#30423=CARTESIAN_POINT('Ctrl Pts',(1.5129078685785E-11,-95.2939842542419,
8.40164026751963));
#30424=CARTESIAN_POINT('Ctrl Pts',(4.85068927010198,-95.1189842542419,8.40164026751089));
#30425=CARTESIAN_POINT('Ctrl Pts',(7.27603390513785,-94.9439842542419,4.20082013374671));
#30426=CARTESIAN_POINT('Ctrl Pts',(9.70137854017371,-94.7689842542419,-1.74689612655491E-11));
#30427=CARTESIAN_POINT('Ctrl Pts',(7.27603390512272,-94.5939842542419,-4.20082013377291));
#30428=CARTESIAN_POINT('Ctrl Pts',(4.85068927007173,-94.4189842542419,-8.40164026752836));
#30429=CARTESIAN_POINT('Ctrl Pts',(-1.51301075899711E-11,-94.2439842542419,
-8.40164026751963));
#30430=CARTESIAN_POINT('Ctrl Pts',(-4.85068927010198,-94.0689842542419,
-8.40164026751089));
#30431=CARTESIAN_POINT('Ctrl Pts',(-7.27603390513785,-93.8939842542419,
-4.20082013374671));
#30432=CARTESIAN_POINT('Ctrl Pts',(-9.70137854017371,-93.7189842542419,
1.74701493417668E-11));
#30433=CARTESIAN_POINT('Ctrl Pts',(-7.27603390512272,-93.5439842542419,
4.20082013377291));
#30434=CARTESIAN_POINT('Ctrl Pts',(-4.85068927007173,-93.3689842542419,
8.40164026752836));
#30435=CARTESIAN_POINT('Ctrl Pts',(1.5129078685785E-11,-93.1939842542419,
8.40164026751963));
#30436=CARTESIAN_POINT('Ctrl Pts',(4.85068927010198,-93.0189842542419,8.40164026751089));
#30437=CARTESIAN_POINT('Ctrl Pts',(7.27603390513785,-92.8439842542419,4.20082013374671));
#30438=CARTESIAN_POINT('Ctrl Pts',(9.70137854017371,-92.6689842542419,-1.74689612655491E-11));
#30439=CARTESIAN_POINT('Ctrl Pts',(7.27603390512272,-92.4939842542419,-4.20082013377291));
#30440=CARTESIAN_POINT('Ctrl Pts',(4.85068927007173,-92.3189842542419,-8.40164026752836));
#30441=CARTESIAN_POINT('Ctrl Pts',(-1.51301075899711E-11,-92.1439842542419,
-8.40164026751963));
#30442=CARTESIAN_POINT('Ctrl Pts',(-4.85068927010198,-91.9689842542419,
-8.40164026751089));
#30443=CARTESIAN_POINT('Ctrl Pts',(-7.27603390513785,-91.7939842542419,
-4.20082013374671));
#30444=CARTESIAN_POINT('Ctrl Pts',(-9.70137854017371,-91.6189842542419,
1.74701493417668E-11));
#30445=CARTESIAN_POINT('Ctrl Pts',(-7.27603390512272,-91.4439842542419,
4.20082013377291));
#30446=CARTESIAN_POINT('Ctrl Pts',(-4.85068927007173,-91.2689842542419,
8.40164026752836));
#30447=CARTESIAN_POINT('Ctrl Pts',(1.5129078685785E-11,-91.0939842542419,
8.40164026751963));
#30448=CARTESIAN_POINT('Ctrl Pts',(4.85068927010198,-90.9189842542419,8.40164026751089));
#30449=CARTESIAN_POINT('Ctrl Pts',(7.27603390513785,-90.7439842542419,4.20082013374671));
#30450=CARTESIAN_POINT('Ctrl Pts',(9.70137854017371,-90.5689842542419,-1.74689612655491E-11));
#30451=CARTESIAN_POINT('Ctrl Pts',(7.27603390512272,-90.3939842542419,-4.20082013377291));
#30452=CARTESIAN_POINT('Ctrl Pts',(4.85068927007173,-90.2189842542419,-8.40164026752836));
#30453=CARTESIAN_POINT('Ctrl Pts',(-1.51301075899711E-11,-90.0439842542419,
-8.40164026751963));
#30454=CARTESIAN_POINT('Ctrl Pts',(-4.85068927010198,-89.8689842542419,
-8.40164026751089));
#30455=CARTESIAN_POINT('Ctrl Pts',(-7.27603390513785,-89.6939842542419,
-4.20082013374671));
#30456=CARTESIAN_POINT('Ctrl Pts',(-9.70137854017371,-89.5189842542419,
1.74701493417668E-11));
#30457=CARTESIAN_POINT('Ctrl Pts',(-7.27603390512272,-89.3439842542419,
4.20082013377291));
#30458=CARTESIAN_POINT('Ctrl Pts',(-4.85068927007173,-89.1689842542419,
8.40164026752836));
#30459=CARTESIAN_POINT('Ctrl Pts',(1.5129078685785E-11,-88.9939842542419,
8.40164026751963));
#30460=CARTESIAN_POINT('Ctrl Pts',(4.85068927010198,-88.8189842542419,8.40164026751089));
#30461=CARTESIAN_POINT('Ctrl Pts',(7.27603390513785,-88.6439842542419,4.20082013374671));
#30462=CARTESIAN_POINT('Ctrl Pts',(9.70137854017371,-88.4689842542419,-1.74689612655491E-11));
#30463=CARTESIAN_POINT('Ctrl Pts',(7.27603390512272,-88.2939842542419,-4.20082013377291));
#30464=CARTESIAN_POINT('Ctrl Pts',(4.85068927007173,-88.1189842542419,-8.40164026752836));
#30465=CARTESIAN_POINT('Ctrl Pts',(-1.51301075899711E-11,-87.9439842542419,
-8.40164026751963));
#30466=CARTESIAN_POINT('Ctrl Pts',(-4.85068927010198,-87.7689842542419,
-8.40164026751089));
#30467=CARTESIAN_POINT('Ctrl Pts',(-7.27603390513785,-87.5939842542419,
-4.20082013374671));
#30468=CARTESIAN_POINT('Ctrl Pts',(-9.70137854017371,-87.4189842542419,
1.74701493417668E-11));
#30469=CARTESIAN_POINT('Ctrl Pts',(-7.27603390512272,-87.2439842542419,
4.20082013377291));
#30470=CARTESIAN_POINT('Ctrl Pts',(-4.85068927007173,-87.0689842542419,
8.40164026752836));
#30471=CARTESIAN_POINT('Ctrl Pts',(1.5129078685785E-11,-86.8939842542419,
8.40164026751963));
#30472=CARTESIAN_POINT('Ctrl Pts',(4.85068927010198,-86.7189842542419,8.40164026751089));
#30473=CARTESIAN_POINT('Ctrl Pts',(7.27603390513785,-86.5439842542419,4.20082013374671));
#30474=CARTESIAN_POINT('Ctrl Pts',(9.70137854017371,-86.3689842542419,-1.74689612655491E-11));
#30475=CARTESIAN_POINT('Ctrl Pts',(7.27603390512272,-86.1939842542419,-4.20082013377291));
#30476=CARTESIAN_POINT('Ctrl Pts',(4.85068927007173,-86.0189842542419,-8.40164026752836));
#30477=CARTESIAN_POINT('Ctrl Pts',(-1.51301075899711E-11,-85.8439842542419,
-8.40164026751963));
#30478=CARTESIAN_POINT('Ctrl Pts',(-4.85068927010198,-85.6689842542419,
-8.40164026751089));
#30479=CARTESIAN_POINT('Ctrl Pts',(-7.27603390513785,-85.4939842542419,
-4.20082013374671));
#30480=CARTESIAN_POINT('Ctrl Pts',(-9.70137854017371,-85.3189842542419,
1.74701493417668E-11));
#30481=CARTESIAN_POINT('Ctrl Pts',(-7.27603390512272,-85.143984254242,4.20082013377291));
#30482=CARTESIAN_POINT('Ctrl Pts',(-4.85068927007173,-84.9689842542419,
8.40164026752836));
#30483=CARTESIAN_POINT('Ctrl Pts',(1.5129078685785E-11,-84.7939842542419,
8.40164026751963));
#30484=CARTESIAN_POINT('Ctrl Pts',(4.85068927010198,-84.6189842542419,8.40164026751089));
#30485=CARTESIAN_POINT('Ctrl Pts',(7.27603390513785,-84.443984254242,4.20082013374671));
#30486=CARTESIAN_POINT('Ctrl Pts',(9.70137854017371,-84.2689842542419,-1.74689612655491E-11));
#30487=CARTESIAN_POINT('Ctrl Pts',(7.27603390512272,-84.0939842542419,-4.20082013377291));
#30488=CARTESIAN_POINT('Ctrl Pts',(4.85068927007173,-83.9189842542419,-8.40164026752836));
#30489=CARTESIAN_POINT('Ctrl Pts',(-1.51301075899711E-11,-83.7439842542419,
-8.40164026751963));
#30490=CARTESIAN_POINT('Ctrl Pts',(-4.85068927010198,-83.5689842542419,
-8.40164026751089));
#30491=CARTESIAN_POINT('Ctrl Pts',(-7.27603390513785,-83.3939842542419,
-4.20082013374671));
#30492=CARTESIAN_POINT('Ctrl Pts',(-9.70137854017371,-83.2189842542419,
1.74701493417668E-11));
#30493=CARTESIAN_POINT('Ctrl Pts',(-7.27603390512272,-83.0439842542419,
4.20082013377291));
#30494=CARTESIAN_POINT('Ctrl Pts',(-4.85068927007173,-82.868984254242,8.40164026752836));
#30495=CARTESIAN_POINT('Ctrl Pts',(1.5129078685785E-11,-82.6939842542419,
8.40164026751963));
#30496=CARTESIAN_POINT('Ctrl Pts',(4.85068927010198,-82.5189842542419,8.40164026751089));
#30497=CARTESIAN_POINT('Ctrl Pts',(7.27603390513785,-82.3439842542419,4.20082013374671));
#30498=CARTESIAN_POINT('Ctrl Pts',(9.70137854017371,-82.1689842542419,-1.74689612655491E-11));
#30499=CARTESIAN_POINT('Ctrl Pts',(7.27603390512272,-81.993984254242,-4.20082013377291));
#30500=CARTESIAN_POINT('Ctrl Pts',(4.85068927007173,-81.8189842542419,-8.40164026752836));
#30501=CARTESIAN_POINT('Ctrl Pts',(-1.51301075899711E-11,-81.6439842542419,
-8.40164026751963));
#30502=CARTESIAN_POINT('Ctrl Pts',(-4.85068927010198,-81.4689842542419,
-8.40164026751089));
#30503=CARTESIAN_POINT('Ctrl Pts',(-7.27603390513785,-81.293984254242,-4.20082013374671));
#30504=CARTESIAN_POINT('Ctrl Pts',(-9.70137854017371,-81.1189842542419,
1.74701493417668E-11));
#30505=CARTESIAN_POINT('Ctrl Pts',(-7.27603390512272,-80.9439842542419,
4.20082013377291));
#30506=CARTESIAN_POINT('Ctrl Pts',(-4.85068927007173,-80.768984254242,8.40164026752836));
#30507=CARTESIAN_POINT('Ctrl Pts',(1.5129078685785E-11,-80.5939842542419,
8.40164026751963));
#30508=CARTESIAN_POINT('Ctrl Pts',(4.85068927010198,-80.4189842542419,8.40164026751089));
#30509=CARTESIAN_POINT('Ctrl Pts',(7.27603390513785,-80.243984254242,4.20082013374671));
#30510=CARTESIAN_POINT('Ctrl Pts',(9.70137854017371,-80.068984254242,-1.74689612655491E-11));
#30511=CARTESIAN_POINT('Ctrl Pts',(7.27603390512272,-79.8939842542419,-4.20082013377291));
#30512=CARTESIAN_POINT('Ctrl Pts',(4.85068927007173,-79.7189842542419,-8.40164026752836));
#30513=CARTESIAN_POINT('Ctrl Pts',(-1.51301075899711E-11,-79.5439842542419,
-8.40164026751963));
#30514=CARTESIAN_POINT('Ctrl Pts',(-4.85068927010198,-79.368984254242,-8.40164026751089));
#30515=CARTESIAN_POINT('Ctrl Pts',(-7.27603390513785,-79.193984254242,-4.20082013374671));
#30516=CARTESIAN_POINT('Ctrl Pts',(-9.70137854017371,-79.0189842542419,
1.74701493417668E-11));
#30517=CARTESIAN_POINT('Ctrl Pts',(-7.27603390512272,-78.8439842542419,
4.20082013377291));
#30518=CARTESIAN_POINT('Ctrl Pts',(-4.85068927007173,-78.668984254242,8.40164026752836));
#30519=CARTESIAN_POINT('Ctrl Pts',(1.5129078685785E-11,-78.493984254242,
8.40164026751963));
#30520=CARTESIAN_POINT('Ctrl Pts',(4.85068927010198,-78.3189842542419,8.40164026751089));
#30521=CARTESIAN_POINT('Ctrl Pts',(7.27603390513785,-78.143984254242,4.20082013374671));
#30522=CARTESIAN_POINT('Ctrl Pts',(9.70137854017371,-77.968984254242,-1.74689612655491E-11));
#30523=CARTESIAN_POINT('Ctrl Pts',(7.27603390512272,-77.7939842542419,-4.20082013377291));
#30524=CARTESIAN_POINT('Ctrl Pts',(4.85068927007173,-77.618984254242,-8.40164026752836));
#30525=CARTESIAN_POINT('Ctrl Pts',(-1.51301075899711E-11,-77.443984254242,
-8.40164026751963));
#30526=CARTESIAN_POINT('Ctrl Pts',(-4.85068927010198,-77.268984254242,-8.40164026751089));
#30527=CARTESIAN_POINT('Ctrl Pts',(-7.27603390513785,-77.0939842542419,
-4.20082013374671));
#30528=CARTESIAN_POINT('Ctrl Pts',(-9.70137854017371,-76.918984254242,1.74701493417668E-11));
#30529=CARTESIAN_POINT('Ctrl Pts',(-7.27603390512272,-76.743984254242,4.20082013377291));
#30530=CARTESIAN_POINT('Ctrl Pts',(-4.85068927007173,-76.5689842542419,
8.40164026752836));
#30531=CARTESIAN_POINT('Ctrl Pts',(1.5129078685785E-11,-76.393984254242,
8.40164026751963));
#30532=CARTESIAN_POINT('Ctrl Pts',(4.85068927010198,-76.218984254242,8.40164026751089));
#30533=CARTESIAN_POINT('Ctrl Pts',(7.27603390513785,-76.0439842542419,4.20082013374671));
#30534=CARTESIAN_POINT('Ctrl Pts',(9.70137854017371,-75.868984254242,-1.74689612655491E-11));
#30535=CARTESIAN_POINT('Ctrl Pts',(7.27603390512272,-75.693984254242,-4.20082013377291));
#30536=CARTESIAN_POINT('Ctrl Pts',(4.85068927007173,-75.518984254242,-8.40164026752836));
#30537=CARTESIAN_POINT('Ctrl Pts',(-1.51301075899711E-11,-75.343984254242,
-8.40164026751963));
#30538=CARTESIAN_POINT('Ctrl Pts',(-4.85068927010198,-75.1689842542419,
-8.40164026751089));
#30539=CARTESIAN_POINT('Ctrl Pts',(-7.27603390513785,-74.993984254242,-4.20082013374671));
#30540=CARTESIAN_POINT('Ctrl Pts',(-9.70137854017371,-74.818984254242,1.74701493417668E-11));
#30541=CARTESIAN_POINT('Ctrl Pts',(-7.27603390512272,-74.643984254242,4.20082013377291));
#30542=CARTESIAN_POINT('Ctrl Pts',(-4.85068927007173,-74.4689842542419,
8.40164026752836));
#30543=CARTESIAN_POINT('Ctrl Pts',(1.5129078685785E-11,-74.293984254242,
8.40164026751963));
#30544=CARTESIAN_POINT('Ctrl Pts',(4.85068927010198,-74.118984254242,8.40164026751089));
#30545=CARTESIAN_POINT('Ctrl Pts',(7.27603390513785,-73.943984254242,4.20082013374671));
#30546=CARTESIAN_POINT('Ctrl Pts',(9.70137854017371,-73.768984254242,-1.74689612655491E-11));
#30547=CARTESIAN_POINT('Ctrl Pts',(7.27603390512272,-73.593984254242,-4.20082013377291));
#30548=CARTESIAN_POINT('Ctrl Pts',(4.85068927007173,-73.4189842542419,-8.40164026752836));
#30549=CARTESIAN_POINT('Ctrl Pts',(-1.51301075899711E-11,-73.243984254242,
-8.40164026751963));
#30550=CARTESIAN_POINT('Ctrl Pts',(-4.85068927010198,-73.068984254242,-8.40164026751089));
#30551=CARTESIAN_POINT('Ctrl Pts',(-7.27603390513785,-72.893984254242,-4.20082013374671));
#30552=CARTESIAN_POINT('Ctrl Pts',(-9.70137854017371,-72.718984254242,1.74701493417668E-11));
#30553=CARTESIAN_POINT('Ctrl Pts',(-7.27603390512272,-72.543984254242,4.20082013377291));
#30554=CARTESIAN_POINT('Ctrl Pts',(-4.85068927007173,-72.368984254242,8.40164026752836));
#30555=CARTESIAN_POINT('Ctrl Pts',(1.5129078685785E-11,-72.193984254242,
8.40164026751963));
#30556=CARTESIAN_POINT('Ctrl Pts',(4.85068927010198,-72.018984254242,8.40164026751089));
#30557=CARTESIAN_POINT('Ctrl Pts',(7.27603390513785,-71.843984254242,4.20082013374671));
#30558=CARTESIAN_POINT('Ctrl Pts',(9.70137854017371,-71.6689842542419,-1.74689612655491E-11));
#30559=CARTESIAN_POINT('Ctrl Pts',(7.27603390512272,-71.493984254242,-4.20082013377291));
#30560=CARTESIAN_POINT('Ctrl Pts',(4.85068927007173,-71.318984254242,-8.40164026752836));
#30561=CARTESIAN_POINT('Ctrl Pts',(-1.51301075899711E-11,-71.143984254242,
-8.40164026751963));
#30562=CARTESIAN_POINT('Ctrl Pts',(-4.85068927010198,-70.968984254242,-8.40164026751089));
#30563=CARTESIAN_POINT('Ctrl Pts',(-7.27603390513785,-70.793984254242,-4.20082013374671));
#30564=CARTESIAN_POINT('Ctrl Pts',(-9.70137854017371,-70.618984254242,1.74701493417668E-11));
#30565=CARTESIAN_POINT('Ctrl Pts',(-7.27603390512272,-70.443984254242,4.20082013377291));
#30566=CARTESIAN_POINT('Ctrl Pts',(-4.85068927007173,-70.268984254242,8.40164026752836));
#30567=CARTESIAN_POINT('Ctrl Pts',(1.5129078685785E-11,-70.093984254242,
8.40164026751963));
#30568=CARTESIAN_POINT('Ctrl Pts',(4.85068927010198,-69.918984254242,8.40164026751089));
#30569=CARTESIAN_POINT('Ctrl Pts',(7.27603390513785,-69.743984254242,4.20082013374671));
#30570=CARTESIAN_POINT('Ctrl Pts',(9.70137854017371,-69.568984254242,-1.74689612655491E-11));
#30571=CARTESIAN_POINT('Ctrl Pts',(7.27603390512272,-69.393984254242,-4.20082013377291));
#30572=CARTESIAN_POINT('Ctrl Pts',(4.85068927007173,-69.218984254242,-8.40164026752836));
#30573=CARTESIAN_POINT('Ctrl Pts',(-1.51301075899711E-11,-69.043984254242,
-8.40164026751963));
#30574=CARTESIAN_POINT('Ctrl Pts',(-4.85068927010198,-68.868984254242,-8.40164026751089));
#30575=CARTESIAN_POINT('Ctrl Pts',(-7.27603390513785,-68.693984254242,-4.20082013374671));
#30576=CARTESIAN_POINT('Ctrl Pts',(-9.70137854017371,-68.518984254242,1.74701493417668E-11));
#30577=CARTESIAN_POINT('Ctrl Pts',(-7.27603390512272,-68.343984254242,4.20082013377291));
#30578=CARTESIAN_POINT('Ctrl Pts',(-4.85068927007173,-68.168984254242,8.40164026752836));
#30579=CARTESIAN_POINT('Ctrl Pts',(1.5129078685785E-11,-67.993984254242,
8.40164026751963));
#30580=CARTESIAN_POINT('Ctrl Pts',(4.85068927010198,-67.818984254242,8.40164026751089));
#30581=CARTESIAN_POINT('Ctrl Pts',(7.27603390513785,-67.643984254242,4.20082013374671));
#30582=CARTESIAN_POINT('Ctrl Pts',(9.70137854017371,-67.468984254242,-1.74689612655491E-11));
#30583=CARTESIAN_POINT('Ctrl Pts',(7.27603390512272,-67.293984254242,-4.20082013377291));
#30584=CARTESIAN_POINT('Ctrl Pts',(4.85068927007173,-67.118984254242,-8.40164026752836));
#30585=CARTESIAN_POINT('Ctrl Pts',(-1.51301075899711E-11,-66.943984254242,
-8.40164026751963));
#30586=CARTESIAN_POINT('Ctrl Pts',(-4.85068927010198,-66.768984254242,-8.40164026751089));
#30587=CARTESIAN_POINT('Ctrl Pts',(-7.27603390513785,-66.593984254242,-4.20082013374671));
#30588=CARTESIAN_POINT('Ctrl Pts',(-9.70137854017371,-66.418984254242,1.74701493417668E-11));
#30589=CARTESIAN_POINT('Ctrl Pts',(-7.27603390512272,-66.243984254242,4.20082013377291));
#30590=CARTESIAN_POINT('Ctrl Pts',(-4.85068927007173,-66.068984254242,8.40164026752836));
#30591=CARTESIAN_POINT('Ctrl Pts',(1.5129078685785E-11,-65.893984254242,
8.40164026751963));
#30592=CARTESIAN_POINT('Ctrl Pts',(4.85068927010198,-65.718984254242,8.40164026751089));
#30593=CARTESIAN_POINT('Ctrl Pts',(7.27603390513785,-65.543984254242,4.20082013374671));
#30594=CARTESIAN_POINT('Ctrl Pts',(9.70137854017371,-65.368984254242,-1.74689612655491E-11));
#30595=CARTESIAN_POINT('Ctrl Pts',(7.27603390512272,-65.193984254242,-4.20082013377291));
#30596=CARTESIAN_POINT('Ctrl Pts',(4.85068927007173,-65.018984254242,-8.40164026752836));
#30597=CARTESIAN_POINT('Ctrl Pts',(-1.51301075899711E-11,-64.843984254242,
-8.40164026751963));
#30598=CARTESIAN_POINT('Ctrl Pts',(-4.85068927010198,-64.668984254242,-8.40164026751089));
#30599=CARTESIAN_POINT('Ctrl Pts',(-7.27603390513785,-64.493984254242,-4.20082013374671));
#30600=CARTESIAN_POINT('Ctrl Pts',(-9.70137854017371,-64.318984254242,1.74701493417668E-11));
#30601=CARTESIAN_POINT('Ctrl Pts',(-7.27603390512272,-64.143984254242,4.20082013377291));
#30602=CARTESIAN_POINT('Ctrl Pts',(-4.85068927007173,-63.968984254242,8.40164026752836));
#30603=CARTESIAN_POINT('Ctrl Pts',(1.5129078685785E-11,-63.793984254242,
8.40164026751963));
#30604=CARTESIAN_POINT('Ctrl Pts',(4.85068927010198,-63.618984254242,8.40164026751089));
#30605=CARTESIAN_POINT('Ctrl Pts',(7.27603390513785,-63.443984254242,4.20082013374671));
#30606=CARTESIAN_POINT('Ctrl Pts',(9.70137854017371,-63.268984254242,-1.74689612655491E-11));
#30607=CARTESIAN_POINT('Ctrl Pts',(7.27603390512272,-63.093984254242,-4.20082013377291));
#30608=CARTESIAN_POINT('Ctrl Pts',(4.85068927007173,-62.918984254242,-8.40164026752836));
#30609=CARTESIAN_POINT('Ctrl Pts',(-1.51301075899711E-11,-62.743984254242,
-8.40164026751963));
#30610=CARTESIAN_POINT('Ctrl Pts',(-4.85068927010198,-62.568984254242,-8.40164026751089));
#30611=CARTESIAN_POINT('Ctrl Pts',(-7.27603390513785,-62.393984254242,-4.20082013374671));
#30612=CARTESIAN_POINT('Ctrl Pts',(-9.70137854017371,-62.218984254242,1.74701493417668E-11));
#30613=CARTESIAN_POINT('Ctrl Pts',(-7.27603390512272,-62.043984254242,4.20082013377291));
#30614=CARTESIAN_POINT('Ctrl Pts',(-4.85068927007173,-61.868984254242,8.40164026752836));
#30615=CARTESIAN_POINT('Ctrl Pts',(1.5129078685785E-11,-61.693984254242,
8.40164026751963));
#30616=CARTESIAN_POINT('Ctrl Pts',(4.85068927010198,-61.518984254242,8.40164026751089));
#30617=CARTESIAN_POINT('Ctrl Pts',(7.27603390513785,-61.343984254242,4.20082013374671));
#30618=CARTESIAN_POINT('Ctrl Pts',(9.70137854017371,-61.168984254242,-1.74689612655491E-11));
#30619=CARTESIAN_POINT('Ctrl Pts',(7.27603390512272,-60.993984254242,-4.20082013377291));
#30620=CARTESIAN_POINT('Ctrl Pts',(4.85068927007173,-60.818984254242,-8.40164026752836));
#30621=CARTESIAN_POINT('Ctrl Pts',(-1.51301075899711E-11,-60.643984254242,
-8.40164026751963));
#30622=CARTESIAN_POINT('Ctrl Pts',(-4.85068927010198,-60.468984254242,-8.40164026751089));
#30623=CARTESIAN_POINT('Ctrl Pts',(-7.27603390513785,-60.293984254242,-4.20082013374671));
#30624=CARTESIAN_POINT('Ctrl Pts',(-9.70137854017371,-60.118984254242,1.74701493417668E-11));
#30625=CARTESIAN_POINT('Ctrl Pts',(-7.27603390512272,-59.943984254242,4.20082013377291));
#30626=CARTESIAN_POINT('Ctrl Pts',(-4.85068927007173,-59.768984254242,8.40164026752836));
#30627=CARTESIAN_POINT('Ctrl Pts',(1.5129078685785E-11,-59.593984254242,
8.40164026751963));
#30628=CARTESIAN_POINT('Ctrl Pts',(4.85068927010198,-59.418984254242,8.40164026751089));
#30629=CARTESIAN_POINT('Ctrl Pts',(7.27603390513785,-59.243984254242,4.20082013374671));
#30630=CARTESIAN_POINT('Ctrl Pts',(9.70137854017371,-59.068984254242,-1.74689612655491E-11));
#30631=CARTESIAN_POINT('Ctrl Pts',(7.27603390512272,-58.893984254242,-4.20082013377291));
#30632=CARTESIAN_POINT('Ctrl Pts',(4.85068927007173,-58.718984254242,-8.40164026752836));
#30633=CARTESIAN_POINT('Ctrl Pts',(-1.51301075899711E-11,-58.543984254242,
-8.40164026751963));
#30634=CARTESIAN_POINT('Ctrl Pts',(-4.85068927010198,-58.368984254242,-8.40164026751089));
#30635=CARTESIAN_POINT('Ctrl Pts',(-7.27603390513785,-58.193984254242,-4.20082013374671));
#30636=CARTESIAN_POINT('Ctrl Pts',(-9.70137854017371,-58.018984254242,1.74701493417668E-11));
#30637=CARTESIAN_POINT('Ctrl Pts',(-7.27603390512272,-57.843984254242,4.20082013377291));
#30638=CARTESIAN_POINT('Ctrl Pts',(-4.85068927007173,-57.668984254242,8.40164026752836));
#30639=CARTESIAN_POINT('Ctrl Pts',(1.5129078685785E-11,-57.493984254242,
8.40164026751963));
#30640=CARTESIAN_POINT('Ctrl Pts',(4.85068927010198,-57.318984254242,8.40164026751089));
#30641=CARTESIAN_POINT('Ctrl Pts',(7.27603390513785,-57.143984254242,4.20082013374671));
#30642=CARTESIAN_POINT('Ctrl Pts',(9.70137854017371,-56.968984254242,-1.74689612655491E-11));
#30643=CARTESIAN_POINT('Ctrl Pts',(7.27603390512272,-56.793984254242,-4.20082013377291));
#30644=CARTESIAN_POINT('Ctrl Pts',(4.85068927007173,-56.618984254242,-8.40164026752836));
#30645=CARTESIAN_POINT('Ctrl Pts',(-1.51301075899711E-11,-56.443984254242,
-8.40164026751963));
#30646=CARTESIAN_POINT('Ctrl Pts',(-4.85068927010198,-56.268984254242,-8.40164026751089));
#30647=CARTESIAN_POINT('Ctrl Pts',(-7.27603390513785,-56.093984254242,-4.20082013374671));
#30648=CARTESIAN_POINT('Ctrl Pts',(-9.70137854017371,-55.918984254242,1.74701493417668E-11));
#30649=CARTESIAN_POINT('Ctrl Pts',(-7.27603390512272,-55.743984254242,4.20082013377291));
#30650=CARTESIAN_POINT('Ctrl Pts',(-4.85068927007173,-55.568984254242,8.40164026752836));
#30651=CARTESIAN_POINT('Ctrl Pts',(1.5129078685785E-11,-55.393984254242,
8.40164026751963));
#30652=CARTESIAN_POINT('Ctrl Pts',(4.85068927010198,-55.218984254242,8.40164026751089));
#30653=CARTESIAN_POINT('Ctrl Pts',(7.27603390513785,-55.043984254242,4.20082013374671));
#30654=CARTESIAN_POINT('Ctrl Pts',(9.70137854017371,-54.868984254242,-1.74689612655491E-11));
#30655=CARTESIAN_POINT('Ctrl Pts',(7.27603390512272,-54.693984254242,-4.20082013377291));
#30656=CARTESIAN_POINT('Ctrl Pts',(4.85068927007173,-54.518984254242,-8.40164026752836));
#30657=CARTESIAN_POINT('Ctrl Pts',(-1.51301075899711E-11,-54.343984254242,
-8.40164026751963));
#30658=CARTESIAN_POINT('Ctrl Pts',(-4.85068927010198,-54.168984254242,-8.40164026751089));
#30659=CARTESIAN_POINT('Ctrl Pts',(-7.27603390513785,-53.993984254242,-4.20082013374671));
#30660=CARTESIAN_POINT('Ctrl Pts',(-9.70137854017371,-53.818984254242,1.74701493417668E-11));
#30661=CARTESIAN_POINT('Ctrl Pts',(-7.27603390512272,-53.643984254242,4.20082013377291));
#30662=CARTESIAN_POINT('Ctrl Pts',(-4.85068927007173,-53.468984254242,8.40164026752836));
#30663=CARTESIAN_POINT('Ctrl Pts',(1.5129078685785E-11,-53.293984254242,
8.40164026751963));
#30664=CARTESIAN_POINT('Ctrl Pts',(4.85068927010198,-53.118984254242,8.40164026751089));
#30665=CARTESIAN_POINT('Ctrl Pts',(7.27603390513785,-52.943984254242,4.20082013374671));
#30666=CARTESIAN_POINT('Ctrl Pts',(9.70137854017371,-52.768984254242,-1.74689612655491E-11));
#30667=CARTESIAN_POINT('Ctrl Pts',(7.27603390512272,-52.593984254242,-4.20082013377291));
#30668=CARTESIAN_POINT('Ctrl Pts',(4.85068927007173,-52.418984254242,-8.40164026752836));
#30669=CARTESIAN_POINT('Ctrl Pts',(-1.51301075899711E-11,-52.243984254242,
-8.40164026751963));
#30670=CARTESIAN_POINT('Ctrl Pts',(-4.85068927010198,-52.068984254242,-8.40164026751089));
#30671=CARTESIAN_POINT('Ctrl Pts',(-7.27603390513785,-51.893984254242,-4.20082013374671));
#30672=CARTESIAN_POINT('Ctrl Pts',(-9.70137854017371,-51.718984254242,1.74701493417668E-11));
#30673=CARTESIAN_POINT('Ctrl Pts',(-7.27603390512272,-51.543984254242,4.20082013377291));
#30674=CARTESIAN_POINT('Ctrl Pts',(-4.85068927007173,-51.368984254242,8.40164026752836));
#30675=CARTESIAN_POINT('Ctrl Pts',(1.5129078685785E-11,-51.193984254242,
8.40164026751963));
#30676=CARTESIAN_POINT('Ctrl Pts',(4.85068927010198,-51.018984254242,8.40164026751089));
#30677=CARTESIAN_POINT('Ctrl Pts',(7.27603390513785,-50.843984254242,4.20082013374671));
#30678=CARTESIAN_POINT('Ctrl Pts',(9.70137854017371,-50.668984254242,-1.74689612655491E-11));
#30679=CARTESIAN_POINT('Ctrl Pts',(7.27603390512272,-50.493984254242,-4.20082013377291));
#30680=CARTESIAN_POINT('Ctrl Pts',(4.85068927007173,-50.318984254242,-8.40164026752836));
#30681=CARTESIAN_POINT('Ctrl Pts',(-1.51301075899711E-11,-50.143984254242,
-8.40164026751963));
#30682=CARTESIAN_POINT('Ctrl Pts',(-4.85068927010198,-49.968984254242,-8.40164026751089));
#30683=CARTESIAN_POINT('Ctrl Pts',(-7.27603390513785,-49.793984254242,-4.20082013374671));
#30684=CARTESIAN_POINT('Ctrl Pts',(-9.70137854017371,-49.618984254242,1.74701493417668E-11));
#30685=CARTESIAN_POINT('Ctrl Pts',(-7.27603390512272,-49.443984254242,4.20082013377291));
#30686=CARTESIAN_POINT('Ctrl Pts',(-4.85068927007173,-49.268984254242,8.40164026752836));
#30687=CARTESIAN_POINT('Ctrl Pts',(1.5129078685785E-11,-49.093984254242,
8.40164026751963));
#30688=CARTESIAN_POINT('Ctrl Pts',(4.85068927010198,-48.918984254242,8.40164026751089));
#30689=CARTESIAN_POINT('Ctrl Pts',(7.27603390513785,-48.743984254242,4.20082013374671));
#30690=CARTESIAN_POINT('Ctrl Pts',(9.70137854017371,-48.568984254242,-1.74689612655491E-11));
#30691=CARTESIAN_POINT('Ctrl Pts',(7.27603390512272,-48.393984254242,-4.20082013377291));
#30692=CARTESIAN_POINT('Ctrl Pts',(4.85068927007173,-48.218984254242,-8.40164026752836));
#30693=CARTESIAN_POINT('Ctrl Pts',(-1.51301075899711E-11,-48.043984254242,
-8.40164026751963));
#30694=CARTESIAN_POINT('Ctrl Pts',(-4.85068927010198,-47.868984254242,-8.40164026751089));
#30695=CARTESIAN_POINT('Ctrl Pts',(-7.27603390513785,-47.693984254242,-4.20082013374671));
#30696=CARTESIAN_POINT('Ctrl Pts',(-9.70137854017371,-47.518984254242,1.74701493417668E-11));
#30697=CARTESIAN_POINT('Ctrl Pts',(-7.27603390512272,-47.343984254242,4.20082013377291));
#30698=CARTESIAN_POINT('Ctrl Pts',(-4.85068927007173,-47.168984254242,8.40164026752836));
#30699=CARTESIAN_POINT('Ctrl Pts',(1.5129078685785E-11,-46.993984254242,
8.40164026751963));
#30700=CARTESIAN_POINT('Ctrl Pts',(4.85068927010198,-46.818984254242,8.40164026751089));
#30701=CARTESIAN_POINT('Ctrl Pts',(7.27603390513785,-46.643984254242,4.20082013374671));
#30702=CARTESIAN_POINT('Ctrl Pts',(9.70137854017371,-46.468984254242,-1.74689612655491E-11));
#30703=CARTESIAN_POINT('Ctrl Pts',(7.27603390512272,-46.293984254242,-4.20082013377291));
#30704=CARTESIAN_POINT('Ctrl Pts',(4.85068927007173,-46.118984254242,-8.40164026752836));
#30705=CARTESIAN_POINT('Ctrl Pts',(-1.51301075899711E-11,-45.943984254242,
-8.40164026751963));
#30706=CARTESIAN_POINT('Ctrl Pts',(-4.85068927010198,-45.768984254242,-8.40164026751089));
#30707=CARTESIAN_POINT('Ctrl Pts',(-7.27603390513785,-45.593984254242,-4.20082013374671));
#30708=CARTESIAN_POINT('Ctrl Pts',(-9.70137854017371,-45.418984254242,1.74701493417668E-11));
#30709=CARTESIAN_POINT('Ctrl Pts',(-7.27603390512272,-45.243984254242,4.20082013377291));
#30710=CARTESIAN_POINT('Ctrl Pts',(-4.85068927007173,-45.068984254242,8.40164026752836));
#30711=CARTESIAN_POINT('Ctrl Pts',(1.5129078685785E-11,-44.893984254242,
8.40164026751963));
#30712=CARTESIAN_POINT('Ctrl Pts',(4.85068927010198,-44.718984254242,8.40164026751089));
#30713=CARTESIAN_POINT('Ctrl Pts',(7.27603390513785,-44.543984254242,4.20082013374671));
#30714=CARTESIAN_POINT('Ctrl Pts',(9.70137854017371,-44.368984254242,-1.74689612655491E-11));
#30715=CARTESIAN_POINT('Ctrl Pts',(7.27603390512272,-44.193984254242,-4.20082013377291));
#30716=CARTESIAN_POINT('Ctrl Pts',(4.85068927007173,-44.018984254242,-8.40164026752836));
#30717=CARTESIAN_POINT('Ctrl Pts',(-1.51301075899711E-11,-43.843984254242,
-8.40164026751963));
#30718=CARTESIAN_POINT('',(5.91264939824166,-212.63,5.96893091585754));
#30719=CARTESIAN_POINT('Ctrl Pts',(5.91264939824165,-212.63,5.96893091585754));
#30720=CARTESIAN_POINT('Ctrl Pts',(6.71286052373726,-212.584619857249,5.17626504380697));
#30721=CARTESIAN_POINT('Ctrl Pts',(7.27603390513785,-212.543984254242,4.20082013374672));
#30722=CARTESIAN_POINT('Ctrl Pts',(9.70137854017372,-212.368984254242,-1.74689612655491E-11));
#30723=CARTESIAN_POINT('Ctrl Pts',(7.27603390512273,-212.193984254242,-4.20082013377291));
#30724=CARTESIAN_POINT('Ctrl Pts',(4.85068927007173,-212.018984254242,-8.40164026752836));
#30725=CARTESIAN_POINT('Ctrl Pts',(-1.51280497815988E-11,-211.843984254242,
-8.40164026751963));
#30726=CARTESIAN_POINT('Ctrl Pts',(-4.85068927010198,-211.668984254242,
-8.4016402675109));
#30727=CARTESIAN_POINT('Ctrl Pts',(-7.27603390513785,-211.493984254242,
-4.20082013374672));
#30728=CARTESIAN_POINT('Ctrl Pts',(-9.70137854017372,-211.318984254242,
1.74591566342707E-11));
#30729=CARTESIAN_POINT('Ctrl Pts',(-7.27603390512273,-211.143984254242,
4.20082013377291));
#30730=CARTESIAN_POINT('Ctrl Pts',(-4.85068927007174,-210.968984254242,
8.40164026752836));
#30731=CARTESIAN_POINT('Ctrl Pts',(1.51270208774127E-11,-210.793984254242,
8.40164026751963));
#30732=CARTESIAN_POINT('Ctrl Pts',(4.85068927010198,-210.618984254242,8.4016402675109));
#30733=CARTESIAN_POINT('Ctrl Pts',(7.27603390513785,-210.443984254242,4.20082013374672));
#30734=CARTESIAN_POINT('Ctrl Pts',(9.70137854017372,-210.268984254242,-1.74665851131138E-11));
#30735=CARTESIAN_POINT('Ctrl Pts',(7.27603390512273,-210.093984254242,-4.20082013377291));
#30736=CARTESIAN_POINT('Ctrl Pts',(4.85068927007174,-209.918984254242,-8.40164026752836));
#30737=CARTESIAN_POINT('Ctrl Pts',(-1.51259919732266E-11,-209.743984254242,
-8.40164026751963));
#30738=CARTESIAN_POINT('Ctrl Pts',(-4.85068927010198,-209.568984254242,
-8.4016402675109));
#30739=CARTESIAN_POINT('Ctrl Pts',(-7.27603390513785,-209.393984254242,
-4.20082013374672));
#30740=CARTESIAN_POINT('Ctrl Pts',(-9.70137854017372,-209.218984254242,
1.74481639267747E-11));
#30741=CARTESIAN_POINT('Ctrl Pts',(-7.27603390512273,-209.043984254242,
4.20082013377291));
#30742=CARTESIAN_POINT('Ctrl Pts',(-4.85068927007174,-208.868984254242,
8.40164026752836));
#30743=CARTESIAN_POINT('Ctrl Pts',(1.51100387578891E-11,-208.693984254242,
8.40164026751963));
#30744=CARTESIAN_POINT('Ctrl Pts',(4.85068927010198,-208.518984254242,8.4016402675109));
#30745=CARTESIAN_POINT('Ctrl Pts',(7.27603390513784,-208.343984254242,4.20082013374673));
#30746=CARTESIAN_POINT('Ctrl Pts',(9.70137854017372,-208.168984254242,-1.74469758505571E-11));
#30747=CARTESIAN_POINT('Ctrl Pts',(7.27603390512273,-207.993984254242,-4.2008201337729));
#30748=CARTESIAN_POINT('Ctrl Pts',(4.85068927007176,-207.818984254242,-8.40164026752835));
#30749=CARTESIAN_POINT('Ctrl Pts',(-1.51239341648544E-11,-207.643984254242,
-8.40164026751963));
#30750=CARTESIAN_POINT('Ctrl Pts',(-4.85068927010198,-207.468984254242,
-8.4016402675109));
#30751=CARTESIAN_POINT('Ctrl Pts',(-7.27603390513784,-207.293984254242,
-4.20082013374673));
#30752=CARTESIAN_POINT('Ctrl Pts',(-9.70137854017372,-207.118984254242,
1.74457877743394E-11));
#30753=CARTESIAN_POINT('Ctrl Pts',(-7.27603390512273,-206.943984254242,
4.20082013377289));
#30754=CARTESIAN_POINT('Ctrl Pts',(-4.85068927007176,-206.768984254242,
8.40164026752835));
#30755=CARTESIAN_POINT('Ctrl Pts',(1.51229052606682E-11,-206.593984254242,
8.40164026751963));
#30756=CARTESIAN_POINT('Ctrl Pts',(4.85068927010198,-206.418984254242,8.4016402675109));
#30757=CARTESIAN_POINT('Ctrl Pts',(7.27603390513784,-206.243984254242,4.20082013374673));
#30758=CARTESIAN_POINT('Ctrl Pts',(9.70137854017372,-206.068984254242,-1.74445996981217E-11));
#30759=CARTESIAN_POINT('Ctrl Pts',(7.27603390512273,-205.893984254242,-4.20082013377289));
#30760=CARTESIAN_POINT('Ctrl Pts',(4.85068927007176,-205.718984254242,-8.40164026752835));
#30761=CARTESIAN_POINT('Ctrl Pts',(-1.51218763564821E-11,-205.543984254242,
-8.40164026751963));
#30762=CARTESIAN_POINT('Ctrl Pts',(-4.85068927010197,-205.368984254242,
-8.4016402675109));
#30763=CARTESIAN_POINT('Ctrl Pts',(-7.27603390513784,-205.193984254242,
-4.20082013374673));
#30764=CARTESIAN_POINT('Ctrl Pts',(-9.70137854017372,-205.018984254242,
1.74434116219041E-11));
#30765=CARTESIAN_POINT('Ctrl Pts',(-7.27603390512274,-204.843984254242,
4.20082013377289));
#30766=CARTESIAN_POINT('Ctrl Pts',(-4.85068927007176,-204.668984254242,
8.40164026752834));
#30767=CARTESIAN_POINT('Ctrl Pts',(1.50909988299932E-11,-204.493984254242,
8.40164026751963));
#30768=CARTESIAN_POINT('Ctrl Pts',(4.85068927010197,-204.318984254242,8.4016402675109));
#30769=CARTESIAN_POINT('Ctrl Pts',(7.27603390513784,-204.143984254242,4.20082013374673));
#30770=CARTESIAN_POINT('Ctrl Pts',(9.70137854017372,-203.968984254242,-1.74422235456864E-11));
#30771=CARTESIAN_POINT('Ctrl Pts',(7.27603390512274,-203.793984254242,-4.20082013377289));
#30772=CARTESIAN_POINT('Ctrl Pts',(4.85068927007176,-203.618984254242,-8.40164026752834));
#30773=CARTESIAN_POINT('Ctrl Pts',(-1.50899699258071E-11,-203.443984254242,
-8.40164026751963));
#30774=CARTESIAN_POINT('Ctrl Pts',(-4.85068927010197,-203.268984254242,
-8.4016402675109));
#30775=CARTESIAN_POINT('Ctrl Pts',(-7.27603390513784,-203.093984254242,
-4.20082013374673));
#30776=CARTESIAN_POINT('Ctrl Pts',(-9.70137854017372,-202.918984254242,
1.74065692492259E-11));
#30777=CARTESIAN_POINT('Ctrl Pts',(-7.27603390512274,-202.743984254242,
4.20082013377289));
#30778=CARTESIAN_POINT('Ctrl Pts',(-4.85068927007173,-202.568984254242,
8.40164026752836));
#30779=CARTESIAN_POINT('Ctrl Pts',(1.5088941021621E-11,-202.393984254242,
8.40164026751963));
#30780=CARTESIAN_POINT('Ctrl Pts',(4.85068927010197,-202.218984254242,8.4016402675109));
#30781=CARTESIAN_POINT('Ctrl Pts',(7.27603390513783,-202.043984254242,4.20082013374676));
#30782=CARTESIAN_POINT('Ctrl Pts',(9.70137854017372,-201.868984254242,-1.74398473932511E-11));
#30783=CARTESIAN_POINT('Ctrl Pts',(7.27603390512275,-201.693984254242,-4.20082013377287));
#30784=CARTESIAN_POINT('Ctrl Pts',(4.85068927007176,-201.518984254242,-8.40164026752834));
#30785=CARTESIAN_POINT('Ctrl Pts',(-1.51177607397376E-11,-201.343984254242,
-8.40164026751963));
#30786=CARTESIAN_POINT('Ctrl Pts',(-4.85068927010194,-201.168984254242,
-8.40164026751092));
#30787=CARTESIAN_POINT('Ctrl Pts',(-7.27603390513784,-200.993984254242,
-4.20082013374673));
#30788=CARTESIAN_POINT('Ctrl Pts',(-9.70137854017372,-200.818984254242,
1.74041930967906E-11));
#30789=CARTESIAN_POINT('Ctrl Pts',(-7.27603390512274,-200.643984254242,
4.20082013377289));
#30790=CARTESIAN_POINT('Ctrl Pts',(-4.85068927007174,-200.468984254242,
8.40164026752836));
#30791=CARTESIAN_POINT('Ctrl Pts',(1.50868832132487E-11,-200.293984254242,
8.40164026751963));
#30792=CARTESIAN_POINT('Ctrl Pts',(4.85068927010197,-200.118984254242,8.4016402675109));
#30793=CARTESIAN_POINT('Ctrl Pts',(7.27603390513783,-199.943984254242,4.20082013374676));
#30794=CARTESIAN_POINT('Ctrl Pts',(9.70137854017372,-199.768984254242,-1.74374712408158E-11));
#30795=CARTESIAN_POINT('Ctrl Pts',(7.27603390512275,-199.593984254242,-4.20082013377286));
#30796=CARTESIAN_POINT('Ctrl Pts',(4.85068927007177,-199.418984254242,-8.40164026752834));
#30797=CARTESIAN_POINT('Ctrl Pts',(-1.51157029313654E-11,-199.243984254242,
-8.40164026751963));
#30798=CARTESIAN_POINT('Ctrl Pts',(-4.85068927010194,-199.068984254242,
-8.40164026751092));
#30799=CARTESIAN_POINT('Ctrl Pts',(-7.27603390513784,-198.893984254242,
-4.20082013374673));
#30800=CARTESIAN_POINT('Ctrl Pts',(-9.70137854017372,-198.718984254242,
1.74018169443553E-11));
#30801=CARTESIAN_POINT('Ctrl Pts',(-7.27603390512274,-198.543984254242,
4.20082013377289));
#30802=CARTESIAN_POINT('Ctrl Pts',(-4.8506892700718,-198.368984254242,8.40164026752832));
#30803=CARTESIAN_POINT('Ctrl Pts',(1.50848254048765E-11,-198.193984254242,
8.40164026751963));
#30804=CARTESIAN_POINT('Ctrl Pts',(4.85068927010197,-198.018984254242,8.4016402675109));
#30805=CARTESIAN_POINT('Ctrl Pts',(7.27603390513782,-197.843984254242,4.20082013374676));
#30806=CARTESIAN_POINT('Ctrl Pts',(9.70137854017372,-197.668984254242,-1.74350950883805E-11));
#30807=CARTESIAN_POINT('Ctrl Pts',(7.27603390512276,-197.493984254242,-4.20082013377286));
#30808=CARTESIAN_POINT('Ctrl Pts',(4.85068927007177,-197.318984254242,-8.40164026752834));
#30809=CARTESIAN_POINT('Ctrl Pts',(-1.51136451229931E-11,-197.143984254242,
-8.40164026751963));
#30810=CARTESIAN_POINT('Ctrl Pts',(-4.85068927010194,-196.968984254242,
-8.40164026751092));
#30811=CARTESIAN_POINT('Ctrl Pts',(-7.27603390513784,-196.793984254242,
-4.20082013374673));
#30812=CARTESIAN_POINT('Ctrl Pts',(-9.70137854017372,-196.618984254242,
1.739944079192E-11));
#30813=CARTESIAN_POINT('Ctrl Pts',(-7.27603390512274,-196.443984254242,
4.20082013377289));
#30814=CARTESIAN_POINT('Ctrl Pts',(-4.8506892700718,-196.268984254242,8.40164026752832));
#30815=CARTESIAN_POINT('Ctrl Pts',(1.50827675965043E-11,-196.093984254242,
8.40164026751963));
#30816=CARTESIAN_POINT('Ctrl Pts',(4.85068927010196,-195.918984254242,8.40164026751091));
#30817=CARTESIAN_POINT('Ctrl Pts',(7.27603390513782,-195.743984254242,4.20082013374676));
#30818=CARTESIAN_POINT('Ctrl Pts',(9.70137854017372,-195.568984254242,-1.74327189359452E-11));
#30819=CARTESIAN_POINT('Ctrl Pts',(7.27603390512276,-195.393984254242,-4.20082013377286));
#30820=CARTESIAN_POINT('Ctrl Pts',(4.85068927007177,-195.218984254242,-8.40164026752834));
#30821=CARTESIAN_POINT('Ctrl Pts',(-1.50518900700154E-11,-195.043984254242,
-8.40164026751963));
#30822=CARTESIAN_POINT('Ctrl Pts',(-4.85068927010193,-194.868984254242,
-8.40164026751092));
#30823=CARTESIAN_POINT('Ctrl Pts',(-7.27603390513784,-194.693984254242,
-4.20082013374674));
#30824=CARTESIAN_POINT('Ctrl Pts',(-9.70137854017372,-194.518984254242,
1.73970646394847E-11));
#30825=CARTESIAN_POINT('Ctrl Pts',(-7.27603390512274,-194.343984254242,
4.20082013377288));
#30826=CARTESIAN_POINT('Ctrl Pts',(-4.8506892700718,-194.168984254242,8.40164026752832));
#30827=CARTESIAN_POINT('Ctrl Pts',(1.5080709788132E-11,-193.993984254242,
8.40164026751963));
#30828=CARTESIAN_POINT('Ctrl Pts',(4.8506892701019,-193.818984254242,8.40164026751094));
#30829=CARTESIAN_POINT('Ctrl Pts',(7.27603390513782,-193.643984254242,4.20082013374676));
#30830=CARTESIAN_POINT('Ctrl Pts',(9.70137854017372,-193.468984254242,-1.74303427835099E-11));
#30831=CARTESIAN_POINT('Ctrl Pts',(7.27603390512276,-193.293984254242,-4.20082013377286));
#30832=CARTESIAN_POINT('Ctrl Pts',(4.85068927007177,-193.118984254242,-8.40164026752834));
#30833=CARTESIAN_POINT('Ctrl Pts',(-1.50498322616431E-11,-192.943984254242,
-8.40164026751963));
#30834=CARTESIAN_POINT('Ctrl Pts',(-4.85068927010193,-192.768984254242,
-8.40164026751093));
#30835=CARTESIAN_POINT('Ctrl Pts',(-7.27603390513784,-192.593984254242,
-4.20082013374674));
#30836=CARTESIAN_POINT('Ctrl Pts',(-9.70137854017372,-192.418984254242,
1.73946884870493E-11));
#30837=CARTESIAN_POINT('Ctrl Pts',(-7.27603390512274,-192.243984254242,
4.20082013377288));
#30838=CARTESIAN_POINT('Ctrl Pts',(-4.85068927007174,-192.068984254242,
8.40164026752836));
#30839=CARTESIAN_POINT('Ctrl Pts',(1.50189547351542E-11,-191.893984254242,
8.40164026751963));
#30840=CARTESIAN_POINT('Ctrl Pts',(4.8506892701019,-191.718984254242,8.40164026751094));
#30841=CARTESIAN_POINT('Ctrl Pts',(7.27603390513782,-191.543984254242,4.20082013374676));
#30842=CARTESIAN_POINT('Ctrl Pts',(9.70137854017372,-191.368984254242,-1.74279666310746E-11));
#30843=CARTESIAN_POINT('Ctrl Pts',(7.27603390512273,-191.193984254242,-4.20082013377291));
#30844=CARTESIAN_POINT('Ctrl Pts',(4.85068927007184,-191.018984254242,-8.4016402675283));
#30845=CARTESIAN_POINT('Ctrl Pts',(-1.50477744532709E-11,-190.843984254242,
-8.40164026751963));
#30846=CARTESIAN_POINT('Ctrl Pts',(-4.85068927010193,-190.668984254242,
-8.40164026751093));
#30847=CARTESIAN_POINT('Ctrl Pts',(-7.27603390513784,-190.493984254242,
-4.20082013374674));
#30848=CARTESIAN_POINT('Ctrl Pts',(-9.70137854017372,-190.318984254242,
1.74612447750998E-11));
#30849=CARTESIAN_POINT('Ctrl Pts',(-7.27603390512277,-190.143984254242,
4.20082013377283));
#30850=CARTESIAN_POINT('Ctrl Pts',(-4.8506892700718,-189.968984254242,8.40164026752832));
#30851=CARTESIAN_POINT('Ctrl Pts',(1.50765941713875E-11,-189.793984254242,
8.40164026751963));
#30852=CARTESIAN_POINT('Ctrl Pts',(4.85068927010196,-189.618984254242,8.40164026751091));
#30853=CARTESIAN_POINT('Ctrl Pts',(7.27603390513779,-189.443984254242,4.20082013374682));
#30854=CARTESIAN_POINT('Ctrl Pts',(9.70137854017372,-189.268984254242,-1.73566580381535E-11));
#30855=CARTESIAN_POINT('Ctrl Pts',(7.27603390512276,-189.093984254242,-4.20082013377285));
#30856=CARTESIAN_POINT('Ctrl Pts',(4.85068927007178,-188.918984254242,-8.40164026752834));
#30857=CARTESIAN_POINT('Ctrl Pts',(-1.51054138895042E-11,-188.743984254242,
-8.40164026751963));
#30858=CARTESIAN_POINT('Ctrl Pts',(-4.85068927010187,-188.568984254242,
-8.40164026751096));
#30859=CARTESIAN_POINT('Ctrl Pts',(-7.27603390513781,-188.393984254242,
-4.20082013374679));
#30860=CARTESIAN_POINT('Ctrl Pts',(-9.70137854017372,-188.218984254242,
1.73899361821787E-11));
#30861=CARTESIAN_POINT('Ctrl Pts',(-7.27603390512274,-188.043984254242,
4.20082013377288));
#30862=CARTESIAN_POINT('Ctrl Pts',(-4.85068927007175,-187.868984254242,
8.40164026752835));
#30863=CARTESIAN_POINT('Ctrl Pts',(1.50148391184097E-11,-187.693984254242,
8.40164026751963));
#30864=CARTESIAN_POINT('Ctrl Pts',(4.8506892701019,-187.518984254242,8.40164026751095));
#30865=CARTESIAN_POINT('Ctrl Pts',(7.27603390513782,-187.343984254242,4.20082013374677));
#30866=CARTESIAN_POINT('Ctrl Pts',(9.70137854017372,-187.168984254242,-1.7423214326204E-11));
#30867=CARTESIAN_POINT('Ctrl Pts',(7.27603390512273,-186.993984254242,-4.2008201337729));
#30868=CARTESIAN_POINT('Ctrl Pts',(4.85068927007184,-186.818984254242,-8.4016402675283));
#30869=CARTESIAN_POINT('Ctrl Pts',(-1.50436588365264E-11,-186.643984254242,
-8.40164026751963));
#30870=CARTESIAN_POINT('Ctrl Pts',(-4.85068927010193,-186.468984254242,
-8.40164026751093));
#30871=CARTESIAN_POINT('Ctrl Pts',(-7.27603390513783,-186.293984254242,
-4.20082013374674));
#30872=CARTESIAN_POINT('Ctrl Pts',(-9.70137854017372,-186.118984254242,
1.73186275892576E-11));
#30873=CARTESIAN_POINT('Ctrl Pts',(-7.27603390512277,-185.943984254242,
4.20082013377283));
#30874=CARTESIAN_POINT('Ctrl Pts',(-4.85068927007181,-185.768984254242,
8.40164026752832));
#30875=CARTESIAN_POINT('Ctrl Pts',(1.5072478554643E-11,-185.593984254242,
8.40164026751963));
#30876=CARTESIAN_POINT('Ctrl Pts',(4.85068927010196,-185.418984254242,8.40164026751091));
#30877=CARTESIAN_POINT('Ctrl Pts',(7.27603390513779,-185.243984254242,4.20082013374682));
#30878=CARTESIAN_POINT('Ctrl Pts',(9.70137854017372,-185.068984254242,-1.73519057332829E-11));
#30879=CARTESIAN_POINT('Ctrl Pts',(7.27603390512276,-184.893984254242,-4.20082013377285));
#30880=CARTESIAN_POINT('Ctrl Pts',(4.85068927007178,-184.718984254242,-8.40164026752833));
#30881=CARTESIAN_POINT('Ctrl Pts',(-1.51012982727597E-11,-184.543984254242,
-8.40164026751963));
#30882=CARTESIAN_POINT('Ctrl Pts',(-4.85068927010186,-184.368984254242,
-8.40164026751097));
#30883=CARTESIAN_POINT('Ctrl Pts',(-7.2760339051378,-184.193984254242,-4.2008201337468));
#30884=CARTESIAN_POINT('Ctrl Pts',(-9.70137854017372,-184.018984254242,
1.73851838773081E-11));
#30885=CARTESIAN_POINT('Ctrl Pts',(-7.27603390512275,-183.843984254242,
4.20082013377288));
#30886=CARTESIAN_POINT('Ctrl Pts',(-4.85068927007175,-183.668984254242,
8.40164026752835));
#30887=CARTESIAN_POINT('Ctrl Pts',(1.50107235016652E-11,-183.493984254242,
8.40164026751963));
#30888=CARTESIAN_POINT('Ctrl Pts',(4.85068927010189,-183.318984254242,8.40164026751095));
#30889=CARTESIAN_POINT('Ctrl Pts',(7.27603390513782,-183.143984254242,4.20082013374677));
#30890=CARTESIAN_POINT('Ctrl Pts',(9.70137854017372,-182.968984254242,-1.74184620213334E-11));
#30891=CARTESIAN_POINT('Ctrl Pts',(7.27603390512279,-182.793984254242,-4.2008201337728));
#30892=CARTESIAN_POINT('Ctrl Pts',(4.85068927007184,-182.618984254242,-8.4016402675283));
#30893=CARTESIAN_POINT('Ctrl Pts',(-1.50395432197819E-11,-182.443984254242,
-8.40164026751963));
#30894=CARTESIAN_POINT('Ctrl Pts',(-4.85068927010192,-182.268984254242,
-8.40164026751093));
#30895=CARTESIAN_POINT('Ctrl Pts',(-7.27603390513783,-182.093984254242,
-4.20082013374675));
#30896=CARTESIAN_POINT('Ctrl Pts',(-9.70137854017372,-181.918984254242,
1.7313875284387E-11));
#30897=CARTESIAN_POINT('Ctrl Pts',(-7.27603390512278,-181.743984254242,
4.20082013377282));
#30898=CARTESIAN_POINT('Ctrl Pts',(-4.85068927007181,-181.568984254242,
8.40164026752832));
#30899=CARTESIAN_POINT('Ctrl Pts',(1.50683629378986E-11,-181.393984254242,
8.40164026751963));
#30900=CARTESIAN_POINT('Ctrl Pts',(4.85068927010195,-181.218984254242,8.40164026751092));
#30901=CARTESIAN_POINT('Ctrl Pts',(7.27603390513779,-181.043984254242,4.20082013374683));
#30902=CARTESIAN_POINT('Ctrl Pts',(9.70137854017372,-180.868984254242,-1.73471534284123E-11));
#30903=CARTESIAN_POINT('Ctrl Pts',(7.27603390512276,-180.693984254242,-4.20082013377285));
#30904=CARTESIAN_POINT('Ctrl Pts',(4.85068927007178,-180.518984254242,-8.40164026752833));
#30905=CARTESIAN_POINT('Ctrl Pts',(-1.50971826560152E-11,-180.343984254242,
-8.40164026751963));
#30906=CARTESIAN_POINT('Ctrl Pts',(-4.85068927010186,-180.168984254242,
-8.40164026751097));
#30907=CARTESIAN_POINT('Ctrl Pts',(-7.2760339051378,-179.993984254242,-4.2008201337468));
#30908=CARTESIAN_POINT('Ctrl Pts',(-9.70137854017372,-179.818984254242,
1.73804315724375E-11));
#30909=CARTESIAN_POINT('Ctrl Pts',(-7.27603390512275,-179.643984254242,
4.20082013377287));
#30910=CARTESIAN_POINT('Ctrl Pts',(-4.85068927007188,-179.468984254242,
8.40164026752828));
#30911=CARTESIAN_POINT('Ctrl Pts',(1.50066078849208E-11,-179.293984254242,
8.40164026751963));
#30912=CARTESIAN_POINT('Ctrl Pts',(4.85068927010189,-179.118984254242,8.40164026751095));
#30913=CARTESIAN_POINT('Ctrl Pts',(7.27603390513782,-178.943984254242,4.20082013374678));
#30914=CARTESIAN_POINT('Ctrl Pts',(9.70137854017372,-178.768984254242,-1.74137097164627E-11));
#30915=CARTESIAN_POINT('Ctrl Pts',(7.27603390512279,-178.593984254242,-4.20082013377279));
#30916=CARTESIAN_POINT('Ctrl Pts',(4.85068927007185,-178.418984254242,-8.4016402675283));
#30917=CARTESIAN_POINT('Ctrl Pts',(-1.50354276030374E-11,-178.243984254242,
-8.40164026751963));
#30918=CARTESIAN_POINT('Ctrl Pts',(-4.85068927010192,-178.068984254242,
-8.40164026751093));
#30919=CARTESIAN_POINT('Ctrl Pts',(-7.27603390513783,-177.893984254242,
-4.20082013374675));
#30920=CARTESIAN_POINT('Ctrl Pts',(-9.70137854017372,-177.718984254242,
1.73091229795164E-11));
#30921=CARTESIAN_POINT('Ctrl Pts',(-7.27603390512278,-177.543984254242,
4.20082013377282));
#30922=CARTESIAN_POINT('Ctrl Pts',(-4.85068927007182,-177.368984254242,
8.40164026752831));
#30923=CARTESIAN_POINT('Ctrl Pts',(1.50642473211541E-11,-177.193984254242,
8.40164026751963));
#30924=CARTESIAN_POINT('Ctrl Pts',(4.85068927010183,-177.018984254242,8.40164026751099));
#30925=CARTESIAN_POINT('Ctrl Pts',(7.27603390513778,-176.843984254242,4.20082013374683));
#30926=CARTESIAN_POINT('Ctrl Pts',(9.70137854017372,-176.668984254242,-1.73424011235416E-11));
#30927=CARTESIAN_POINT('Ctrl Pts',(7.27603390512277,-176.493984254242,-4.20082013377284));
#30928=CARTESIAN_POINT('Ctrl Pts',(4.85068927007179,-176.318984254242,-8.40164026752833));
#30929=CARTESIAN_POINT('Ctrl Pts',(-1.49736725500596E-11,-176.143984254242,
-8.40164026751963));
#30930=CARTESIAN_POINT('Ctrl Pts',(-4.85068927010185,-175.968984254242,
-8.40164026751097));
#30931=CARTESIAN_POINT('Ctrl Pts',(-7.2760339051378,-175.793984254242,-4.2008201337468));
#30932=CARTESIAN_POINT('Ctrl Pts',(-9.70137854017372,-175.618984254242,
1.73756792675669E-11));
#30933=CARTESIAN_POINT('Ctrl Pts',(-7.27603390512275,-175.443984254242,
4.20082013377287));
#30934=CARTESIAN_POINT('Ctrl Pts',(-4.85068927007188,-175.268984254242,
8.40164026752828));
#30935=CARTESIAN_POINT('Ctrl Pts',(1.50024922681763E-11,-175.093984254242,
8.40164026751963));
#30936=CARTESIAN_POINT('Ctrl Pts',(4.85068927010188,-174.918984254242,8.40164026751095));
#30937=CARTESIAN_POINT('Ctrl Pts',(7.27603390513781,-174.743984254242,4.20082013374678));
#30938=CARTESIAN_POINT('Ctrl Pts',(9.70137854017372,-174.568984254242,-1.74089574115921E-11));
#30939=CARTESIAN_POINT('Ctrl Pts',(7.2760339051228,-174.393984254242,-4.20082013377279));
#30940=CARTESIAN_POINT('Ctrl Pts',(4.85068927007185,-174.218984254242,-8.4016402675283));
#30941=CARTESIAN_POINT('Ctrl Pts',(-1.50313119862929E-11,-174.043984254242,
-8.40164026751963));
#30942=CARTESIAN_POINT('Ctrl Pts',(-4.85068927010191,-173.868984254242,
-8.40164026751094));
#30943=CARTESIAN_POINT('Ctrl Pts',(-7.27603390513777,-173.693984254242,
-4.20082013374686));
#30944=CARTESIAN_POINT('Ctrl Pts',(-9.70137854017372,-173.518984254242,
1.73043706746458E-11));
#30945=CARTESIAN_POINT('Ctrl Pts',(-7.27603390512278,-173.343984254242,
4.20082013377282));
#30946=CARTESIAN_POINT('Ctrl Pts',(-4.85068927007182,-173.168984254242,
8.40164026752831));
#30947=CARTESIAN_POINT('Ctrl Pts',(1.50601317044096E-11,-172.993984254242,
8.40164026751963));
#30948=CARTESIAN_POINT('Ctrl Pts',(4.85068927010182,-172.818984254242,8.40164026751099));
#30949=CARTESIAN_POINT('Ctrl Pts',(7.27603390513778,-172.643984254242,4.20082013374683));
#30950=CARTESIAN_POINT('Ctrl Pts',(9.70137854017372,-172.468984254242,-1.7337648818671E-11));
#30951=CARTESIAN_POINT('Ctrl Pts',(7.27603390512277,-172.293984254242,-4.20082013377284));
#30952=CARTESIAN_POINT('Ctrl Pts',(4.85068927007179,-172.118984254242,-8.40164026752833));
#30953=CARTESIAN_POINT('Ctrl Pts',(-1.49695569333151E-11,-171.943984254242,
-8.40164026751963));
#30954=CARTESIAN_POINT('Ctrl Pts',(-4.85068927010185,-171.768984254242,
-8.40164026751097));
#30955=CARTESIAN_POINT('Ctrl Pts',(-7.2760339051378,-171.593984254242,-4.20082013374681));
#30956=CARTESIAN_POINT('Ctrl Pts',(-9.70137854017372,-171.418984254242,
1.73709269626963E-11));
#30957=CARTESIAN_POINT('Ctrl Pts',(-7.27603390512275,-171.243984254242,
4.20082013377287));
#30958=CARTESIAN_POINT('Ctrl Pts',(-4.85068927007176,-171.068984254242,
8.40164026752834));
#30959=CARTESIAN_POINT('Ctrl Pts',(1.49983766514318E-11,-170.893984254242,
8.40164026751963));
#30960=CARTESIAN_POINT('Ctrl Pts',(4.85068927010176,-170.718984254242,8.40164026751102));
#30961=CARTESIAN_POINT('Ctrl Pts',(7.27603390513781,-170.543984254242,4.20082013374678));
#30962=CARTESIAN_POINT('Ctrl Pts',(9.70137854017372,-170.368984254242,-1.72663402257499E-11));
#30963=CARTESIAN_POINT('Ctrl Pts',(7.27603390512274,-170.193984254242,-4.20082013377289));
#30964=CARTESIAN_POINT('Ctrl Pts',(4.85068927007186,-170.018984254242,-8.40164026752829));
#30965=CARTESIAN_POINT('Ctrl Pts',(-1.49078018803373E-11,-169.843984254242,
-8.40164026751963));
#30966=CARTESIAN_POINT('Ctrl Pts',(-4.85068927010191,-169.668984254242,
-8.40164026751094));
#30967=CARTESIAN_POINT('Ctrl Pts',(-7.27603390513777,-169.493984254242,
-4.20082013374686));
#30968=CARTESIAN_POINT('Ctrl Pts',(-9.70137854017372,-169.318984254242,
1.74374832507468E-11));
#30969=CARTESIAN_POINT('Ctrl Pts',(-7.27603390512278,-169.143984254242,
4.20082013377281));
#30970=CARTESIAN_POINT('Ctrl Pts',(-4.85068927007195,-168.968984254242,
8.40164026752824));
#30971=CARTESIAN_POINT('Ctrl Pts',(1.50560160876651E-11,-168.793984254242,
8.40164026751963));
#30972=CARTESIAN_POINT('Ctrl Pts',(4.85068927010182,-168.618984254242,8.40164026751099));
#30973=CARTESIAN_POINT('Ctrl Pts',(7.27603390513784,-168.443984254242,4.20082013374673));
#30974=CARTESIAN_POINT('Ctrl Pts',(9.70137854017372,-168.268984254242,-1.73328965138004E-11));
#30975=CARTESIAN_POINT('Ctrl Pts',(7.27603390512283,-168.093984254242,-4.20082013377273));
#30976=CARTESIAN_POINT('Ctrl Pts',(4.8506892700718,-167.918984254242,-8.40164026752832));
#30977=CARTESIAN_POINT('Ctrl Pts',(-1.49654413165707E-11,-167.743984254242,
-8.40164026751963));
#30978=CARTESIAN_POINT('Ctrl Pts',(-4.85068927010197,-167.568984254242,
-8.4016402675109));
#30979=CARTESIAN_POINT('Ctrl Pts',(-7.27603390513779,-167.393984254242,
-4.20082013374681));
#30980=CARTESIAN_POINT('Ctrl Pts',(-9.70137854017372,-167.218984254242,
1.72283097768541E-11));
#30981=CARTESIAN_POINT('Ctrl Pts',(-7.27603390512276,-167.043984254242,
4.20082013377286));
#30982=CARTESIAN_POINT('Ctrl Pts',(-4.85068927007189,-166.868984254242,
8.40164026752827));
#30983=CARTESIAN_POINT('Ctrl Pts',(1.51136555238984E-11,-166.693984254242,
8.40164026751963));
#30984=CARTESIAN_POINT('Ctrl Pts',(4.85068927010188,-166.518984254242,8.40164026751096));
#30985=CARTESIAN_POINT('Ctrl Pts',(7.27603390513775,-166.343984254242,4.20082013374689));
#30986=CARTESIAN_POINT('Ctrl Pts',(9.70137854017372,-166.168984254242,-1.73994528018509E-11));
#30987=CARTESIAN_POINT('Ctrl Pts',(7.2760339051228,-165.993984254242,-4.20082013377278));
#30988=CARTESIAN_POINT('Ctrl Pts',(4.85068927007198,-165.818984254242,-8.40164026752822));
#30989=CARTESIAN_POINT('Ctrl Pts',(-1.5023080752804E-11,-165.643984254242,
-8.40164026751963));
#30990=CARTESIAN_POINT('Ctrl Pts',(-4.85068927010179,-165.468984254242,
-8.40164026751101));
#30991=CARTESIAN_POINT('Ctrl Pts',(-7.27603390513782,-165.293984254242,
-4.20082013374676));
#30992=CARTESIAN_POINT('Ctrl Pts',(-9.70137854017372,-165.118984254242,
1.72948660649045E-11));
#30993=CARTESIAN_POINT('Ctrl Pts',(-7.27603390512285,-164.943984254242,
4.20082013377271));
#30994=CARTESIAN_POINT('Ctrl Pts',(-4.85068927007183,-164.768984254242,
8.40164026752831));
#30995=CARTESIAN_POINT('Ctrl Pts',(1.49325059817095E-11,-164.593984254242,
8.40164026751963));
#30996=CARTESIAN_POINT('Ctrl Pts',(4.85068927010193,-164.418984254242,8.40164026751092));
#30997=CARTESIAN_POINT('Ctrl Pts',(7.27603390513778,-164.243984254242,4.20082013374684));
#30998=CARTESIAN_POINT('Ctrl Pts',(9.70137854017372,-164.068984254242,-1.71902793279582E-11));
#30999=CARTESIAN_POINT('Ctrl Pts',(7.27603390512277,-163.893984254242,-4.20082013377283));
#31000=CARTESIAN_POINT('Ctrl Pts',(4.85068927007192,-163.718984254242,-8.40164026752825));
#31001=CARTESIAN_POINT('Ctrl Pts',(-1.50807201890373E-11,-163.543984254242,
-8.40164026751963));
#31002=CARTESIAN_POINT('Ctrl Pts',(-4.85068927010184,-163.368984254242,
-8.40164026751098));
#31003=CARTESIAN_POINT('Ctrl Pts',(-7.27603390513773,-163.193984254242,
-4.20082013374692));
#31004=CARTESIAN_POINT('Ctrl Pts',(-9.70137854017372,-163.018984254242,
1.7361422352955E-11));
#31005=CARTESIAN_POINT('Ctrl Pts',(-7.27603390512282,-162.843984254242,
4.20082013377275));
#31006=CARTESIAN_POINT('Ctrl Pts',(-4.85068927007177,-162.668984254242,
8.40164026752834));
#31007=CARTESIAN_POINT('Ctrl Pts',(1.49901454179428E-11,-162.493984254242,
8.40164026751963));
#31008=CARTESIAN_POINT('Ctrl Pts',(4.85068927010175,-162.318984254242,8.40164026751103));
#31009=CARTESIAN_POINT('Ctrl Pts',(7.27603390513781,-162.143984254242,4.20082013374679));
#31010=CARTESIAN_POINT('Ctrl Pts',(9.70137854017372,-161.968984254242,-1.72568356160087E-11));
#31011=CARTESIAN_POINT('Ctrl Pts',(7.27603390512274,-161.793984254242,-4.20082013377288));
#31012=CARTESIAN_POINT('Ctrl Pts',(4.85068927007186,-161.618984254242,-8.40164026752829));
#31013=CARTESIAN_POINT('Ctrl Pts',(-1.48995706468484E-11,-161.443984254242,
-8.40164026751963));
#31014=CARTESIAN_POINT('Ctrl Pts',(-4.8506892701019,-161.268984254242,-8.40164026751094));
#31015=CARTESIAN_POINT('Ctrl Pts',(-7.27603390513776,-161.093984254242,
-4.20082013374687));
#31016=CARTESIAN_POINT('Ctrl Pts',(-9.70137854017372,-160.918984254242,
1.74279786410055E-11));
#31017=CARTESIAN_POINT('Ctrl Pts',(-7.27603390512279,-160.743984254242,
4.2008201337728));
#31018=CARTESIAN_POINT('Ctrl Pts',(-4.85068927007195,-160.568984254242,
8.40164026752823));
#31019=CARTESIAN_POINT('Ctrl Pts',(1.50477848541761E-11,-160.393984254242,
8.40164026751963));
#31020=CARTESIAN_POINT('Ctrl Pts',(4.85068927010181,-160.218984254242,8.401640267511));
#31021=CARTESIAN_POINT('Ctrl Pts',(7.27603390513784,-160.043984254242,4.20082013374674));
#31022=CARTESIAN_POINT('Ctrl Pts',(9.70137854017372,-159.868984254242,-1.73233919040592E-11));
#31023=CARTESIAN_POINT('Ctrl Pts',(7.27603390512283,-159.693984254242,-4.20082013377273));
#31024=CARTESIAN_POINT('Ctrl Pts',(4.8506892700718,-159.518984254242,-8.40164026752832));
#31025=CARTESIAN_POINT('Ctrl Pts',(-1.49572100830817E-11,-159.343984254242,
-8.40164026751963));
#31026=CARTESIAN_POINT('Ctrl Pts',(-4.85068927010172,-159.168984254242,
-8.40164026751105));
#31027=CARTESIAN_POINT('Ctrl Pts',(-7.27603390513779,-158.993984254242,
-4.20082013374682));
#31028=CARTESIAN_POINT('Ctrl Pts',(-9.70137854017372,-158.818984254242,
1.72188051671128E-11));
#31029=CARTESIAN_POINT('Ctrl Pts',(-7.27603390512276,-158.643984254242,
4.20082013377285));
#31030=CARTESIAN_POINT('Ctrl Pts',(-4.8506892700719,-158.468984254242,8.40164026752827));
#31031=CARTESIAN_POINT('Ctrl Pts',(1.48666353119872E-11,-158.293984254242,
8.40164026751963));
#31032=CARTESIAN_POINT('Ctrl Pts',(4.85068927010187,-158.118984254242,8.40164026751096));
#31033=CARTESIAN_POINT('Ctrl Pts',(7.27603390513774,-157.943984254242,4.2008201337469));
#31034=CARTESIAN_POINT('Ctrl Pts',(9.70137854017372,-157.768984254242,-1.73899481921097E-11));
#31035=CARTESIAN_POINT('Ctrl Pts',(7.27603390512281,-157.593984254242,-4.20082013377278));
#31036=CARTESIAN_POINT('Ctrl Pts',(4.85068927007199,-157.418984254242,-8.40164026752822));
#31037=CARTESIAN_POINT('Ctrl Pts',(-1.5014849519315E-11,-157.243984254242,
-8.40164026751963));
#31038=CARTESIAN_POINT('Ctrl Pts',(-4.85068927010178,-157.068984254242,
-8.40164026751101));
#31039=CARTESIAN_POINT('Ctrl Pts',(-7.27603390513782,-156.893984254242,
-4.20082013374677));
#31040=CARTESIAN_POINT('Ctrl Pts',(-9.70137854017372,-156.718984254242,
1.72853614551633E-11));
#31041=CARTESIAN_POINT('Ctrl Pts',(-7.27603390512285,-156.543984254242,
4.2008201337727));
#31042=CARTESIAN_POINT('Ctrl Pts',(-4.85068927007184,-156.368984254242,
8.4016402675283));
#31043=CARTESIAN_POINT('Ctrl Pts',(1.49242747482206E-11,-156.193984254242,
8.40164026751963));
#31044=CARTESIAN_POINT('Ctrl Pts',(4.85068927010193,-156.018984254242,8.40164026751093));
#31045=CARTESIAN_POINT('Ctrl Pts',(7.27603390513778,-155.843984254242,4.20082013374685));
#31046=CARTESIAN_POINT('Ctrl Pts',(9.70137854017372,-155.668984254242,-1.7180774718217E-11));
#31047=CARTESIAN_POINT('Ctrl Pts',(7.27603390512277,-155.493984254242,-4.20082013377283));
#31048=CARTESIAN_POINT('Ctrl Pts',(4.85068927007193,-155.318984254242,-8.40164026752825));
#31049=CARTESIAN_POINT('Ctrl Pts',(-1.50724889555483E-11,-155.143984254242,
-8.40164026751963));
#31050=CARTESIAN_POINT('Ctrl Pts',(-4.85068927010184,-154.968984254242,
-8.40164026751098));
#31051=CARTESIAN_POINT('Ctrl Pts',(-7.27603390513773,-154.793984254242,
-4.20082013374692));
#31052=CARTESIAN_POINT('Ctrl Pts',(-9.70137854017372,-154.618984254242,
1.73519177432138E-11));
#31053=CARTESIAN_POINT('Ctrl Pts',(-7.27603390512282,-154.443984254242,
4.20082013377275));
#31054=CARTESIAN_POINT('Ctrl Pts',(-4.85068927007178,-154.268984254242,
8.40164026752833));
#31055=CARTESIAN_POINT('Ctrl Pts',(1.49819141844539E-11,-154.093984254242,
8.40164026751963));
#31056=CARTESIAN_POINT('Ctrl Pts',(4.85068927010175,-153.918984254242,8.40164026751103));
#31057=CARTESIAN_POINT('Ctrl Pts',(7.2760339051378,-153.743984254242,4.2008201337468));
#31058=CARTESIAN_POINT('Ctrl Pts',(9.70137854017372,-153.568984254242,-1.72473310062675E-11));
#31059=CARTESIAN_POINT('Ctrl Pts',(7.27603390512275,-153.393984254242,-4.20082013377288));
#31060=CARTESIAN_POINT('Ctrl Pts',(4.85068927007187,-153.218984254242,-8.40164026752828));
#31061=CARTESIAN_POINT('Ctrl Pts',(-1.48913394133594E-11,-153.043984254242,
-8.40164026751963));
#31062=CARTESIAN_POINT('Ctrl Pts',(-4.85068927010189,-152.868984254242,
-8.40164026751095));
#31063=CARTESIAN_POINT('Ctrl Pts',(-7.27603390513776,-152.693984254242,
-4.20082013374688));
#31064=CARTESIAN_POINT('Ctrl Pts',(-9.70137854017372,-152.518984254242,
1.71427442693211E-11));
#31065=CARTESIAN_POINT('Ctrl Pts',(-7.27603390512279,-152.343984254242,
4.2008201337728));
#31066=CARTESIAN_POINT('Ctrl Pts',(-4.85068927007196,-152.168984254242,
8.40164026752823));
#31067=CARTESIAN_POINT('Ctrl Pts',(1.50395536206872E-11,-151.993984254242,
8.40164026751963));
#31068=CARTESIAN_POINT('Ctrl Pts',(4.8506892701018,-151.818984254242,8.401640267511));
#31069=CARTESIAN_POINT('Ctrl Pts',(7.27603390513771,-151.643984254242,4.20082013374695));
#31070=CARTESIAN_POINT('Ctrl Pts',(9.70137854017372,-151.468984254242,-1.73138872943179E-11));
#31071=CARTESIAN_POINT('Ctrl Pts',(7.27603390512284,-151.293984254242,-4.20082013377272));
#31072=CARTESIAN_POINT('Ctrl Pts',(4.85068927007181,-151.118984254242,-8.40164026752832));
#31073=CARTESIAN_POINT('Ctrl Pts',(-1.49489788495927E-11,-150.943984254242,
-8.40164026751963));
#31074=CARTESIAN_POINT('Ctrl Pts',(-4.85068927010171,-150.768984254242,
-8.40164026751105));
#31075=CARTESIAN_POINT('Ctrl Pts',(-7.27603390513779,-150.593984254242,
-4.20082013374683));
#31076=CARTESIAN_POINT('Ctrl Pts',(-9.70137854017372,-150.418984254242,
1.72093005573716E-11));
#31077=CARTESIAN_POINT('Ctrl Pts',(-7.27603390512276,-150.243984254242,
4.20082013377285));
#31078=CARTESIAN_POINT('Ctrl Pts',(-4.8506892700719,-150.068984254242,8.40164026752826));
#31079=CARTESIAN_POINT('Ctrl Pts',(1.48584040784983E-11,-149.893984254242,
8.40164026751963));
#31080=CARTESIAN_POINT('Ctrl Pts',(4.85068927010186,-149.718984254242,8.40164026751097));
#31081=CARTESIAN_POINT('Ctrl Pts',(7.27603390513774,-149.543984254242,4.2008201337469));
#31082=CARTESIAN_POINT('Ctrl Pts',(9.70137854017372,-149.368984254242,-1.73804435823684E-11));
#31083=CARTESIAN_POINT('Ctrl Pts',(7.27603390512281,-149.193984254242,-4.20082013377277));
#31084=CARTESIAN_POINT('Ctrl Pts',(4.85068927007199,-149.018984254242,-8.40164026752821));
#31085=CARTESIAN_POINT('Ctrl Pts',(-1.5006618285826E-11,-148.843984254242,
-8.40164026751963));
#31086=CARTESIAN_POINT('Ctrl Pts',(-4.85068927010177,-148.668984254242,
-8.40164026751102));
#31087=CARTESIAN_POINT('Ctrl Pts',(-7.27603390513782,-148.493984254242,
-4.20082013374678));
#31088=CARTESIAN_POINT('Ctrl Pts',(-9.70137854017372,-148.318984254242,
1.72758568454221E-11));
#31089=CARTESIAN_POINT('Ctrl Pts',(-7.27603390512285,-148.143984254242,
4.20082013377269));
#31090=CARTESIAN_POINT('Ctrl Pts',(-4.85068927007185,-147.968984254242,
8.4016402675283));
#31091=CARTESIAN_POINT('Ctrl Pts',(1.49160435147316E-11,-147.793984254242,
8.40164026751963));
#31092=CARTESIAN_POINT('Ctrl Pts',(4.85068927010192,-147.618984254242,8.40164026751093));
#31093=CARTESIAN_POINT('Ctrl Pts',(7.27603390513777,-147.443984254242,4.20082013374685));
#31094=CARTESIAN_POINT('Ctrl Pts',(9.70137854017372,-147.268984254242,-1.71712701084757E-11));
#31095=CARTESIAN_POINT('Ctrl Pts',(7.27603390512278,-147.093984254242,-4.20082013377282));
#31096=CARTESIAN_POINT('Ctrl Pts',(4.85068927007194,-146.918984254242,-8.40164026752825));
#31097=CARTESIAN_POINT('Ctrl Pts',(-1.50642577220594E-11,-146.743984254242,
-8.40164026751963));
#31098=CARTESIAN_POINT('Ctrl Pts',(-4.85068927010183,-146.568984254242,
-8.40164026751099));
#31099=CARTESIAN_POINT('Ctrl Pts',(-7.27603390513773,-146.393984254242,
-4.20082013374693));
#31100=CARTESIAN_POINT('Ctrl Pts',(-9.70137854017372,-146.218984254242,
1.73424131334726E-11));
#31101=CARTESIAN_POINT('Ctrl Pts',(-7.27603390512282,-146.043984254242,
4.20082013377274));
#31102=CARTESIAN_POINT('Ctrl Pts',(-4.85068927007203,-145.868984254242,
8.40164026752819));
#31103=CARTESIAN_POINT('Ctrl Pts',(1.49736829509649E-11,-145.693984254242,
8.40164026751963));
#31104=CARTESIAN_POINT('Ctrl Pts',(4.85068927010174,-145.518984254242,8.40164026751104));
#31105=CARTESIAN_POINT('Ctrl Pts',(7.2760339051378,-145.343984254242,4.2008201337468));
#31106=CARTESIAN_POINT('Ctrl Pts',(9.70137854017372,-145.168984254242,-1.72378263965262E-11));
#31107=CARTESIAN_POINT('Ctrl Pts',(7.27603390512287,-144.993984254242,-4.20082013377266));
#31108=CARTESIAN_POINT('Ctrl Pts',(4.85068927007188,-144.818984254242,-8.40164026752828));
#31109=CARTESIAN_POINT('Ctrl Pts',(-1.48831081798705E-11,-144.643984254242,
-8.40164026751963));
#31110=CARTESIAN_POINT('Ctrl Pts',(-4.85068927010188,-144.468984254242,
-8.40164026751095));
#31111=CARTESIAN_POINT('Ctrl Pts',(-7.27603390513775,-144.293984254242,
-4.20082013374688));
#31112=CARTESIAN_POINT('Ctrl Pts',(-9.70137854017372,-144.118984254242,
1.71332396595799E-11));
#31113=CARTESIAN_POINT('Ctrl Pts',(-7.2760339051228,-143.943984254242,4.20082013377279));
#31114=CARTESIAN_POINT('Ctrl Pts',(-4.85068927007197,-143.768984254242,
8.40164026752823));
#31115=CARTESIAN_POINT('Ctrl Pts',(1.50313223871982E-11,-143.593984254242,
8.40164026751963));
#31116=CARTESIAN_POINT('Ctrl Pts',(4.85068927010179,-143.418984254242,8.401640267511));
#31117=CARTESIAN_POINT('Ctrl Pts',(7.27603390513771,-143.243984254242,4.20082013374696));
#31118=CARTESIAN_POINT('Ctrl Pts',(9.70137854017372,-143.068984254242,-1.73043826845767E-11));
#31119=CARTESIAN_POINT('Ctrl Pts',(7.27603390512284,-142.893984254242,-4.20082013377271));
#31120=CARTESIAN_POINT('Ctrl Pts',(4.85068927007182,-142.718984254242,-8.40164026752831));
#31121=CARTESIAN_POINT('Ctrl Pts',(-1.49407476161038E-11,-142.543984254242,
-8.40164026751963));
#31122=CARTESIAN_POINT('Ctrl Pts',(-4.8506892701017,-142.368984254242,-8.40164026751106));
#31123=CARTESIAN_POINT('Ctrl Pts',(-7.27603390513778,-142.193984254242,
-4.20082013374683));
#31124=CARTESIAN_POINT('Ctrl Pts',(-9.70137854017372,-142.018984254242,
1.71997959476304E-11));
#31125=CARTESIAN_POINT('Ctrl Pts',(-7.27603390512277,-141.843984254242,
4.20082013377284));
#31126=CARTESIAN_POINT('Ctrl Pts',(-4.85068927007191,-141.668984254242,
8.40164026752826));
#31127=CARTESIAN_POINT('Ctrl Pts',(1.48501728450093E-11,-141.493984254242,
8.40164026751963));
#31128=CARTESIAN_POINT('Ctrl Pts',(4.85068927010185,-141.318984254242,8.40164026751097));
#31129=CARTESIAN_POINT('Ctrl Pts',(7.27603390513774,-141.143984254242,4.20082013374691));
#31130=CARTESIAN_POINT('Ctrl Pts',(9.70137854017372,-140.968984254242,-1.73709389726272E-11));
#31131=CARTESIAN_POINT('Ctrl Pts',(7.27603390512281,-140.793984254242,-4.20082013377276));
#31132=CARTESIAN_POINT('Ctrl Pts',(4.850689270072,-140.618984254242,-8.40164026752821));
#31133=CARTESIAN_POINT('Ctrl Pts',(-1.49983870523371E-11,-140.443984254242,
-8.40164026751963));
#31134=CARTESIAN_POINT('Ctrl Pts',(-4.85068927010176,-140.268984254242,
-8.40164026751102));
#31135=CARTESIAN_POINT('Ctrl Pts',(-7.27603390513769,-140.093984254242,
-4.20082013374699));
#31136=CARTESIAN_POINT('Ctrl Pts',(-9.70137854017372,-139.918984254242,
1.72663522356809E-11));
#31137=CARTESIAN_POINT('Ctrl Pts',(-7.27603390512286,-139.743984254242,
4.20082013377268));
#31138=CARTESIAN_POINT('Ctrl Pts',(-4.85068927007186,-139.568984254242,
8.40164026752829));
#31139=CARTESIAN_POINT('Ctrl Pts',(1.49078122812426E-11,-139.393984254242,
8.40164026751963));
#31140=CARTESIAN_POINT('Ctrl Pts',(4.85068927010167,-139.218984254242,8.40164026751108));
#31141=CARTESIAN_POINT('Ctrl Pts',(7.27603390513777,-139.043984254242,4.20082013374686));
#31142=CARTESIAN_POINT('Ctrl Pts',(9.70137854017372,-138.868984254242,-1.71617654987345E-11));
#31143=CARTESIAN_POINT('Ctrl Pts',(7.27603390512278,-138.693984254242,-4.20082013377281));
#31144=CARTESIAN_POINT('Ctrl Pts',(4.85068927007195,-138.518984254242,-8.40164026752824));
#31145=CARTESIAN_POINT('Ctrl Pts',(-1.48172375101482E-11,-138.343984254242,
-8.40164026751963));
#31146=CARTESIAN_POINT('Ctrl Pts',(-4.85068927010182,-138.168984254242,
-8.40164026751099));
#31147=CARTESIAN_POINT('Ctrl Pts',(-7.27603390513772,-137.993984254242,
-4.20082013374694));
#31148=CARTESIAN_POINT('Ctrl Pts',(-9.70137854017372,-137.818984254242,
1.73329085237313E-11));
#31149=CARTESIAN_POINT('Ctrl Pts',(-7.27603390512283,-137.643984254242,
4.20082013377273));
#31150=CARTESIAN_POINT('Ctrl Pts',(-4.85068927007204,-137.468984254242,
8.40164026752819));
#31151=CARTESIAN_POINT('Ctrl Pts',(1.49654517174759E-11,-137.293984254242,
8.40164026751963));
#31152=CARTESIAN_POINT('Ctrl Pts',(4.85068927010173,-137.118984254242,8.40164026751104));
#31153=CARTESIAN_POINT('Ctrl Pts',(7.27603390513779,-136.943984254242,4.20082013374681));
#31154=CARTESIAN_POINT('Ctrl Pts',(9.70137854017372,-136.768984254242,-1.7228321786785E-11));
#31155=CARTESIAN_POINT('Ctrl Pts',(7.27603390512287,-136.593984254242,-4.20082013377265));
#31156=CARTESIAN_POINT('Ctrl Pts',(4.85068927007189,-136.418984254242,-8.40164026752827));
#31157=CARTESIAN_POINT('Ctrl Pts',(-1.48748769463815E-11,-136.243984254242,
-8.40164026751963));
#31158=CARTESIAN_POINT('Ctrl Pts',(-4.85068927010188,-136.068984254242,
-8.40164026751096));
#31159=CARTESIAN_POINT('Ctrl Pts',(-7.27603390513775,-135.893984254242,
-4.20082013374689));
#31160=CARTESIAN_POINT('Ctrl Pts',(-9.70137854017372,-135.718984254242,
1.71237350498386E-11));
#31161=CARTESIAN_POINT('Ctrl Pts',(-7.2760339051228,-135.543984254242,4.20082013377278));
#31162=CARTESIAN_POINT('Ctrl Pts',(-4.85068927007198,-135.368984254242,
8.40164026752822));
#31163=CARTESIAN_POINT('Ctrl Pts',(1.50230911537093E-11,-135.193984254242,
8.40164026751963));
#31164=CARTESIAN_POINT('Ctrl Pts',(4.85068927010179,-135.018984254242,8.40164026751101));
#31165=CARTESIAN_POINT('Ctrl Pts',(7.2760339051377,-134.843984254242,4.20082013374697));
#31166=CARTESIAN_POINT('Ctrl Pts',(9.70137854017372,-134.668984254242,-1.72948780748355E-11));
#31167=CARTESIAN_POINT('Ctrl Pts',(7.27603390512285,-134.493984254242,-4.20082013377271));
#31168=CARTESIAN_POINT('Ctrl Pts',(4.85068927007183,-134.318984254242,-8.40164026752831));
#31169=CARTESIAN_POINT('Ctrl Pts',(-1.49325163826148E-11,-134.143984254242,
-8.40164026751963));
#31170=CARTESIAN_POINT('Ctrl Pts',(-4.85068927010169,-133.968984254242,
-8.40164026751106));
#31171=CARTESIAN_POINT('Ctrl Pts',(-7.27603390513778,-133.793984254242,
-4.20082013374684));
#31172=CARTESIAN_POINT('Ctrl Pts',(-9.70137854017372,-133.618984254242,
1.71902913378891E-11));
#31173=CARTESIAN_POINT('Ctrl Pts',(-7.27603390512289,-133.443984254242,
4.20082013377263));
#31174=CARTESIAN_POINT('Ctrl Pts',(-4.85068927007192,-133.268984254242,
8.40164026752825));
#31175=CARTESIAN_POINT('Ctrl Pts',(1.48419416115203E-11,-133.093984254242,
8.40164026751963));
#31176=CARTESIAN_POINT('Ctrl Pts',(4.85068927010184,-132.918984254242,8.40164026751098));
#31177=CARTESIAN_POINT('Ctrl Pts',(7.27603390513773,-132.743984254242,4.20082013374692));
#31178=CARTESIAN_POINT('Ctrl Pts',(9.70137854017372,-132.568984254242,-1.70857046009428E-11));
#31179=CARTESIAN_POINT('Ctrl Pts',(7.27603390512282,-132.393984254242,-4.20082013377275));
#31180=CARTESIAN_POINT('Ctrl Pts',(4.85068927007201,-132.218984254242,-8.4016402675282));
#31181=CARTESIAN_POINT('Ctrl Pts',(-1.49901558188481E-11,-132.043984254242,
-8.40164026751963));
#31182=CARTESIAN_POINT('Ctrl Pts',(-4.85068927010175,-131.868984254242,
-8.40164026751103));
#31183=CARTESIAN_POINT('Ctrl Pts',(-7.27603390513769,-131.693984254242,
-4.200820133747));
#31184=CARTESIAN_POINT('Ctrl Pts',(-9.70137854017372,-131.518984254242,
1.72568476259396E-11));
#31185=CARTESIAN_POINT('Ctrl Pts',(-7.27603390512286,-131.343984254242,
4.20082013377267));
#31186=CARTESIAN_POINT('Ctrl Pts',(-4.85068927007186,-131.168984254242,
8.40164026752829));
#31187=CARTESIAN_POINT('Ctrl Pts',(1.48995810477537E-11,-130.993984254242,
8.40164026751963));
#31188=CARTESIAN_POINT('Ctrl Pts',(4.85068927010166,-130.818984254242,8.40164026751108));
#31189=CARTESIAN_POINT('Ctrl Pts',(7.27603390513776,-130.643984254242,4.20082013374687));
#31190=CARTESIAN_POINT('Ctrl Pts',(9.70137854017372,-130.468984254242,-1.71522608889933E-11));
#31191=CARTESIAN_POINT('Ctrl Pts',(7.27603390512279,-130.293984254242,-4.2008201337728));
#31192=CARTESIAN_POINT('Ctrl Pts',(4.85068927007195,-130.118984254242,-8.40164026752823));
#31193=CARTESIAN_POINT('Ctrl Pts',(-1.48090062766592E-11,-129.943984254242,
-8.40164026751963));
#31194=CARTESIAN_POINT('Ctrl Pts',(-4.85068927010181,-129.768984254242,
-8.401640267511));
#31195=CARTESIAN_POINT('Ctrl Pts',(-7.27603390513772,-129.593984254242,
-4.20082013374695));
#31196=CARTESIAN_POINT('Ctrl Pts',(-9.70137854017372,-129.418984254242,
1.73234039139901E-11));
#31197=CARTESIAN_POINT('Ctrl Pts',(-7.27603390512283,-129.243984254242,
4.20082013377273));
#31198=CARTESIAN_POINT('Ctrl Pts',(-4.85068927007204,-129.068984254242,
8.40164026752818));
#31199=CARTESIAN_POINT('Ctrl Pts',(1.4957220483987E-11,-128.893984254242,
8.40164026751963));
#31200=CARTESIAN_POINT('Ctrl Pts',(4.85068927010172,-128.718984254242,8.40164026751105));
#31201=CARTESIAN_POINT('Ctrl Pts',(7.27603390513779,-128.543984254242,4.20082013374682));
#31202=CARTESIAN_POINT('Ctrl Pts',(9.70137854017372,-128.368984254242,-1.72188171770438E-11));
#31203=CARTESIAN_POINT('Ctrl Pts',(7.27603390512276,-128.193984254242,-4.20082013377285));
#31204=CARTESIAN_POINT('Ctrl Pts',(4.85068927007213,-128.018984254242,-8.40164026752813));
#31205=CARTESIAN_POINT('Ctrl Pts',(-1.48666457128925E-11,-127.843984254242,
-8.40164026751963));
#31206=CARTESIAN_POINT('Ctrl Pts',(-4.85068927010187,-127.668984254242,
-8.40164026751096));
#31207=CARTESIAN_POINT('Ctrl Pts',(-7.27603390513763,-127.493984254242,
-4.2008201337471));
#31208=CARTESIAN_POINT('Ctrl Pts',(-9.70137854017372,-127.318984254242,
1.71142304400974E-11));
#31209=CARTESIAN_POINT('Ctrl Pts',(-7.27603390512281,-127.143984254242,
4.20082013377278));
#31210=CARTESIAN_POINT('Ctrl Pts',(-4.85068927007175,-126.968984254242,
8.40164026752835));
#31211=CARTESIAN_POINT('Ctrl Pts',(1.47760709417981E-11,-126.793984254242,
8.40164026751963));
#31212=CARTESIAN_POINT('Ctrl Pts',(4.85068927010178,-126.618984254242,8.40164026751101));
#31213=CARTESIAN_POINT('Ctrl Pts',(7.27603390513782,-126.443984254242,4.20082013374677));
#31214=CARTESIAN_POINT('Ctrl Pts',(9.70137854017372,-126.268984254242,-1.70096437031511E-11));
#31215=CARTESIAN_POINT('Ctrl Pts',(7.27603390512285,-126.093984254242,-4.2008201337727));
#31216=CARTESIAN_POINT('Ctrl Pts',(4.85068927007184,-125.918984254242,-8.4016402675283));
#31217=CARTESIAN_POINT('Ctrl Pts',(-1.46854961707036E-11,-125.743984254242,
-8.40164026751963));
#31218=CARTESIAN_POINT('Ctrl Pts',(-4.85068927010169,-125.568984254242,
-8.40164026751107));
#31219=CARTESIAN_POINT('Ctrl Pts',(-7.27603390513778,-125.393984254242,
-4.20082013374685));
#31220=CARTESIAN_POINT('Ctrl Pts',(-9.70137854017372,-125.218984254242,
1.74565164900911E-11));
#31221=CARTESIAN_POINT('Ctrl Pts',(-7.27603390512289,-125.043984254242,
4.20082013377262));
#31222=CARTESIAN_POINT('Ctrl Pts',(-4.85068927007193,-124.868984254242,
8.40164026752825));
#31223=CARTESIAN_POINT('Ctrl Pts',(1.50724993564536E-11,-124.693984254242,
8.40164026751963));
#31224=CARTESIAN_POINT('Ctrl Pts',(4.8506892701016,-124.518984254242,8.40164026751112));
#31225=CARTESIAN_POINT('Ctrl Pts',(7.27603390513773,-124.343984254242,4.20082013374692));
#31226=CARTESIAN_POINT('Ctrl Pts',(9.70137854017372,-124.168984254242,-1.73519297531447E-11));
#31227=CARTESIAN_POINT('Ctrl Pts',(7.27603390512294,-123.993984254242,-4.20082013377254));
#31228=CARTESIAN_POINT('Ctrl Pts',(4.85068927007202,-123.818984254242,-8.4016402675282));
#31229=CARTESIAN_POINT('Ctrl Pts',(-1.49819245853592E-11,-123.643984254242,
-8.40164026751963));
#31230=CARTESIAN_POINT('Ctrl Pts',(-4.85068927010151,-123.468984254242,
-8.40164026751117));
#31231=CARTESIAN_POINT('Ctrl Pts',(-7.27603390513768,-123.293984254242,
-4.200820133747));
#31232=CARTESIAN_POINT('Ctrl Pts',(-9.70137854017372,-123.118984254242,
1.72473430161984E-11));
#31233=CARTESIAN_POINT('Ctrl Pts',(-7.27603390512275,-122.943984254242,
4.20082013377288));
#31234=CARTESIAN_POINT('Ctrl Pts',(-4.85068927007211,-122.768984254242,
8.40164026752814));
#31235=CARTESIAN_POINT('Ctrl Pts',(1.48913498142647E-11,-122.593984254242,
8.40164026751963));
#31236=CARTESIAN_POINT('Ctrl Pts',(4.85068927010189,-122.418984254242,8.40164026751095));
#31237=CARTESIAN_POINT('Ctrl Pts',(7.27603390513764,-122.243984254242,4.20082013374708));
#31238=CARTESIAN_POINT('Ctrl Pts',(9.70137854017372,-122.068984254242,-1.7142756279252E-11));
#31239=CARTESIAN_POINT('Ctrl Pts',(7.27603390512279,-121.893984254242,-4.2008201337728));
#31240=CARTESIAN_POINT('Ctrl Pts',(4.8506892700722,-121.718984254242,-8.40164026752809));
#31241=CARTESIAN_POINT('Ctrl Pts',(-1.48007750431702E-11,-121.543984254242,
-8.40164026751963));
#31242=CARTESIAN_POINT('Ctrl Pts',(-4.8506892701018,-121.368984254242,-8.401640267511));
#31243=CARTESIAN_POINT('Ctrl Pts',(-7.27603390513783,-121.193984254242,
-4.20082013374675));
#31244=CARTESIAN_POINT('Ctrl Pts',(-9.70137854017372,-121.018984254242,
1.70381695423057E-11));
#31245=CARTESIAN_POINT('Ctrl Pts',(-7.27603390512284,-120.843984254242,
4.20082013377272));
#31246=CARTESIAN_POINT('Ctrl Pts',(-4.85068927007181,-120.668984254242,
8.40164026752832));
#31247=CARTESIAN_POINT('Ctrl Pts',(1.47102002720758E-11,-120.493984254242,
8.40164026751963));
#31248=CARTESIAN_POINT('Ctrl Pts',(4.85068927010171,-120.318984254242,8.40164026751105));
#31249=CARTESIAN_POINT('Ctrl Pts',(7.27603390513779,-120.143984254242,4.20082013374683));
#31250=CARTESIAN_POINT('Ctrl Pts',(9.70137854017372,-119.968984254242,-1.69335828053594E-11));
#31251=CARTESIAN_POINT('Ctrl Pts',(7.27603390512288,-119.793984254242,-4.20082013377264));
#31252=CARTESIAN_POINT('Ctrl Pts',(4.8506892700719,-119.618984254242,-8.40164026752826));
#31253=CARTESIAN_POINT('Ctrl Pts',(-1.50972034578258E-11,-119.443984254242,
-8.40164026751963));
#31254=CARTESIAN_POINT('Ctrl Pts',(-4.85068927010162,-119.268984254242,
-8.40164026751111));
#31255=CARTESIAN_POINT('Ctrl Pts',(-7.27603390513774,-119.093984254242,
-4.2008201337469));
#31256=CARTESIAN_POINT('Ctrl Pts',(-9.70137854017372,-118.918984254242,
1.73804555922994E-11));
#31257=CARTESIAN_POINT('Ctrl Pts',(-7.27603390512293,-118.743984254242,
4.20082013377256));
#31258=CARTESIAN_POINT('Ctrl Pts',(-4.85068927007199,-118.568984254242,
8.40164026752821));
#31259=CARTESIAN_POINT('Ctrl Pts',(1.50066286867313E-11,-118.393984254242,
8.40164026751963));
#31260=CARTESIAN_POINT('Ctrl Pts',(4.85068927010153,-118.218984254242,8.40164026751116));
#31261=CARTESIAN_POINT('Ctrl Pts',(7.2760339051377,-118.043984254242,4.20082013374698));
#31262=CARTESIAN_POINT('Ctrl Pts',(9.70137854017372,-117.868984254242,-1.7275868855353E-11));
#31263=CARTESIAN_POINT('Ctrl Pts',(7.27603390512297,-117.693984254242,-4.20082013377248));
#31264=CARTESIAN_POINT('Ctrl Pts',(4.85068927007208,-117.518984254242,-8.40164026752816));
#31265=CARTESIAN_POINT('Ctrl Pts',(-1.49160539156369E-11,-117.343984254242,
-8.40164026751963));
#31266=CARTESIAN_POINT('Ctrl Pts',(-4.85068927010192,-117.168984254242,
-8.40164026751093));
#31267=CARTESIAN_POINT('Ctrl Pts',(-7.27603390513765,-116.993984254242,
-4.20082013374706));
#31268=CARTESIAN_POINT('Ctrl Pts',(-9.70137854017372,-116.818984254242,
1.71712821184067E-11));
#31269=CARTESIAN_POINT('Ctrl Pts',(-7.27603390512278,-116.643984254242,
4.20082013377282));
#31270=CARTESIAN_POINT('Ctrl Pts',(-4.85068927007218,-116.468984254242,
8.40164026752811));
#31271=CARTESIAN_POINT('Ctrl Pts',(1.48254791445424E-11,-116.293984254242,
8.40164026751963));
#31272=CARTESIAN_POINT('Ctrl Pts',(4.85068927010183,-116.118984254242,8.40164026751099));
#31273=CARTESIAN_POINT('Ctrl Pts',(7.27603390513761,-115.943984254242,4.20082013374714));
#31274=CARTESIAN_POINT('Ctrl Pts',(9.70137854017372,-115.768984254242,-1.70666953814603E-11));
#31275=CARTESIAN_POINT('Ctrl Pts',(7.27603390512282,-115.593984254242,-4.20082013377274));
#31276=CARTESIAN_POINT('Ctrl Pts',(4.85068927007179,-115.418984254242,-8.40164026752833));
#31277=CARTESIAN_POINT('Ctrl Pts',(-1.4734904373448E-11,-115.243984254242,
-8.40164026751963));
#31278=CARTESIAN_POINT('Ctrl Pts',(-4.85068927010174,-115.068984254242,
-8.40164026751104));
#31279=CARTESIAN_POINT('Ctrl Pts',(-7.2760339051378,-114.893984254242,-4.2008201337468));
#31280=CARTESIAN_POINT('Ctrl Pts',(-9.70137854017372,-114.718984254242,
1.6962108644514E-11));
#31281=CARTESIAN_POINT('Ctrl Pts',(-7.27603390512287,-114.543984254242,
4.20082013377266));
#31282=CARTESIAN_POINT('Ctrl Pts',(-4.85068927007188,-114.368984254242,
8.40164026752828));
#31283=CARTESIAN_POINT('Ctrl Pts',(1.46443296023535E-11,-114.193984254242,
8.40164026751963));
#31284=CARTESIAN_POINT('Ctrl Pts',(4.85068927010165,-114.018984254242,8.40164026751109));
#31285=CARTESIAN_POINT('Ctrl Pts',(7.27603390513775,-113.843984254242,4.20082013374688));
#31286=CARTESIAN_POINT('Ctrl Pts',(9.70137854017372,-113.668984254242,-1.7408981431454E-11));
#31287=CARTESIAN_POINT('Ctrl Pts',(7.27603390512292,-113.493984254242,-4.20082013377258));
#31288=CARTESIAN_POINT('Ctrl Pts',(4.85068927007197,-113.318984254242,-8.40164026752823));
#31289=CARTESIAN_POINT('Ctrl Pts',(-1.50313327881035E-11,-113.143984254242,
-8.40164026751963));
#31290=CARTESIAN_POINT('Ctrl Pts',(-4.85068927010155,-112.968984254242,
-8.40164026751114));
#31291=CARTESIAN_POINT('Ctrl Pts',(-7.27603390513771,-112.793984254242,
-4.20082013374696));
#31292=CARTESIAN_POINT('Ctrl Pts',(-9.70137854017372,-112.618984254242,
1.73043946945076E-11));
#31293=CARTESIAN_POINT('Ctrl Pts',(-7.27603390512296,-112.443984254242,
4.2008201337725));
#31294=CARTESIAN_POINT('Ctrl Pts',(-4.85068927007206,-112.268984254242,
8.40164026752817));
#31295=CARTESIAN_POINT('Ctrl Pts',(1.49407580170091E-11,-112.093984254242,
8.40164026751963));
#31296=CARTESIAN_POINT('Ctrl Pts',(4.85068927010194,-111.918984254242,8.40164026751092));
#31297=CARTESIAN_POINT('Ctrl Pts',(7.27603390513766,-111.743984254242,4.20082013374704));
#31298=CARTESIAN_POINT('Ctrl Pts',(9.70137854017372,-111.568984254242,-1.71998079575613E-11));
#31299=CARTESIAN_POINT('Ctrl Pts',(7.27603390512277,-111.393984254242,-4.20082013377284));
#31300=CARTESIAN_POINT('Ctrl Pts',(4.85068927007215,-111.218984254242,-8.40164026752812));
#31301=CARTESIAN_POINT('Ctrl Pts',(-1.48501832459146E-11,-111.043984254242,
-8.40164026751963));
#31302=CARTESIAN_POINT('Ctrl Pts',(-4.85068927010185,-110.868984254242,
-8.40164026751097));
#31303=CARTESIAN_POINT('Ctrl Pts',(-7.27603390513762,-110.693984254242,
-4.20082013374712));
#31304=CARTESIAN_POINT('Ctrl Pts',(-9.70137854017372,-110.518984254242,
1.7095221220615E-11));
#31305=CARTESIAN_POINT('Ctrl Pts',(-7.27603390512281,-110.343984254242,
4.20082013377276));
#31306=CARTESIAN_POINT('Ctrl Pts',(-4.85068927007224,-110.168984254242,
8.40164026752807));
#31307=CARTESIAN_POINT('Ctrl Pts',(1.47596084748201E-11,-109.993984254242,
8.40164026751963));
#31308=CARTESIAN_POINT('Ctrl Pts',(4.85068927010176,-109.818984254242,8.40164026751102));
#31309=CARTESIAN_POINT('Ctrl Pts',(7.27603390513781,-109.643984254242,4.20082013374678));
#31310=CARTESIAN_POINT('Ctrl Pts',(9.70137854017372,-109.468984254242,-1.69906344836686E-11));
#31311=CARTESIAN_POINT('Ctrl Pts',(7.27603390512286,-109.293984254242,-4.20082013377268));
#31312=CARTESIAN_POINT('Ctrl Pts',(4.85068927007186,-109.118984254242,-8.40164026752829));
#31313=CARTESIAN_POINT('Ctrl Pts',(-1.46690337037257E-11,-108.943984254242,
-8.40164026751963));
#31314=CARTESIAN_POINT('Ctrl Pts',(-4.85068927010167,-108.768984254242,
-8.40164026751108));
#31315=CARTESIAN_POINT('Ctrl Pts',(-7.27603390513777,-108.593984254242,
-4.20082013374686));
#31316=CARTESIAN_POINT('Ctrl Pts',(-9.70137854017372,-108.418984254242,
1.68860477467223E-11));
#31317=CARTESIAN_POINT('Ctrl Pts',(-7.2760339051229,-108.243984254242,4.2008201337726));
#31318=CARTESIAN_POINT('Ctrl Pts',(-4.85068927007195,-108.068984254242,
8.40164026752824));
#31319=CARTESIAN_POINT('Ctrl Pts',(1.50560368894757E-11,-107.893984254242,
8.40164026751963));
#31320=CARTESIAN_POINT('Ctrl Pts',(4.85068927010158,-107.718984254242,8.40164026751113));
#31321=CARTESIAN_POINT('Ctrl Pts',(7.27603390513772,-107.543984254242,4.20082013374694));
#31322=CARTESIAN_POINT('Ctrl Pts',(9.70137854017372,-107.368984254242,-1.73329205336623E-11));
#31323=CARTESIAN_POINT('Ctrl Pts',(7.27603390512295,-107.193984254242,-4.20082013377253));
#31324=CARTESIAN_POINT('Ctrl Pts',(4.85068927007204,-107.018984254242,-8.40164026752819));
#31325=CARTESIAN_POINT('Ctrl Pts',(-1.49654621183812E-11,-106.843984254242,
-8.40164026751963));
#31326=CARTESIAN_POINT('Ctrl Pts',(-4.85068927010149,-106.668984254242,
-8.40164026751118));
#31327=CARTESIAN_POINT('Ctrl Pts',(-7.27603390513768,-106.493984254242,
-4.20082013374702));
#31328=CARTESIAN_POINT('Ctrl Pts',(-9.70137854017372,-106.318984254242,
1.72283337967159E-11));
#31329=CARTESIAN_POINT('Ctrl Pts',(-7.27603390512276,-106.143984254242,
4.20082013377286));
#31330=CARTESIAN_POINT('Ctrl Pts',(-4.85068927007213,-105.968984254242,
8.40164026752814));
#31331=CARTESIAN_POINT('Ctrl Pts',(1.48748873472868E-11,-105.793984254242,
8.40164026751963));
#31332=CARTESIAN_POINT('Ctrl Pts',(4.85068927010188,-105.618984254242,8.40164026751096));
#31333=CARTESIAN_POINT('Ctrl Pts',(7.27603390513763,-105.443984254242,4.2008201337471));
#31334=CARTESIAN_POINT('Ctrl Pts',(9.70137854017372,-105.268984254242,-1.71237470597696E-11));
#31335=CARTESIAN_POINT('Ctrl Pts',(7.2760339051228,-105.093984254242,-4.20082013377278));
#31336=CARTESIAN_POINT('Ctrl Pts',(4.85068927007222,-104.918984254242,-8.40164026752808));
#31337=CARTESIAN_POINT('Ctrl Pts',(-1.47843125761923E-11,-104.743984254242,
-8.40164026751963));
#31338=CARTESIAN_POINT('Ctrl Pts',(-4.85068927010179,-104.568984254242,
-8.40164026751101));
#31339=CARTESIAN_POINT('Ctrl Pts',(-7.27603390513758,-104.393984254242,
-4.20082013374717));
#31340=CARTESIAN_POINT('Ctrl Pts',(-9.70137854017372,-104.218984254242,
1.70191603228232E-11));
#31341=CARTESIAN_POINT('Ctrl Pts',(-7.27603390512285,-104.043984254242,
4.20082013377271));
#31342=CARTESIAN_POINT('Ctrl Pts',(-4.85068927007183,-103.868984254242,
8.40164026752831));
#31343=CARTESIAN_POINT('Ctrl Pts',(1.46937378050979E-11,-103.693984254242,
8.40164026751963));
#31344=CARTESIAN_POINT('Ctrl Pts',(4.85068927010169,-103.518984254242,8.40164026751106));
#31345=CARTESIAN_POINT('Ctrl Pts',(7.27603390513778,-103.343984254242,4.20082013374684));
#31346=CARTESIAN_POINT('Ctrl Pts',(9.70137854017372,-103.168984254242,-1.69145735858769E-11));
#31347=CARTESIAN_POINT('Ctrl Pts',(7.27603390512289,-102.993984254242,-4.20082013377263));
#31348=CARTESIAN_POINT('Ctrl Pts',(4.85068927007192,-102.818984254242,-8.40164026752825));
#31349=CARTESIAN_POINT('Ctrl Pts',(-1.46031630340034E-11,-102.643984254242,
-8.40164026751963));
#31350=CARTESIAN_POINT('Ctrl Pts',(-4.8506892701016,-102.468984254242,-8.40164026751111));
#31351=CARTESIAN_POINT('Ctrl Pts',(-7.27603390513773,-102.293984254242,
-4.20082013374692));
#31352=CARTESIAN_POINT('Ctrl Pts',(-9.70137854017372,-102.118984254242,
1.73614463728169E-11));
#31353=CARTESIAN_POINT('Ctrl Pts',(-7.27603390512294,-101.943984254242,
4.20082013377255));
#31354=CARTESIAN_POINT('Ctrl Pts',(-4.85068927007201,-101.768984254242,
8.4016402675282));
#31355=CARTESIAN_POINT('Ctrl Pts',(1.49901662197534E-11,-101.593984254242,
8.40164026751963));
#31356=CARTESIAN_POINT('Ctrl Pts',(4.85068927010151,-101.418984254242,8.40164026751117));
#31357=CARTESIAN_POINT('Ctrl Pts',(7.27603390513769,-101.243984254242,4.200820133747));
#31358=CARTESIAN_POINT('Ctrl Pts',(9.70137854017372,-101.068984254242,-1.72568596358705E-11));
#31359=CARTESIAN_POINT('Ctrl Pts',(7.27603390512298,-100.893984254242,-4.20082013377247));
#31360=CARTESIAN_POINT('Ctrl Pts',(4.8506892700721,-100.718984254242,-8.40164026752815));
#31361=CARTESIAN_POINT('Ctrl Pts',(-1.48995914486589E-11,-100.543984254242,
-8.40164026751963));
#31362=CARTESIAN_POINT('Ctrl Pts',(-4.8506892701019,-100.368984254242,-8.40164026751094));
#31363=CARTESIAN_POINT('Ctrl Pts',(-7.27603390513764,-100.193984254242,
-4.20082013374707));
#31364=CARTESIAN_POINT('Ctrl Pts',(-9.70137854017372,-100.018984254242,
1.71522728989242E-11));
#31365=CARTESIAN_POINT('Ctrl Pts',(-7.27603390512279,-99.8439842542419,
4.2008201337728));
#31366=CARTESIAN_POINT('Ctrl Pts',(-4.85068927007219,-99.6689842542419,
8.4016402675281));
#31367=CARTESIAN_POINT('Ctrl Pts',(1.48090166775645E-11,-99.4939842542419,
8.40164026751963));
#31368=CARTESIAN_POINT('Ctrl Pts',(4.85068927010181,-99.3189842542419,8.401640267511));
#31369=CARTESIAN_POINT('Ctrl Pts',(7.2760339051376,-99.1439842542419,4.20082013374715));
#31370=CARTESIAN_POINT('Ctrl Pts',(9.70137854017372,-98.9689842542419,-1.70476861619779E-11));
#31371=CARTESIAN_POINT('Ctrl Pts',(7.27603390512283,-98.7939842542419,-4.20082013377273));
#31372=CARTESIAN_POINT('Ctrl Pts',(4.85068927007228,-98.6189842542419,-8.40164026752804));
#31373=CARTESIAN_POINT('Ctrl Pts',(-1.471844190647E-11,-98.4439842542419,
-8.40164026751963));
#31374=CARTESIAN_POINT('Ctrl Pts',(-4.85068927010172,-98.2689842542419,
-8.40164026751105));
#31375=CARTESIAN_POINT('Ctrl Pts',(-7.27603390513779,-98.0939842542419,
-4.20082013374682));
#31376=CARTESIAN_POINT('Ctrl Pts',(-9.70137854017372,-97.9189842542419,
1.69430994250315E-11));
#31377=CARTESIAN_POINT('Ctrl Pts',(-7.27603390512288,-97.7439842542419,
4.20082013377265));
#31378=CARTESIAN_POINT('Ctrl Pts',(-4.8506892700719,-97.5689842542419,8.40164026752827));
#31379=CARTESIAN_POINT('Ctrl Pts',(1.46278671353756E-11,-97.3939842542419,
8.40164026751963));
#31380=CARTESIAN_POINT('Ctrl Pts',(4.85068927010163,-97.2189842542419,8.4016402675111));
#31381=CARTESIAN_POINT('Ctrl Pts',(7.27603390513774,-97.0439842542419,4.2008201337469));
#31382=CARTESIAN_POINT('Ctrl Pts',(9.70137854017372,-96.8689842542419,-1.68385126880852E-11));
#31383=CARTESIAN_POINT('Ctrl Pts',(7.27603390512292,-96.6939842542419,-4.20082013377257));
#31384=CARTESIAN_POINT('Ctrl Pts',(4.85068927007199,-96.5189842542419,-8.40164026752822));
#31385=CARTESIAN_POINT('Ctrl Pts',(-1.50148703211256E-11,-96.3439842542419,
-8.40164026751963));
#31386=CARTESIAN_POINT('Ctrl Pts',(-4.85068927010154,-96.1689842542419,
-8.40164026751115));
#31387=CARTESIAN_POINT('Ctrl Pts',(-7.2760339051377,-95.9939842542419,-4.20082013374698));
#31388=CARTESIAN_POINT('Ctrl Pts',(-9.70137854017372,-95.8189842542419,
1.72853854750252E-11));
#31389=CARTESIAN_POINT('Ctrl Pts',(-7.27603390512297,-95.6439842542419,
4.20082013377249));
#31390=CARTESIAN_POINT('Ctrl Pts',(-4.85068927007208,-95.4689842542419,
8.40164026752816));
#31391=CARTESIAN_POINT('Ctrl Pts',(1.49242955500311E-11,-95.2939842542419,
8.40164026751963));
#31392=CARTESIAN_POINT('Ctrl Pts',(4.85068927010145,-95.1189842542419,8.40164026751121));
#31393=CARTESIAN_POINT('Ctrl Pts',(7.27603390513766,-94.9439842542419,4.20082013374705));
#31394=CARTESIAN_POINT('Ctrl Pts',(9.70137854017372,-94.7689842542419,-1.71807987380788E-11));
#31395=CARTESIAN_POINT('Ctrl Pts',(7.27603390512277,-94.5939842542419,-4.20082013377283));
#31396=CARTESIAN_POINT('Ctrl Pts',(4.85068927007217,-94.4189842542419,-8.40164026752811));
#31397=CARTESIAN_POINT('Ctrl Pts',(-1.48337207789367E-11,-94.2439842542419,
-8.40164026751963));
#31398=CARTESIAN_POINT('Ctrl Pts',(-4.85068927010184,-94.0689842542419,
-8.40164026751098));
#31399=CARTESIAN_POINT('Ctrl Pts',(-7.27603390513761,-93.8939842542419,
-4.20082013374713));
#31400=CARTESIAN_POINT('Ctrl Pts',(-9.70137854017372,-93.7189842542419,
1.70762120011325E-11));
#31401=CARTESIAN_POINT('Ctrl Pts',(-7.27603390512282,-93.5439842542419,
4.20082013377275));
#31402=CARTESIAN_POINT('Ctrl Pts',(-4.85068927007226,-93.3689842542419,
8.40164026752806));
#31403=CARTESIAN_POINT('Ctrl Pts',(1.47431460078422E-11,-93.1939842542419,
8.40164026751963));
#31404=CARTESIAN_POINT('Ctrl Pts',(4.85068927010175,-93.0189842542419,8.40164026751103));
#31405=CARTESIAN_POINT('Ctrl Pts',(7.2760339051378,-92.8439842542419,4.2008201337468));
#31406=CARTESIAN_POINT('Ctrl Pts',(9.70137854017372,-92.6689842542419,-1.69716252641861E-11));
#31407=CARTESIAN_POINT('Ctrl Pts',(7.27603390512287,-92.4939842542419,-4.20082013377267));
#31408=CARTESIAN_POINT('Ctrl Pts',(4.85068927007187,-92.3189842542419,-8.40164026752828));
#31409=CARTESIAN_POINT('Ctrl Pts',(-1.46525712367478E-11,-92.1439842542419,
-8.40164026751963));
#31410=CARTESIAN_POINT('Ctrl Pts',(-4.85068927010165,-91.9689842542419,
-8.40164026751109));
#31411=CARTESIAN_POINT('Ctrl Pts',(-7.27603390513776,-91.7939842542419,
-4.20082013374688));
#31412=CARTESIAN_POINT('Ctrl Pts',(-9.70137854017372,-91.6189842542419,
1.68670385272398E-11));
#31413=CARTESIAN_POINT('Ctrl Pts',(-7.27603390512291,-91.4439842542419,
4.20082013377259));
#31414=CARTESIAN_POINT('Ctrl Pts',(-4.85068927007196,-91.2689842542419,
8.40164026752823));
#31415=CARTESIAN_POINT('Ctrl Pts',(1.45619964656533E-11,-91.0939842542419,
8.40164026751963));
#31416=CARTESIAN_POINT('Ctrl Pts',(4.85068927010157,-90.9189842542419,8.40164026751114));
#31417=CARTESIAN_POINT('Ctrl Pts',(7.27603390513771,-90.7439842542419,4.20082013374695));
#31418=CARTESIAN_POINT('Ctrl Pts',(9.70137854017372,-90.5689842542419,-1.73139113141798E-11));
#31419=CARTESIAN_POINT('Ctrl Pts',(7.27603390512296,-90.3939842542419,-4.20082013377251));
#31420=CARTESIAN_POINT('Ctrl Pts',(4.85068927007205,-90.2189842542419,-8.40164026752818));
#31421=CARTESIAN_POINT('Ctrl Pts',(-1.49489996514033E-11,-90.0439842542419,
-8.40164026751963));
#31422=CARTESIAN_POINT('Ctrl Pts',(-4.85068927010147,-89.8689842542419,
-8.40164026751119));
#31423=CARTESIAN_POINT('Ctrl Pts',(-7.27603390513767,-89.6939842542419,
-4.20082013374703));
#31424=CARTESIAN_POINT('Ctrl Pts',(-9.70137854017372,-89.5189842542419,
1.72093245772335E-11));
#31425=CARTESIAN_POINT('Ctrl Pts',(-7.276033905123,-89.3439842542419,4.20082013377243));
#31426=CARTESIAN_POINT('Ctrl Pts',(-4.85068927007214,-89.1689842542419,
8.40164026752813));
#31427=CARTESIAN_POINT('Ctrl Pts',(1.48584248803088E-11,-88.9939842542419,
8.40164026751963));
#31428=CARTESIAN_POINT('Ctrl Pts',(4.85068927010186,-88.8189842542419,8.40164026751097));
#31429=CARTESIAN_POINT('Ctrl Pts',(7.27603390513762,-88.6439842542419,4.20082013374711));
#31430=CARTESIAN_POINT('Ctrl Pts',(9.70137854017372,-88.4689842542419,-1.71047378402871E-11));
#31431=CARTESIAN_POINT('Ctrl Pts',(7.27603390512281,-88.2939842542419,-4.20082013377277));
#31432=CARTESIAN_POINT('Ctrl Pts',(4.85068927007223,-88.1189842542419,-8.40164026752807));
#31433=CARTESIAN_POINT('Ctrl Pts',(-1.47678501092144E-11,-87.9439842542419,
-8.40164026751963));
#31434=CARTESIAN_POINT('Ctrl Pts',(-4.85068927010177,-87.7689842542419,
-8.40164026751102));
#31435=CARTESIAN_POINT('Ctrl Pts',(-7.27603390513758,-87.5939842542419,
-4.20082013374719));
#31436=CARTESIAN_POINT('Ctrl Pts',(-9.70137854017372,-87.4189842542419,
1.70001511033408E-11));
#31437=CARTESIAN_POINT('Ctrl Pts',(-7.27603390512285,-87.2439842542419,
4.20082013377269));
#31438=CARTESIAN_POINT('Ctrl Pts',(-4.85068927007185,-87.0689842542419,
8.4016402675283));
#31439=CARTESIAN_POINT('Ctrl Pts',(1.46772753381199E-11,-86.8939842542419,
8.40164026751963));
#31440=CARTESIAN_POINT('Ctrl Pts',(4.85068927010168,-86.7189842542419,8.40164026751107));
#31441=CARTESIAN_POINT('Ctrl Pts',(7.27603390513777,-86.5439842542419,4.20082013374685));
#31442=CARTESIAN_POINT('Ctrl Pts',(9.70137854017372,-86.3689842542419,-1.68955643663944E-11));
#31443=CARTESIAN_POINT('Ctrl Pts',(7.2760339051229,-86.1939842542419,-4.20082013377261));
#31444=CARTESIAN_POINT('Ctrl Pts',(4.85068927007194,-86.0189842542419,-8.40164026752825));
#31445=CARTESIAN_POINT('Ctrl Pts',(-1.45867005670255E-11,-85.8439842542419,
-8.40164026751963));
#31446=CARTESIAN_POINT('Ctrl Pts',(-4.85068927010159,-85.6689842542419,
-8.40164026751112));
#31447=CARTESIAN_POINT('Ctrl Pts',(-7.27603390513773,-85.4939842542419,
-4.20082013374693));
#31448=CARTESIAN_POINT('Ctrl Pts',(-9.70137854017372,-85.3189842542419,
1.67909776294481E-11));
#31449=CARTESIAN_POINT('Ctrl Pts',(-7.27603390512294,-85.143984254242,4.20082013377253));
#31450=CARTESIAN_POINT('Ctrl Pts',(-4.85068927007203,-84.9689842542419,
8.40164026752819));
#31451=CARTESIAN_POINT('Ctrl Pts',(1.49737037527755E-11,-84.7939842542419,
8.40164026751963));
#31452=CARTESIAN_POINT('Ctrl Pts',(4.8506892701015,-84.6189842542419,8.40164026751117));
#31453=CARTESIAN_POINT('Ctrl Pts',(7.27603390513768,-84.443984254242,4.20082013374701));
#31454=CARTESIAN_POINT('Ctrl Pts',(9.70137854017372,-84.2689842542419,-1.72378504163881E-11));
#31455=CARTESIAN_POINT('Ctrl Pts',(7.27603390512299,-84.0939842542419,-4.20082013377245));
#31456=CARTESIAN_POINT('Ctrl Pts',(4.85068927007212,-83.9189842542419,-8.40164026752814));
#31457=CARTESIAN_POINT('Ctrl Pts',(-1.4883128981681E-11,-83.7439842542419,
-8.40164026751963));
#31458=CARTESIAN_POINT('Ctrl Pts',(-4.85068927010141,-83.5689842542419,
-8.40164026751123));
#31459=CARTESIAN_POINT('Ctrl Pts',(-7.27603390513763,-83.3939842542419,
-4.20082013374709));
#31460=CARTESIAN_POINT('Ctrl Pts',(-9.70137854017372,-83.2189842542419,
1.71332636794417E-11));
#31461=CARTESIAN_POINT('Ctrl Pts',(-7.2760339051228,-83.0439842542419,4.20082013377279));
#31462=CARTESIAN_POINT('Ctrl Pts',(-4.85068927007221,-82.868984254242,8.40164026752809));
#31463=CARTESIAN_POINT('Ctrl Pts',(1.47925542105866E-11,-82.6939842542419,
8.40164026751963));
#31464=CARTESIAN_POINT('Ctrl Pts',(4.85068927010179,-82.5189842542419,8.401640267511));
#31465=CARTESIAN_POINT('Ctrl Pts',(7.27603390513759,-82.3439842542419,4.20082013374717));
#31466=CARTESIAN_POINT('Ctrl Pts',(9.70137854017372,-82.1689842542419,-1.70286769424954E-11));
#31467=CARTESIAN_POINT('Ctrl Pts',(7.27603390512284,-81.993984254242,-4.20082013377271));
#31468=CARTESIAN_POINT('Ctrl Pts',(4.8506892700723,-81.8189842542419,-8.40164026752804));
#31469=CARTESIAN_POINT('Ctrl Pts',(-1.47019794394921E-11,-81.6439842542419,
-8.40164026751963));
#31470=CARTESIAN_POINT('Ctrl Pts',(-4.8506892701017,-81.4689842542419,-8.40164026751106));
#31471=CARTESIAN_POINT('Ctrl Pts',(-7.27603390513778,-81.293984254242,-4.20082013374683));
#31472=CARTESIAN_POINT('Ctrl Pts',(-9.70137854017372,-81.1189842542419,
1.69240902055491E-11));
#31473=CARTESIAN_POINT('Ctrl Pts',(-7.27603390512289,-80.9439842542419,
4.20082013377263));
#31474=CARTESIAN_POINT('Ctrl Pts',(-4.85068927007191,-80.768984254242,8.40164026752826));
#31475=CARTESIAN_POINT('Ctrl Pts',(1.46114046683977E-11,-80.5939842542419,
8.40164026751963));
#31476=CARTESIAN_POINT('Ctrl Pts',(4.85068927010161,-80.4189842542419,8.40164026751111));
#31477=CARTESIAN_POINT('Ctrl Pts',(7.27603390513774,-80.243984254242,4.20082013374691));
#31478=CARTESIAN_POINT('Ctrl Pts',(9.70137854017372,-80.068984254242,-1.68195034686027E-11));
#31479=CARTESIAN_POINT('Ctrl Pts',(7.27603390512293,-79.8939842542419,-4.20082013377256));
#31480=CARTESIAN_POINT('Ctrl Pts',(4.850689270072,-79.718984254242,-8.40164026752821));
#31481=CARTESIAN_POINT('Ctrl Pts',(-1.49984078541476E-11,-79.5439842542419,
-8.40164026751963));
#31482=CARTESIAN_POINT('Ctrl Pts',(-4.85068927010152,-79.3689842542419,
-8.40164026751116));
#31483=CARTESIAN_POINT('Ctrl Pts',(-7.27603390513769,-79.193984254242,-4.20082013374699));
#31484=CARTESIAN_POINT('Ctrl Pts',(-9.70137854017372,-79.0189842542419,
1.72663762555427E-11));
#31485=CARTESIAN_POINT('Ctrl Pts',(-7.27603390512298,-78.8439842542419,
4.20082013377248));
#31486=CARTESIAN_POINT('Ctrl Pts',(-4.85068927007209,-78.668984254242,8.40164026752815));
#31487=CARTESIAN_POINT('Ctrl Pts',(1.49078330830532E-11,-78.493984254242,
8.40164026751963));
#31488=CARTESIAN_POINT('Ctrl Pts',(4.85068927010143,-78.3189842542419,8.40164026751122));
#31489=CARTESIAN_POINT('Ctrl Pts',(7.27603390513765,-78.143984254242,4.20082013374707));
#31490=CARTESIAN_POINT('Ctrl Pts',(9.70137854017372,-77.9689842542419,-1.71617895185964E-11));
#31491=CARTESIAN_POINT('Ctrl Pts',(7.27603390512302,-77.7939842542419,-4.2008201337724));
#31492=CARTESIAN_POINT('Ctrl Pts',(4.85068927007219,-77.618984254242,-8.4016402675281));
#31493=CARTESIAN_POINT('Ctrl Pts',(-1.48172583119587E-11,-77.443984254242,
-8.40164026751963));
#31494=CARTESIAN_POINT('Ctrl Pts',(-4.85068927010182,-77.268984254242,-8.40164026751099));
#31495=CARTESIAN_POINT('Ctrl Pts',(-7.2760339051376,-77.0939842542419,-4.20082013374715));
#31496=CARTESIAN_POINT('Ctrl Pts',(-9.70137854017372,-76.918984254242,1.705720278165E-11));
#31497=CARTESIAN_POINT('Ctrl Pts',(-7.27603390512283,-76.743984254242,4.20082013377273));
#31498=CARTESIAN_POINT('Ctrl Pts',(-4.85068927007227,-76.5689842542419,
8.40164026752805));
#31499=CARTESIAN_POINT('Ctrl Pts',(1.47266835408643E-11,-76.393984254242,
8.40164026751963));
#31500=CARTESIAN_POINT('Ctrl Pts',(4.85068927010173,-76.2189842542419,8.40164026751104));
#31501=CARTESIAN_POINT('Ctrl Pts',(7.27603390513756,-76.0439842542419,4.20082013374722));
#31502=CARTESIAN_POINT('Ctrl Pts',(9.70137854017372,-75.868984254242,-1.69526160447037E-11));
#31503=CARTESIAN_POINT('Ctrl Pts',(7.27603390512287,-75.693984254242,-4.20082013377265));
#31504=CARTESIAN_POINT('Ctrl Pts',(4.85068927007189,-75.518984254242,-8.40164026752827));
#31505=CARTESIAN_POINT('Ctrl Pts',(-1.46361087697698E-11,-75.343984254242,
-8.40164026751963));
#31506=CARTESIAN_POINT('Ctrl Pts',(-4.85068927010164,-75.1689842542419,
-8.40164026751109));
#31507=CARTESIAN_POINT('Ctrl Pts',(-7.27603390513775,-74.993984254242,-4.20082013374689));
#31508=CARTESIAN_POINT('Ctrl Pts',(-9.70137854017372,-74.818984254242,1.68480293077573E-11));
#31509=CARTESIAN_POINT('Ctrl Pts',(-7.27603390512292,-74.643984254242,4.20082013377258));
#31510=CARTESIAN_POINT('Ctrl Pts',(-4.85068927007198,-74.4689842542419,
8.40164026752822));
#31511=CARTESIAN_POINT('Ctrl Pts',(1.45455339986754E-11,-74.293984254242,
8.40164026751963));
#31512=CARTESIAN_POINT('Ctrl Pts',(4.85068927010155,-74.118984254242,8.40164026751115));
#31513=CARTESIAN_POINT('Ctrl Pts',(7.2760339051377,-73.943984254242,4.20082013374697));
#31514=CARTESIAN_POINT('Ctrl Pts',(9.70137854017372,-73.768984254242,-1.72949020946973E-11));
#31515=CARTESIAN_POINT('Ctrl Pts',(7.27603390512296,-73.593984254242,-4.2008201337725));
#31516=CARTESIAN_POINT('Ctrl Pts',(4.85068927007207,-73.4189842542419,-8.40164026752817));
#31517=CARTESIAN_POINT('Ctrl Pts',(-1.49325371844254E-11,-73.243984254242,
-8.40164026751963));
#31518=CARTESIAN_POINT('Ctrl Pts',(-4.85068927010146,-73.068984254242,-8.4016402675112));
#31519=CARTESIAN_POINT('Ctrl Pts',(-7.27603390513766,-72.893984254242,-4.20082013374705));
#31520=CARTESIAN_POINT('Ctrl Pts',(-9.70137854017372,-72.718984254242,1.7190315357751E-11));
#31521=CARTESIAN_POINT('Ctrl Pts',(-7.27603390512301,-72.543984254242,4.20082013377242));
#31522=CARTESIAN_POINT('Ctrl Pts',(-4.85068927007216,-72.368984254242,8.40164026752812));
#31523=CARTESIAN_POINT('Ctrl Pts',(1.48419624133309E-11,-72.193984254242,
8.40164026751963));
#31524=CARTESIAN_POINT('Ctrl Pts',(4.85068927010137,-72.018984254242,8.40164026751125));
#31525=CARTESIAN_POINT('Ctrl Pts',(7.27603390513761,-71.843984254242,4.20082013374713));
#31526=CARTESIAN_POINT('Ctrl Pts',(9.70137854017372,-71.6689842542419,-1.70857286208046E-11));
#31527=CARTESIAN_POINT('Ctrl Pts',(7.27603390512282,-71.493984254242,-4.20082013377275));
#31528=CARTESIAN_POINT('Ctrl Pts',(4.85068927007225,-71.318984254242,-8.40164026752806));
#31529=CARTESIAN_POINT('Ctrl Pts',(-1.47513876422365E-11,-71.143984254242,
-8.40164026751963));
#31530=CARTESIAN_POINT('Ctrl Pts',(-4.85068927010175,-70.968984254242,-8.40164026751103));
#31531=CARTESIAN_POINT('Ctrl Pts',(-7.27603390513757,-70.793984254242,-4.2008201337472));
#31532=CARTESIAN_POINT('Ctrl Pts',(-9.70137854017372,-70.618984254242,1.69811418838583E-11));
#31533=CARTESIAN_POINT('Ctrl Pts',(-7.27603390512286,-70.443984254242,4.20082013377267));
#31534=CARTESIAN_POINT('Ctrl Pts',(-4.85068927007234,-70.268984254242,8.40164026752801));
#31535=CARTESIAN_POINT('Ctrl Pts',(1.4660812871142E-11,-70.093984254242,
8.40164026751963));
#31536=CARTESIAN_POINT('Ctrl Pts',(4.85068927010166,-69.918984254242,8.40164026751108));
#31537=CARTESIAN_POINT('Ctrl Pts',(7.27603390513776,-69.743984254242,4.20082013374687));
#31538=CARTESIAN_POINT('Ctrl Pts',(9.70137854017372,-69.568984254242,-1.6876555146912E-11));
#31539=CARTESIAN_POINT('Ctrl Pts',(7.27603390512291,-69.393984254242,-4.2008201337726));
#31540=CARTESIAN_POINT('Ctrl Pts',(4.85068927007195,-69.218984254242,-8.40164026752823));
#31541=CARTESIAN_POINT('Ctrl Pts',(-1.45702381000475E-11,-69.043984254242,
-8.40164026751963));
#31542=CARTESIAN_POINT('Ctrl Pts',(-4.85068927010157,-68.868984254242,-8.40164026751113));
#31543=CARTESIAN_POINT('Ctrl Pts',(-7.27603390513772,-68.693984254242,-4.20082013374695));
#31544=CARTESIAN_POINT('Ctrl Pts',(-9.70137854017372,-68.518984254242,1.67719684099656E-11));
#31545=CARTESIAN_POINT('Ctrl Pts',(-7.27603390512295,-68.343984254242,4.20082013377252));
#31546=CARTESIAN_POINT('Ctrl Pts',(-4.85068927007204,-68.168984254242,8.40164026752818));
#31547=CARTESIAN_POINT('Ctrl Pts',(1.49572412857975E-11,-67.993984254242,
8.40164026751963));
#31548=CARTESIAN_POINT('Ctrl Pts',(4.85068927010148,-67.818984254242,8.40164026751119));
#31549=CARTESIAN_POINT('Ctrl Pts',(7.27603390513767,-67.643984254242,4.20082013374703));
#31550=CARTESIAN_POINT('Ctrl Pts',(9.70137854017372,-67.468984254242,-1.72188411969056E-11));
#31551=CARTESIAN_POINT('Ctrl Pts',(7.276033905123,-67.293984254242,-4.20082013377244));
#31552=CARTESIAN_POINT('Ctrl Pts',(4.85068927007213,-67.118984254242,-8.40164026752813));
#31553=CARTESIAN_POINT('Ctrl Pts',(-1.48666665147031E-11,-66.943984254242,
-8.40164026751963));
#31554=CARTESIAN_POINT('Ctrl Pts',(-4.85068927010139,-66.768984254242,-8.40164026751124));
#31555=CARTESIAN_POINT('Ctrl Pts',(-7.27603390513763,-66.593984254242,-4.2008201337471));
#31556=CARTESIAN_POINT('Ctrl Pts',(-9.70137854017372,-66.418984254242,1.71142544599593E-11));
#31557=CARTESIAN_POINT('Ctrl Pts',(-7.27603390512304,-66.243984254242,4.20082013377236));
#31558=CARTESIAN_POINT('Ctrl Pts',(-4.85068927007222,-66.068984254242,8.40164026752808));
#31559=CARTESIAN_POINT('Ctrl Pts',(1.47760917436086E-11,-65.893984254242,
8.40164026751963));
#31560=CARTESIAN_POINT('Ctrl Pts',(4.85068927010178,-65.718984254242,8.40164026751101));
#31561=CARTESIAN_POINT('Ctrl Pts',(7.27603390513758,-65.543984254242,4.20082013374718));
#31562=CARTESIAN_POINT('Ctrl Pts',(9.70137854017372,-65.368984254242,-1.70096677230129E-11));
#31563=CARTESIAN_POINT('Ctrl Pts',(7.27603390512285,-65.193984254242,-4.2008201337727));
#31564=CARTESIAN_POINT('Ctrl Pts',(4.85068927007232,-65.018984254242,-8.40164026752803));
#31565=CARTESIAN_POINT('Ctrl Pts',(-1.46855169725142E-11,-64.843984254242,
-8.40164026751963));
#31566=CARTESIAN_POINT('Ctrl Pts',(-4.85068927010169,-64.668984254242,-8.40164026751107));
#31567=CARTESIAN_POINT('Ctrl Pts',(-7.27603390513754,-64.493984254242,-4.20082013374726));
#31568=CARTESIAN_POINT('Ctrl Pts',(-9.70137854017372,-64.318984254242,1.69050809860666E-11));
#31569=CARTESIAN_POINT('Ctrl Pts',(-7.27603390512289,-64.143984254242,4.20082013377262));
#31570=CARTESIAN_POINT('Ctrl Pts',(-4.85068927007193,-63.968984254242,8.40164026752825));
#31571=CARTESIAN_POINT('Ctrl Pts',(1.45949422014197E-11,-63.793984254242,
8.40164026751963));
#31572=CARTESIAN_POINT('Ctrl Pts',(4.8506892701016,-63.618984254242,8.40164026751112));
#31573=CARTESIAN_POINT('Ctrl Pts',(7.27603390513773,-63.443984254242,4.20082013374692));
#31574=CARTESIAN_POINT('Ctrl Pts',(9.70137854017372,-63.268984254242,-1.68004942491202E-11));
#31575=CARTESIAN_POINT('Ctrl Pts',(7.27603390512294,-63.093984254242,-4.20082013377254));
#31576=CARTESIAN_POINT('Ctrl Pts',(4.85068927007202,-62.918984254242,-8.4016402675282));
#31577=CARTESIAN_POINT('Ctrl Pts',(-1.45043674303253E-11,-62.743984254242,
-8.40164026751963));
#31578=CARTESIAN_POINT('Ctrl Pts',(-4.85068927010151,-62.568984254242,-8.40164026751117));
#31579=CARTESIAN_POINT('Ctrl Pts',(-7.27603390513768,-62.393984254242,-4.200820133747));
#31580=CARTESIAN_POINT('Ctrl Pts',(-9.70137854017372,-62.218984254242,1.72473670360602E-11));
#31581=CARTESIAN_POINT('Ctrl Pts',(-7.27603390512298,-62.043984254242,4.20082013377246));
#31582=CARTESIAN_POINT('Ctrl Pts',(-4.85068927007211,-61.868984254242,8.40164026752814));
#31583=CARTESIAN_POINT('Ctrl Pts',(1.48913706160753E-11,-61.693984254242,
8.40164026751963));
#31584=CARTESIAN_POINT('Ctrl Pts',(4.85068927010141,-61.518984254242,8.40164026751122));
#31585=CARTESIAN_POINT('Ctrl Pts',(7.27603390513764,-61.343984254242,4.20082013374708));
#31586=CARTESIAN_POINT('Ctrl Pts',(9.70137854017372,-61.168984254242,-1.71427802991139E-11));
#31587=CARTESIAN_POINT('Ctrl Pts',(7.27603390512303,-60.993984254242,-4.20082013377238));
#31588=CARTESIAN_POINT('Ctrl Pts',(4.8506892700722,-60.818984254242,-8.40164026752809));
#31589=CARTESIAN_POINT('Ctrl Pts',(-1.48007958449808E-11,-60.643984254242,
-8.40164026751963));
#31590=CARTESIAN_POINT('Ctrl Pts',(-4.8506892701018,-60.468984254242,-8.401640267511));
#31591=CARTESIAN_POINT('Ctrl Pts',(-7.27603390513759,-60.293984254242,-4.20082013374716));
#31592=CARTESIAN_POINT('Ctrl Pts',(-9.70137854017372,-60.118984254242,1.70381935621676E-11));
#31593=CARTESIAN_POINT('Ctrl Pts',(-7.27603390512284,-59.943984254242,4.20082013377272));
#31594=CARTESIAN_POINT('Ctrl Pts',(-4.85068927007229,-59.768984254242,8.40164026752804));
#31595=CARTESIAN_POINT('Ctrl Pts',(1.47102210738864E-11,-59.593984254242,
8.40164026751963));
#31596=CARTESIAN_POINT('Ctrl Pts',(4.85068927010171,-59.418984254242,8.40164026751105));
#31597=CARTESIAN_POINT('Ctrl Pts',(7.27603390513755,-59.243984254242,4.20082013374724));
#31598=CARTESIAN_POINT('Ctrl Pts',(9.70137854017372,-59.068984254242,-1.69336068252212E-11));
#31599=CARTESIAN_POINT('Ctrl Pts',(7.27603390512288,-58.893984254242,-4.20082013377264));
#31600=CARTESIAN_POINT('Ctrl Pts',(4.85068927007238,-58.718984254242,-8.40164026752799));
#31601=CARTESIAN_POINT('Ctrl Pts',(-1.46196463027919E-11,-58.543984254242,
-8.40164026751963));
#31602=CARTESIAN_POINT('Ctrl Pts',(-4.85068927010162,-58.368984254242,-8.40164026751111));
#31603=CARTESIAN_POINT('Ctrl Pts',(-7.27603390513774,-58.193984254242,-4.2008201337469));
#31604=CARTESIAN_POINT('Ctrl Pts',(-9.70137854017372,-58.018984254242,1.68290200882749E-11));
#31605=CARTESIAN_POINT('Ctrl Pts',(-7.27603390512293,-57.843984254242,4.20082013377256));
#31606=CARTESIAN_POINT('Ctrl Pts',(-4.85068927007199,-57.668984254242,8.40164026752821));
#31607=CARTESIAN_POINT('Ctrl Pts',(1.45290715316974E-11,-57.493984254242,
8.40164026751963));
#31608=CARTESIAN_POINT('Ctrl Pts',(4.85068927010153,-57.318984254242,8.40164026751116));
#31609=CARTESIAN_POINT('Ctrl Pts',(7.2760339051377,-57.143984254242,4.20082013374698));
#31610=CARTESIAN_POINT('Ctrl Pts',(9.70137854017372,-56.968984254242,-1.67244333513285E-11));
#31611=CARTESIAN_POINT('Ctrl Pts',(7.27603390512297,-56.793984254242,-4.20082013377248));
#31612=CARTESIAN_POINT('Ctrl Pts',(4.85068927007208,-56.618984254242,-8.40164026752816));
#31613=CARTESIAN_POINT('Ctrl Pts',(-1.49160747174474E-11,-56.443984254242,
-8.40164026751963));
#31614=CARTESIAN_POINT('Ctrl Pts',(-4.85068927010144,-56.268984254242,-8.40164026751121));
#31615=CARTESIAN_POINT('Ctrl Pts',(-7.27603390513765,-56.093984254242,-4.20082013374706));
#31616=CARTESIAN_POINT('Ctrl Pts',(-9.70137854017372,-55.918984254242,1.71713061382685E-11));
#31617=CARTESIAN_POINT('Ctrl Pts',(-7.27603390512302,-55.743984254242,4.2008201337724));
#31618=CARTESIAN_POINT('Ctrl Pts',(-4.85068927007218,-55.568984254242,8.40164026752811));
#31619=CARTESIAN_POINT('Ctrl Pts',(1.4825499946353E-11,-55.393984254242,
8.40164026751963));
#31620=CARTESIAN_POINT('Ctrl Pts',(4.85068927010135,-55.218984254242,8.40164026751126));
#31621=CARTESIAN_POINT('Ctrl Pts',(7.27603390513761,-55.043984254242,4.20082013374714));
#31622=CARTESIAN_POINT('Ctrl Pts',(9.70137854017372,-54.868984254242,-1.70667194013222E-11));
#31623=CARTESIAN_POINT('Ctrl Pts',(7.27603390512282,-54.693984254242,-4.20082013377274));
#31624=CARTESIAN_POINT('Ctrl Pts',(4.85068927007227,-54.518984254242,-8.40164026752806));
#31625=CARTESIAN_POINT('Ctrl Pts',(-1.47349251752585E-11,-54.343984254242,
-8.40164026751963));
#31626=CARTESIAN_POINT('Ctrl Pts',(-4.85068927010174,-54.168984254242,-8.40164026751104));
#31627=CARTESIAN_POINT('Ctrl Pts',(-7.27603390513756,-53.993984254242,-4.20082013374722));
#31628=CARTESIAN_POINT('Ctrl Pts',(-9.70137854017372,-53.818984254242,1.69621326643758E-11));
#31629=CARTESIAN_POINT('Ctrl Pts',(-7.27603390512287,-53.643984254242,4.20082013377266));
#31630=CARTESIAN_POINT('Ctrl Pts',(-4.85068927007236,-53.468984254242,8.401640267528));
#31631=CARTESIAN_POINT('Ctrl Pts',(1.46443504041641E-11,-53.293984254242,
8.40164026751963));
#31632=CARTESIAN_POINT('Ctrl Pts',(4.85068927010165,-53.118984254242,8.40164026751109));
#31633=CARTESIAN_POINT('Ctrl Pts',(7.27603390513752,-52.943984254242,4.2008201337473));
#31634=CARTESIAN_POINT('Ctrl Pts',(9.70137854017372,-52.768984254242,-1.68575459274295E-11));
#31635=CARTESIAN_POINT('Ctrl Pts',(7.27603390512292,-52.593984254242,-4.20082013377258));
#31636=CARTESIAN_POINT('Ctrl Pts',(4.85068927007197,-52.418984254242,-8.40164026752823));
#31637=CARTESIAN_POINT('Ctrl Pts',(-1.45537756330696E-11,-52.243984254242,
-8.40164026751963));
#31638=CARTESIAN_POINT('Ctrl Pts',(-4.85068927010155,-52.068984254242,-8.40164026751114));
#31639=CARTESIAN_POINT('Ctrl Pts',(-7.27603390513771,-51.893984254242,-4.20082013374696));
#31640=CARTESIAN_POINT('Ctrl Pts',(-9.70137854017372,-51.718984254242,1.67529591904832E-11));
#31641=CARTESIAN_POINT('Ctrl Pts',(-7.27603390512296,-51.543984254242,4.2008201337725));
#31642=CARTESIAN_POINT('Ctrl Pts',(-4.85068927007206,-51.368984254242,8.40164026752817));
#31643=CARTESIAN_POINT('Ctrl Pts',(1.44632008619752E-11,-51.193984254242,
8.40164026751963));
#31644=CARTESIAN_POINT('Ctrl Pts',(4.85068927010146,-51.018984254242,8.4016402675112));
#31645=CARTESIAN_POINT('Ctrl Pts',(7.27603390513766,-50.843984254242,4.20082013374704));
#31646=CARTESIAN_POINT('Ctrl Pts',(9.70137854017372,-50.668984254242,-1.71998319774232E-11));
#31647=CARTESIAN_POINT('Ctrl Pts',(7.27603390512301,-50.493984254242,-4.20082013377243));
#31648=CARTESIAN_POINT('Ctrl Pts',(4.85068927007215,-50.318984254242,-8.40164026752812));
#31649=CARTESIAN_POINT('Ctrl Pts',(-1.48502040477252E-11,-50.143984254242,
-8.40164026751963));
#31650=CARTESIAN_POINT('Ctrl Pts',(-4.85068927010137,-49.968984254242,-8.40164026751125));
#31651=CARTESIAN_POINT('Ctrl Pts',(-7.27603390513762,-49.793984254242,-4.20082013374712));
#31652=CARTESIAN_POINT('Ctrl Pts',(-9.70137854017372,-49.618984254242,1.70952452404768E-11));
#31653=CARTESIAN_POINT('Ctrl Pts',(-7.27603390512305,-49.443984254242,4.20082013377235));
#31654=CARTESIAN_POINT('Ctrl Pts',(-4.85068927007224,-49.268984254242,8.40164026752807));
#31655=CARTESIAN_POINT('Ctrl Pts',(1.47596292766307E-11,-49.093984254242,
8.40164026751963));
#31656=CARTESIAN_POINT('Ctrl Pts',(4.85068927010176,-48.918984254242,8.40164026751102));
#31657=CARTESIAN_POINT('Ctrl Pts',(7.27603390513757,-48.743984254242,4.2008201337472));
#31658=CARTESIAN_POINT('Ctrl Pts',(9.70137854017372,-48.568984254242,-1.69906585035305E-11));
#31659=CARTESIAN_POINT('Ctrl Pts',(7.27603390512286,-48.393984254242,-4.20082013377268));
#31660=CARTESIAN_POINT('Ctrl Pts',(4.85068927007233,-48.218984254242,-8.40164026752802));
#31661=CARTESIAN_POINT('Ctrl Pts',(-1.46690545055362E-11,-48.043984254242,
-8.40164026751963));
#31662=CARTESIAN_POINT('Ctrl Pts',(-4.85068927010167,-47.868984254242,-8.40164026751108));
#31663=CARTESIAN_POINT('Ctrl Pts',(-7.27603390513753,-47.693984254242,-4.20082013374728));
#31664=CARTESIAN_POINT('Ctrl Pts',(-7.69929559114725,-47.6634439368035,
-3.46770938867822));
#31665=CARTESIAN_POINT('Ctrl Pts',(-7.96780251527898,-47.63,-2.66489817109789));
#31666=CARTESIAN_POINT('',(-0.219644606349537,-212.63,-9.92210040505713));
#31667=CARTESIAN_POINT('Ctrl Pts',(5.91264939824166,-212.63,5.96893091585755));
#31668=CARTESIAN_POINT('Ctrl Pts',(6.45001176255729,-212.63,5.51316655921169));
#31669=CARTESIAN_POINT('Ctrl Pts',(6.92646504757685,-212.63,4.99014851913996));
#31670=CARTESIAN_POINT('Ctrl Pts',(7.64146177750064,-212.63,3.96829926249844));
#31671=CARTESIAN_POINT('Ctrl Pts',(8.02934603926417,-212.63,3.32494664782914));
#31672=CARTESIAN_POINT('Ctrl Pts',(8.75489545839817,-212.63,1.42020078435432));
#31673=CARTESIAN_POINT('Ctrl Pts',(8.95163602245128,-212.63,0.279729502662558));
#31674=CARTESIAN_POINT('Ctrl Pts',(8.90204310970132,-212.63,-1.94200526332423));
#31675=CARTESIAN_POINT('Ctrl Pts',(8.6828950463362,-212.63,-3.00390386902858));
#31676=CARTESIAN_POINT('Ctrl Pts',(7.851506811291,-212.63,-5.05909339484079));
#31677=CARTESIAN_POINT('Ctrl Pts',(7.21763657197169,-212.63,-6.04291134052863));
#31678=CARTESIAN_POINT('Ctrl Pts',(5.59478772607511,-212.63,-7.78711679211931));
#31679=CARTESIAN_POINT('Ctrl Pts',(4.5846114302215,-212.63,-8.52028630432628));
#31680=CARTESIAN_POINT('Ctrl Pts',(2.63065283482949,-212.63,-9.42649812028965));
#31681=CARTESIAN_POINT('Ctrl Pts',(1.41906832976769,-212.63,-9.86110934044648));
#31682=CARTESIAN_POINT('Ctrl Pts',(-0.219644606349541,-212.63,-9.9221004050572));
#31683=CARTESIAN_POINT('Ctrl Pts',(-0.219644606349537,-212.63,-9.92210040505713));
#31684=CARTESIAN_POINT('Ctrl Pts',(-5.80268971544237,-212.457306795807,
-9.79850905895531));
#31685=CARTESIAN_POINT('Ctrl Pts',(-8.59489616871563,-212.28675111262,-4.96226561664434));
#31686=CARTESIAN_POINT('Ctrl Pts',(-11.4598615582757,-212.11175111262,2.05132644302783E-11));
#31687=CARTESIAN_POINT('Ctrl Pts',(-8.59489616869786,-211.93675111262,4.96226561667511));
#31688=CARTESIAN_POINT('Ctrl Pts',(-5.72993077912007,-211.76175111262,9.9245312333297));
#31689=CARTESIAN_POINT('Ctrl Pts',(1.77644004088984E-11,-211.58675111262,
9.92453123331945));
#31690=CARTESIAN_POINT('Ctrl Pts',(5.72993077915559,-211.41175111262,9.92453123330919));
#31691=CARTESIAN_POINT('Ctrl Pts',(8.59489616871563,-211.23675111262,4.96226561664434));
#31692=CARTESIAN_POINT('Ctrl Pts',(11.4598615582757,-211.06175111262,-2.05118610020007E-11));
#31693=CARTESIAN_POINT('Ctrl Pts',(8.59489616869787,-210.88675111262,-4.9622656166751));
#31694=CARTESIAN_POINT('Ctrl Pts',(5.72993077912007,-210.71175111262,-9.9245312333297));
#31695=CARTESIAN_POINT('Ctrl Pts',(-1.77631850043576E-11,-210.53675111262,
-9.92453123331945));
#31696=CARTESIAN_POINT('Ctrl Pts',(-5.72993077915559,-210.36175111262,-9.9245312333092));
#31697=CARTESIAN_POINT('Ctrl Pts',(-8.59489616871563,-210.18675111262,-4.96226561664434));
#31698=CARTESIAN_POINT('Ctrl Pts',(-11.4598615582757,-210.01175111262,2.05002791719943E-11));
#31699=CARTESIAN_POINT('Ctrl Pts',(-8.59489616869787,-209.83675111262,4.9622656166751));
#31700=CARTESIAN_POINT('Ctrl Pts',(-5.72993077912008,-209.66175111262,9.9245312333297));
#31701=CARTESIAN_POINT('Ctrl Pts',(1.77619695998168E-11,-209.48675111262,
9.92453123331945));
#31702=CARTESIAN_POINT('Ctrl Pts',(5.72993077915559,-209.31175111262,9.9245312333092));
#31703=CARTESIAN_POINT('Ctrl Pts',(8.59489616871562,-209.13675111262,4.96226561664435));
#31704=CARTESIAN_POINT('Ctrl Pts',(11.4598615582757,-208.96175111262,-2.05090541454455E-11));
#31705=CARTESIAN_POINT('Ctrl Pts',(8.59489616869787,-208.78675111262,-4.9622656166751));
#31706=CARTESIAN_POINT('Ctrl Pts',(5.72993077912008,-208.61175111262,-9.9245312333297));
#31707=CARTESIAN_POINT('Ctrl Pts',(-1.7760754195276E-11,-208.43675111262,
-9.92453123331945));
#31708=CARTESIAN_POINT('Ctrl Pts',(-5.72993077915559,-208.26175111262,-9.9245312333092));
#31709=CARTESIAN_POINT('Ctrl Pts',(-8.59489616871562,-208.08675111262,-4.96226561664435));
#31710=CARTESIAN_POINT('Ctrl Pts',(-11.4598615582757,-207.91175111262,2.04872939137103E-11));
#31711=CARTESIAN_POINT('Ctrl Pts',(-8.59489616869787,-207.73675111262,4.9622656166751));
#31712=CARTESIAN_POINT('Ctrl Pts',(-5.72993077912008,-207.56175111262,9.9245312333297));
#31713=CARTESIAN_POINT('Ctrl Pts',(1.7741909281801E-11,-207.38675111262,
9.92453123331945));
#31714=CARTESIAN_POINT('Ctrl Pts',(5.72993077915559,-207.21175111262,9.9245312333092));
#31715=CARTESIAN_POINT('Ctrl Pts',(8.59489616871562,-207.03675111262,4.96226561664435));
#31716=CARTESIAN_POINT('Ctrl Pts',(11.4598615582757,-206.86175111262,-2.04858904854327E-11));
#31717=CARTESIAN_POINT('Ctrl Pts',(8.59489616869788,-206.68675111262,-4.96226561667508));
#31718=CARTESIAN_POINT('Ctrl Pts',(5.7299307791201,-206.51175111262,-9.92453123332968));
#31719=CARTESIAN_POINT('Ctrl Pts',(-1.77583233861944E-11,-206.33675111262,
-9.92453123331945));
#31720=CARTESIAN_POINT('Ctrl Pts',(-5.72993077915558,-206.16175111262,-9.9245312333092));
#31721=CARTESIAN_POINT('Ctrl Pts',(-8.59489616871562,-205.98675111262,-4.96226561664435));
#31722=CARTESIAN_POINT('Ctrl Pts',(-11.4598615582757,-205.81175111262,2.04844870571551E-11));
#31723=CARTESIAN_POINT('Ctrl Pts',(-8.59489616869788,-205.63675111262,4.96226561667508));
#31724=CARTESIAN_POINT('Ctrl Pts',(-5.7299307791201,-205.46175111262,9.92453123332968));
#31725=CARTESIAN_POINT('Ctrl Pts',(1.77571079816536E-11,-205.28675111262,
9.92453123331945));
#31726=CARTESIAN_POINT('Ctrl Pts',(5.72993077915558,-205.11175111262,9.9245312333092));
#31727=CARTESIAN_POINT('Ctrl Pts',(8.59489616871562,-204.93675111262,4.96226561664436));
#31728=CARTESIAN_POINT('Ctrl Pts',(11.4598615582757,-204.76175111262,-2.04830836288775E-11));
#31729=CARTESIAN_POINT('Ctrl Pts',(8.59489616869788,-204.58675111262,-4.96226561667508));
#31730=CARTESIAN_POINT('Ctrl Pts',(5.72993077912011,-204.41175111262,-9.92453123332968));
#31731=CARTESIAN_POINT('Ctrl Pts',(-1.77558925771128E-11,-204.23675111262,
-9.92453123331945));
#31732=CARTESIAN_POINT('Ctrl Pts',(-5.72993077915558,-204.06175111262,-9.9245312333092));
#31733=CARTESIAN_POINT('Ctrl Pts',(-8.59489616871562,-203.88675111262,-4.96226561664436));
#31734=CARTESIAN_POINT('Ctrl Pts',(-11.4598615582757,-203.71175111262,2.04816802005999E-11));
#31735=CARTESIAN_POINT('Ctrl Pts',(-8.59489616869788,-203.53675111262,4.96226561667508));
#31736=CARTESIAN_POINT('Ctrl Pts',(-5.72993077912011,-203.36175111262,9.92453123332968));
#31737=CARTESIAN_POINT('Ctrl Pts',(1.77194181547037E-11,-203.18675111262,
9.92453123331945));
#31738=CARTESIAN_POINT('Ctrl Pts',(5.72993077915558,-203.01175111262,9.9245312333092));
#31739=CARTESIAN_POINT('Ctrl Pts',(8.59489616871562,-202.83675111262,4.96226561664436));
#31740=CARTESIAN_POINT('Ctrl Pts',(11.4598615582757,-202.66175111262,-2.04802767723223E-11));
#31741=CARTESIAN_POINT('Ctrl Pts',(8.59489616869788,-202.48675111262,-4.96226561667508));
#31742=CARTESIAN_POINT('Ctrl Pts',(5.72993077912011,-202.31175111262,-9.92453123332968));
#31743=CARTESIAN_POINT('Ctrl Pts',(-1.77182027501629E-11,-202.13675111262,
-9.92453123331945));
#31744=CARTESIAN_POINT('Ctrl Pts',(-5.72993077915558,-201.96175111262,-9.9245312333092));
#31745=CARTESIAN_POINT('Ctrl Pts',(-8.59489616871562,-201.78675111262,-4.96226561664436));
#31746=CARTESIAN_POINT('Ctrl Pts',(-11.4598615582757,-201.61175111262,2.04381597371295E-11));
#31747=CARTESIAN_POINT('Ctrl Pts',(-8.59489616869788,-201.43675111262,4.96226561667508));
#31748=CARTESIAN_POINT('Ctrl Pts',(-5.72993077912007,-201.26175111262,9.9245312333297));
#31749=CARTESIAN_POINT('Ctrl Pts',(1.77169873456222E-11,-201.08675111262,
9.92453123331945));
#31750=CARTESIAN_POINT('Ctrl Pts',(5.72993077915558,-200.91175111262,9.9245312333092));
#31751=CARTESIAN_POINT('Ctrl Pts',(8.5948961687156,-200.73675111262,4.96226561664439));
#31752=CARTESIAN_POINT('Ctrl Pts',(11.4598615582757,-200.56175111262,-2.04774699157671E-11));
#31753=CARTESIAN_POINT('Ctrl Pts',(8.5948961686979,-200.38675111262,-4.96226561667505));
#31754=CARTESIAN_POINT('Ctrl Pts',(5.72993077912011,-200.21175111262,-9.92453123332968));
#31755=CARTESIAN_POINT('Ctrl Pts',(-1.77510309589497E-11,-200.03675111262,
-9.92453123331945));
#31756=CARTESIAN_POINT('Ctrl Pts',(-5.72993077915554,-199.86175111262,-9.92453123330922));
#31757=CARTESIAN_POINT('Ctrl Pts',(-8.59489616871562,-199.68675111262,-4.96226561664436));
#31758=CARTESIAN_POINT('Ctrl Pts',(-11.4598615582757,-199.51175111262,2.04353528805743E-11));
#31759=CARTESIAN_POINT('Ctrl Pts',(-8.59489616869788,-199.33675111262,4.96226561667507));
#31760=CARTESIAN_POINT('Ctrl Pts',(-5.72993077912008,-199.16175111262,9.9245312333297));
#31761=CARTESIAN_POINT('Ctrl Pts',(1.77145565365406E-11,-198.98675111262,
9.92453123331945));
#31762=CARTESIAN_POINT('Ctrl Pts',(5.72993077915557,-198.81175111262,9.9245312333092));
#31763=CARTESIAN_POINT('Ctrl Pts',(8.5948961687156,-198.63675111262,4.96226561664439));
#31764=CARTESIAN_POINT('Ctrl Pts',(11.4598615582757,-198.46175111262,-2.04746630592119E-11));
#31765=CARTESIAN_POINT('Ctrl Pts',(8.5948961686979,-198.28675111262,-4.96226561667504));
#31766=CARTESIAN_POINT('Ctrl Pts',(5.72993077912011,-198.11175111262,-9.92453123332968));
#31767=CARTESIAN_POINT('Ctrl Pts',(-1.77486001498681E-11,-197.93675111262,
-9.92453123331945));
#31768=CARTESIAN_POINT('Ctrl Pts',(-5.72993077915554,-197.76175111262,-9.92453123330922));
#31769=CARTESIAN_POINT('Ctrl Pts',(-8.59489616871562,-197.58675111262,-4.96226561664436));
#31770=CARTESIAN_POINT('Ctrl Pts',(-11.4598615582757,-197.41175111262,2.04325460240191E-11));
#31771=CARTESIAN_POINT('Ctrl Pts',(-8.59489616869789,-197.23675111262,4.96226561667507));
#31772=CARTESIAN_POINT('Ctrl Pts',(-5.72993077912015,-197.06175111262,9.92453123332966));
#31773=CARTESIAN_POINT('Ctrl Pts',(1.7712125727459E-11,-196.88675111262,
9.92453123331945));
#31774=CARTESIAN_POINT('Ctrl Pts',(5.72993077915557,-196.71175111262,9.9245312333092));
#31775=CARTESIAN_POINT('Ctrl Pts',(8.5948961687156,-196.53675111262,4.9622656166444));
#31776=CARTESIAN_POINT('Ctrl Pts',(11.4598615582757,-196.36175111262,-2.04718562026567E-11));
#31777=CARTESIAN_POINT('Ctrl Pts',(8.5948961686979,-196.18675111262,-4.96226561667504));
#31778=CARTESIAN_POINT('Ctrl Pts',(5.72993077912011,-196.01175111262,-9.92453123332968));
#31779=CARTESIAN_POINT('Ctrl Pts',(-1.77461693407865E-11,-195.83675111262,
-9.92453123331945));
#31780=CARTESIAN_POINT('Ctrl Pts',(-5.72993077915554,-195.66175111262,-9.92453123330922));
#31781=CARTESIAN_POINT('Ctrl Pts',(-8.59489616871562,-195.48675111262,-4.96226561664437));
#31782=CARTESIAN_POINT('Ctrl Pts',(-11.4598615582757,-195.31175111262,2.04297391674638E-11));
#31783=CARTESIAN_POINT('Ctrl Pts',(-8.59489616869789,-195.13675111262,4.96226561667507));
#31784=CARTESIAN_POINT('Ctrl Pts',(-5.72993077912015,-194.96175111262,9.92453123332965));
#31785=CARTESIAN_POINT('Ctrl Pts',(1.77096949183774E-11,-194.78675111262,
9.92453123331945));
#31786=CARTESIAN_POINT('Ctrl Pts',(5.72993077915557,-194.61175111262,9.9245312333092));
#31787=CARTESIAN_POINT('Ctrl Pts',(8.5948961687156,-194.43675111262,4.9622656166444));
#31788=CARTESIAN_POINT('Ctrl Pts',(11.4598615582757,-194.26175111262,-2.04690493461015E-11));
#31789=CARTESIAN_POINT('Ctrl Pts',(8.5948961686979,-194.08675111262,-4.96226561667504));
#31790=CARTESIAN_POINT('Ctrl Pts',(5.72993077912012,-193.91175111262,-9.92453123332967));
#31791=CARTESIAN_POINT('Ctrl Pts',(-1.76732204959683E-11,-193.73675111262,
-9.92453123331945));
#31792=CARTESIAN_POINT('Ctrl Pts',(-5.72993077915553,-193.56175111262,-9.92453123330922));
#31793=CARTESIAN_POINT('Ctrl Pts',(-8.59489616871561,-193.38675111262,-4.96226561664437));
#31794=CARTESIAN_POINT('Ctrl Pts',(-11.4598615582757,-193.21175111262,2.04269323109086E-11));
#31795=CARTESIAN_POINT('Ctrl Pts',(-8.59489616869789,-193.03675111262,4.96226561667507));
#31796=CARTESIAN_POINT('Ctrl Pts',(-5.72993077912015,-192.86175111262,9.92453123332965));
#31797=CARTESIAN_POINT('Ctrl Pts',(1.77072641092958E-11,-192.68675111262,
9.92453123331945));
#31798=CARTESIAN_POINT('Ctrl Pts',(5.7299307791555,-192.51175111262,9.92453123330925));
#31799=CARTESIAN_POINT('Ctrl Pts',(8.5948961687156,-192.33675111262,4.9622656166444));
#31800=CARTESIAN_POINT('Ctrl Pts',(11.4598615582757,-192.16175111262,-2.04662424895463E-11));
#31801=CARTESIAN_POINT('Ctrl Pts',(8.59489616869791,-191.98675111262,-4.96226561667504));
#31802=CARTESIAN_POINT('Ctrl Pts',(5.72993077912012,-191.81175111262,-9.92453123332967));
#31803=CARTESIAN_POINT('Ctrl Pts',(-1.76707896868867E-11,-191.63675111262,
-9.92453123331945));
#31804=CARTESIAN_POINT('Ctrl Pts',(-5.72993077915553,-191.46175111262,-9.92453123330923));
#31805=CARTESIAN_POINT('Ctrl Pts',(-8.59489616871561,-191.28675111262,-4.96226561664437));
#31806=CARTESIAN_POINT('Ctrl Pts',(-11.4598615582757,-191.11175111262,2.04241254543534E-11));
#31807=CARTESIAN_POINT('Ctrl Pts',(-8.59489616869789,-190.93675111262,4.96226561667507));
#31808=CARTESIAN_POINT('Ctrl Pts',(-5.72993077912009,-190.76175111262,9.9245312333297));
#31809=CARTESIAN_POINT('Ctrl Pts',(1.76343152644776E-11,-190.58675111262,
9.92453123331945));
#31810=CARTESIAN_POINT('Ctrl Pts',(5.72993077915549,-190.41175111262,9.92453123330925));
#31811=CARTESIAN_POINT('Ctrl Pts',(8.5948961687156,-190.23675111262,4.9622656166444));
#31812=CARTESIAN_POINT('Ctrl Pts',(11.4598615582757,-190.06175111262,-2.04634356329911E-11));
#31813=CARTESIAN_POINT('Ctrl Pts',(8.59489616869787,-189.88675111262,-4.9622656166751));
#31814=CARTESIAN_POINT('Ctrl Pts',(5.72993077912019,-189.71175111262,-9.92453123332963));
#31815=CARTESIAN_POINT('Ctrl Pts',(-1.76683588778051E-11,-189.53675111262,
-9.92453123331945));
#31816=CARTESIAN_POINT('Ctrl Pts',(-5.72993077915553,-189.36175111262,-9.92453123330923));
#31817=CARTESIAN_POINT('Ctrl Pts',(-8.59489616871561,-189.18675111262,-4.96226561664437));
#31818=CARTESIAN_POINT('Ctrl Pts',(-11.4598615582757,-189.01175111262,2.05027458116287E-11));
#31819=CARTESIAN_POINT('Ctrl Pts',(-8.59489616869793,-188.83675111262,4.962265616675));
#31820=CARTESIAN_POINT('Ctrl Pts',(-5.72993077912016,-188.66175111262,9.92453123332965));
#31821=CARTESIAN_POINT('Ctrl Pts',(1.77024024911326E-11,-188.48675111262,
9.92453123331945));
#31822=CARTESIAN_POINT('Ctrl Pts',(5.72993077915556,-188.31175111262,9.92453123330921));
#31823=CARTESIAN_POINT('Ctrl Pts',(8.59489616871556,-188.13675111262,4.96226561664446));
#31824=CARTESIAN_POINT('Ctrl Pts',(11.4598615582757,-187.96175111262,-2.03792015626054E-11));
#31825=CARTESIAN_POINT('Ctrl Pts',(8.59489616869791,-187.78675111262,-4.96226561667503));
#31826=CARTESIAN_POINT('Ctrl Pts',(5.72993077912012,-187.61175111262,-9.92453123332967));
#31827=CARTESIAN_POINT('Ctrl Pts',(-1.77364461044601E-11,-187.43675111262,
-9.92453123331945));
#31828=CARTESIAN_POINT('Ctrl Pts',(-5.72993077915546,-187.26175111262,-9.92453123330927));
#31829=CARTESIAN_POINT('Ctrl Pts',(-8.59489616871558,-187.08675111262,-4.96226561664444));
#31830=CARTESIAN_POINT('Ctrl Pts',(-11.4598615582757,-186.91175111262,2.0418511741243E-11));
#31831=CARTESIAN_POINT('Ctrl Pts',(-8.59489616869789,-186.73675111262,4.96226561667506));
#31832=CARTESIAN_POINT('Ctrl Pts',(-5.72993077912009,-186.56175111262,9.92453123332969));
#31833=CARTESIAN_POINT('Ctrl Pts',(1.76294536463145E-11,-186.38675111262,
9.92453123331945));
#31834=CARTESIAN_POINT('Ctrl Pts',(5.72993077915549,-186.21175111262,9.92453123330925));
#31835=CARTESIAN_POINT('Ctrl Pts',(8.59489616871559,-186.03675111262,4.96226561664441));
#31836=CARTESIAN_POINT('Ctrl Pts',(11.4598615582757,-185.86175111262,-2.04578219198807E-11));
#31837=CARTESIAN_POINT('Ctrl Pts',(8.59489616869787,-185.68675111262,-4.96226561667509));
#31838=CARTESIAN_POINT('Ctrl Pts',(5.7299307791202,-185.51175111262,-9.92453123332963));
#31839=CARTESIAN_POINT('Ctrl Pts',(-1.7663497259642E-11,-185.33675111262,
-9.92453123331945));
#31840=CARTESIAN_POINT('Ctrl Pts',(-5.72993077915552,-185.16175111262,-9.92453123330923));
#31841=CARTESIAN_POINT('Ctrl Pts',(-8.59489616871561,-184.98675111262,-4.96226561664438));
#31842=CARTESIAN_POINT('Ctrl Pts',(-11.4598615582757,-184.81175111262,2.03342776708573E-11));
#31843=CARTESIAN_POINT('Ctrl Pts',(-8.59489616869793,-184.63675111262,4.962265616675));
#31844=CARTESIAN_POINT('Ctrl Pts',(-5.72993077912016,-184.46175111262,9.92453123332965));
#31845=CARTESIAN_POINT('Ctrl Pts',(1.76975408729695E-11,-184.28675111262,
9.92453123331945));
#31846=CARTESIAN_POINT('Ctrl Pts',(5.72993077915556,-184.11175111262,9.92453123330921));
#31847=CARTESIAN_POINT('Ctrl Pts',(8.59489616871556,-183.93675111262,4.96226561664447));
#31848=CARTESIAN_POINT('Ctrl Pts',(11.4598615582757,-183.76175111262,-2.0373587849495E-11));
#31849=CARTESIAN_POINT('Ctrl Pts',(8.59489616869791,-183.58675111262,-4.96226561667503));
#31850=CARTESIAN_POINT('Ctrl Pts',(5.72993077912013,-183.41175111262,-9.92453123332967));
#31851=CARTESIAN_POINT('Ctrl Pts',(-1.7731584486297E-11,-183.23675111262,
-9.92453123331945));
#31852=CARTESIAN_POINT('Ctrl Pts',(-5.72993077915545,-183.06175111262,-9.92453123330927));
#31853=CARTESIAN_POINT('Ctrl Pts',(-8.59489616871557,-182.88675111262,-4.96226561664444));
#31854=CARTESIAN_POINT('Ctrl Pts',(-11.4598615582757,-182.71175111262,2.04128980281326E-11));
#31855=CARTESIAN_POINT('Ctrl Pts',(-8.59489616869789,-182.53675111262,4.96226561667506));
#31856=CARTESIAN_POINT('Ctrl Pts',(-5.72993077912009,-182.36175111262,9.92453123332969));
#31857=CARTESIAN_POINT('Ctrl Pts',(1.76245920281513E-11,-182.18675111262,
9.92453123331945));
#31858=CARTESIAN_POINT('Ctrl Pts',(5.72993077915548,-182.01175111262,9.92453123330925));
#31859=CARTESIAN_POINT('Ctrl Pts',(8.59489616871559,-181.83675111262,4.96226561664441));
#31860=CARTESIAN_POINT('Ctrl Pts',(11.4598615582757,-181.66175111262,-2.04522082067703E-11));
#31861=CARTESIAN_POINT('Ctrl Pts',(8.59489616869794,-181.48675111262,-4.96226561667497));
#31862=CARTESIAN_POINT('Ctrl Pts',(5.7299307791202,-181.31175111262,-9.92453123332963));
#31863=CARTESIAN_POINT('Ctrl Pts',(-1.76586356414788E-11,-181.13675111262,
-9.92453123331945));
#31864=CARTESIAN_POINT('Ctrl Pts',(-5.72993077915552,-180.96175111262,-9.92453123330923));
#31865=CARTESIAN_POINT('Ctrl Pts',(-8.59489616871561,-180.78675111262,-4.96226561664438));
#31866=CARTESIAN_POINT('Ctrl Pts',(-11.4598615582757,-180.61175111262,2.03286639577469E-11));
#31867=CARTESIAN_POINT('Ctrl Pts',(-8.59489616869793,-180.43675111262,4.96226561667499));
#31868=CARTESIAN_POINT('Ctrl Pts',(-5.72993077912017,-180.26175111262,9.92453123332965));
#31869=CARTESIAN_POINT('Ctrl Pts',(1.76926792548063E-11,-180.08675111262,
9.92453123331945));
#31870=CARTESIAN_POINT('Ctrl Pts',(5.72993077915555,-179.91175111262,9.92453123330921));
#31871=CARTESIAN_POINT('Ctrl Pts',(8.59489616871555,-179.73675111262,4.96226561664447));
#31872=CARTESIAN_POINT('Ctrl Pts',(11.4598615582757,-179.56175111262,-2.03679741363846E-11));
#31873=CARTESIAN_POINT('Ctrl Pts',(8.59489616869791,-179.38675111262,-4.96226561667503));
#31874=CARTESIAN_POINT('Ctrl Pts',(5.72993077912013,-179.21175111262,-9.92453123332966));
#31875=CARTESIAN_POINT('Ctrl Pts',(-1.77267228681338E-11,-179.03675111262,
-9.92453123331945));
#31876=CARTESIAN_POINT('Ctrl Pts',(-5.72993077915545,-178.86175111262,-9.92453123330928));
#31877=CARTESIAN_POINT('Ctrl Pts',(-8.59489616871557,-178.68675111262,-4.96226561664444));
#31878=CARTESIAN_POINT('Ctrl Pts',(-11.4598615582757,-178.51175111262,2.04072843150222E-11));
#31879=CARTESIAN_POINT('Ctrl Pts',(-8.5948961686979,-178.33675111262,4.96226561667505));
#31880=CARTESIAN_POINT('Ctrl Pts',(-5.72993077912024,-178.16175111262,9.92453123332961));
#31881=CARTESIAN_POINT('Ctrl Pts',(1.76197304099881E-11,-177.98675111262,
9.92453123331945));
#31882=CARTESIAN_POINT('Ctrl Pts',(5.72993077915548,-177.81175111262,9.92453123330926));
#31883=CARTESIAN_POINT('Ctrl Pts',(8.59489616871559,-177.63675111262,4.96226561664442));
#31884=CARTESIAN_POINT('Ctrl Pts',(11.4598615582757,-177.46175111262,-2.04465944936599E-11));
#31885=CARTESIAN_POINT('Ctrl Pts',(8.59489616869795,-177.28675111262,-4.96226561667496));
#31886=CARTESIAN_POINT('Ctrl Pts',(5.72993077912021,-177.11175111262,-9.92453123332962));
#31887=CARTESIAN_POINT('Ctrl Pts',(-1.76537740233156E-11,-176.93675111262,
-9.92453123331945));
#31888=CARTESIAN_POINT('Ctrl Pts',(-5.72993077915551,-176.76175111262,-9.92453123330924));
#31889=CARTESIAN_POINT('Ctrl Pts',(-8.5948961687156,-176.58675111262,-4.96226561664438));
#31890=CARTESIAN_POINT('Ctrl Pts',(-11.4598615582757,-176.41175111262,2.03230502446365E-11));
#31891=CARTESIAN_POINT('Ctrl Pts',(-8.59489616869793,-176.23675111262,4.96226561667499));
#31892=CARTESIAN_POINT('Ctrl Pts',(-5.72993077912017,-176.06175111262,9.92453123332964));
#31893=CARTESIAN_POINT('Ctrl Pts',(1.76878176366431E-11,-175.88675111262,
9.92453123331945));
#31894=CARTESIAN_POINT('Ctrl Pts',(5.72993077915541,-175.71175111262,9.9245312333093));
#31895=CARTESIAN_POINT('Ctrl Pts',(8.59489616871555,-175.53675111262,4.96226561664448));
#31896=CARTESIAN_POINT('Ctrl Pts',(11.4598615582757,-175.36175111262,-2.03623604232742E-11));
#31897=CARTESIAN_POINT('Ctrl Pts',(8.59489616869791,-175.18675111262,-4.96226561667502));
#31898=CARTESIAN_POINT('Ctrl Pts',(5.72993077912014,-175.01175111262,-9.92453123332966));
#31899=CARTESIAN_POINT('Ctrl Pts',(-1.75808251784975E-11,-174.83675111262,
-9.92453123331945));
#31900=CARTESIAN_POINT('Ctrl Pts',(-5.72993077915544,-174.66175111262,-9.92453123330928));
#31901=CARTESIAN_POINT('Ctrl Pts',(-8.59489616871557,-174.48675111262,-4.96226561664445));
#31902=CARTESIAN_POINT('Ctrl Pts',(-11.4598615582757,-174.31175111262,2.04016706019118E-11));
#31903=CARTESIAN_POINT('Ctrl Pts',(-8.5948961686979,-174.13675111262,4.96226561667505));
#31904=CARTESIAN_POINT('Ctrl Pts',(-5.72993077912025,-173.96175111262,9.9245312333296));
#31905=CARTESIAN_POINT('Ctrl Pts',(1.7614868791825E-11,-173.78675111262,
9.92453123331945));
#31906=CARTESIAN_POINT('Ctrl Pts',(5.72993077915548,-173.61175111262,9.92453123330926));
#31907=CARTESIAN_POINT('Ctrl Pts',(8.59489616871558,-173.43675111262,4.96226561664442));
#31908=CARTESIAN_POINT('Ctrl Pts',(11.4598615582757,-173.26175111262,-2.04409807805495E-11));
#31909=CARTESIAN_POINT('Ctrl Pts',(8.59489616869795,-173.08675111262,-4.96226561667496));
#31910=CARTESIAN_POINT('Ctrl Pts',(5.72993077912021,-172.91175111262,-9.92453123332962));
#31911=CARTESIAN_POINT('Ctrl Pts',(-1.76489124051525E-11,-172.73675111262,
-9.92453123331945));
#31912=CARTESIAN_POINT('Ctrl Pts',(-5.72993077915551,-172.56175111262,-9.92453123330924));
#31913=CARTESIAN_POINT('Ctrl Pts',(-8.59489616871553,-172.38675111262,-4.96226561664451));
#31914=CARTESIAN_POINT('Ctrl Pts',(-11.4598615582757,-172.21175111262,2.03174365315261E-11));
#31915=CARTESIAN_POINT('Ctrl Pts',(-8.59489616869793,-172.03675111262,4.96226561667499));
#31916=CARTESIAN_POINT('Ctrl Pts',(-5.72993077912018,-171.86175111262,9.92453123332964));
#31917=CARTESIAN_POINT('Ctrl Pts',(1.768295601848E-11,-171.68675111262,
9.92453123331945));
#31918=CARTESIAN_POINT('Ctrl Pts',(5.7299307791554,-171.51175111262,9.9245312333093));
#31919=CARTESIAN_POINT('Ctrl Pts',(8.59489616871555,-171.33675111262,4.96226561664448));
#31920=CARTESIAN_POINT('Ctrl Pts',(11.4598615582757,-171.16175111262,-2.03567467101638E-11));
#31921=CARTESIAN_POINT('Ctrl Pts',(8.59489616869792,-170.98675111262,-4.96226561667502));
#31922=CARTESIAN_POINT('Ctrl Pts',(5.72993077912014,-170.81175111262,-9.92453123332966));
#31923=CARTESIAN_POINT('Ctrl Pts',(-1.75759635603343E-11,-170.63675111262,
-9.92453123331945));
#31924=CARTESIAN_POINT('Ctrl Pts',(-5.72993077915544,-170.46175111262,-9.92453123330928));
#31925=CARTESIAN_POINT('Ctrl Pts',(-8.59489616871556,-170.28675111262,-4.96226561664445));
#31926=CARTESIAN_POINT('Ctrl Pts',(-11.4598615582757,-170.11175111262,2.03960568888014E-11));
#31927=CARTESIAN_POINT('Ctrl Pts',(-8.5948961686979,-169.93675111262,4.96226561667505));
#31928=CARTESIAN_POINT('Ctrl Pts',(-5.72993077912011,-169.76175111262,9.92453123332968));
#31929=CARTESIAN_POINT('Ctrl Pts',(1.76100071736618E-11,-169.58675111262,
9.92453123331945));
#31930=CARTESIAN_POINT('Ctrl Pts',(5.72993077915533,-169.41175111262,9.92453123330935));
#31931=CARTESIAN_POINT('Ctrl Pts',(8.59489616871558,-169.23675111262,4.96226561664442));
#31932=CARTESIAN_POINT('Ctrl Pts',(11.4598615582757,-169.06175111262,-2.02725126397781E-11));
#31933=CARTESIAN_POINT('Ctrl Pts',(8.59489616869788,-168.88675111262,-4.96226561667507));
#31934=CARTESIAN_POINT('Ctrl Pts',(5.72993077912022,-168.71175111262,-9.92453123332962));
#31935=CARTESIAN_POINT('Ctrl Pts',(-1.75030147155161E-11,-168.53675111262,
-9.92453123331945));
#31936=CARTESIAN_POINT('Ctrl Pts',(-5.7299307791555,-168.36175111262,-9.92453123330924));
#31937=CARTESIAN_POINT('Ctrl Pts',(-8.59489616871553,-168.18675111262,-4.96226561664451));
#31938=CARTESIAN_POINT('Ctrl Pts',(-11.4598615582757,-168.01175111262,2.04746772460767E-11));
#31939=CARTESIAN_POINT('Ctrl Pts',(-8.59489616869794,-167.83675111262,4.96226561667498));
#31940=CARTESIAN_POINT('Ctrl Pts',(-5.72993077912033,-167.66175111262,9.92453123332955));
#31941=CARTESIAN_POINT('Ctrl Pts',(1.76780944003168E-11,-167.48675111262,
9.92453123331945));
#31942=CARTESIAN_POINT('Ctrl Pts',(5.7299307791554,-167.31175111262,9.92453123330931));
#31943=CARTESIAN_POINT('Ctrl Pts',(8.59489616871562,-167.13675111262,4.96226561664436));
#31944=CARTESIAN_POINT('Ctrl Pts',(11.4598615582757,-166.96175111262,-2.03511329970534E-11));
#31945=CARTESIAN_POINT('Ctrl Pts',(8.59489616869799,-166.78675111262,-4.96226561667489));
#31946=CARTESIAN_POINT('Ctrl Pts',(5.72993077912015,-166.61175111262,-9.92453123332966));
#31947=CARTESIAN_POINT('Ctrl Pts',(-1.75711019421711E-11,-166.43675111262,
-9.92453123331945));
#31948=CARTESIAN_POINT('Ctrl Pts',(-5.72993077915557,-166.26175111262,-9.9245312333092));
#31949=CARTESIAN_POINT('Ctrl Pts',(-8.59489616871556,-166.08675111262,-4.96226561664446));
#31950=CARTESIAN_POINT('Ctrl Pts',(-11.4598615582757,-165.91175111262,2.022758874803E-11));
#31951=CARTESIAN_POINT('Ctrl Pts',(-8.5948961686979,-165.73675111262,4.96226561667504));
#31952=CARTESIAN_POINT('Ctrl Pts',(-5.72993077912025,-165.56175111262,9.9245312333296));
#31953=CARTESIAN_POINT('Ctrl Pts',(1.77461816269718E-11,-165.38675111262,
9.92453123331945));
#31954=CARTESIAN_POINT('Ctrl Pts',(5.72993077915547,-165.21175111262,9.92453123330927));
#31955=CARTESIAN_POINT('Ctrl Pts',(8.59489616871551,-165.03675111262,4.96226561664455));
#31956=CARTESIAN_POINT('Ctrl Pts',(11.4598615582757,-164.86175111262,-2.04297533543287E-11));
#31957=CARTESIAN_POINT('Ctrl Pts',(8.59489616869796,-164.68675111262,-4.96226561667495));
#31958=CARTESIAN_POINT('Ctrl Pts',(5.72993077912036,-164.51175111262,-9.92453123332954));
#31959=CARTESIAN_POINT('Ctrl Pts',(-1.76391891688261E-11,-164.33675111262,
-9.92453123331945));
#31960=CARTESIAN_POINT('Ctrl Pts',(-5.72993077915536,-164.16175111262,-9.92453123330933));
#31961=CARTESIAN_POINT('Ctrl Pts',(-8.5948961687156,-163.98675111262,-4.9622656166444));
#31962=CARTESIAN_POINT('Ctrl Pts',(-11.4598615582757,-163.81175111262,2.03062091053053E-11));
#31963=CARTESIAN_POINT('Ctrl Pts',(-8.59489616869801,-163.63675111262,4.96226561667486));
#31964=CARTESIAN_POINT('Ctrl Pts',(-5.72993077912019,-163.46175111262,9.92453123332963));
#31965=CARTESIAN_POINT('Ctrl Pts',(1.75321967106804E-11,-163.28675111262,
9.92453123331945));
#31966=CARTESIAN_POINT('Ctrl Pts',(5.72993077915553,-163.11175111262,9.92453123330922));
#31967=CARTESIAN_POINT('Ctrl Pts',(8.59489616871554,-162.93675111262,4.96226561664449));
#31968=CARTESIAN_POINT('Ctrl Pts',(11.4598615582757,-162.76175111262,-2.0182664856282E-11));
#31969=CARTESIAN_POINT('Ctrl Pts',(8.59489616869792,-162.58675111262,-4.96226561667501));
#31970=CARTESIAN_POINT('Ctrl Pts',(5.7299307791203,-162.41175111262,-9.92453123332957));
#31971=CARTESIAN_POINT('Ctrl Pts',(-1.77072763954811E-11,-162.23675111262,
-9.92453123331945));
#31972=CARTESIAN_POINT('Ctrl Pts',(-5.72993077915543,-162.06175111262,-9.92453123330929));
#31973=CARTESIAN_POINT('Ctrl Pts',(-8.59489616871549,-161.88675111262,-4.96226561664458));
#31974=CARTESIAN_POINT('Ctrl Pts',(-11.4598615582757,-161.71175111262,2.03848294625806E-11));
#31975=CARTESIAN_POINT('Ctrl Pts',(-8.59489616869798,-161.53675111262,4.96226561667492));
#31976=CARTESIAN_POINT('Ctrl Pts',(-5.72993077912012,-161.36175111262,9.92453123332967));
#31977=CARTESIAN_POINT('Ctrl Pts',(1.76002839373354E-11,-161.18675111262,
9.92453123331945));
#31978=CARTESIAN_POINT('Ctrl Pts',(5.72993077915532,-161.01175111262,9.92453123330935));
#31979=CARTESIAN_POINT('Ctrl Pts',(8.59489616871558,-160.83675111262,4.96226561664443));
#31980=CARTESIAN_POINT('Ctrl Pts',(11.4598615582757,-160.66175111262,-2.02612852135573E-11));
#31981=CARTESIAN_POINT('Ctrl Pts',(8.59489616869789,-160.48675111262,-4.96226561667507));
#31982=CARTESIAN_POINT('Ctrl Pts',(5.72993077912023,-160.31175111262,-9.92453123332961));
#31983=CARTESIAN_POINT('Ctrl Pts',(-1.74932914791898E-11,-160.13675111262,
-9.92453123331945));
#31984=CARTESIAN_POINT('Ctrl Pts',(-5.72993077915549,-159.96175111262,-9.92453123330925));
#31985=CARTESIAN_POINT('Ctrl Pts',(-8.59489616871553,-159.78675111262,-4.96226561664452));
#31986=CARTESIAN_POINT('Ctrl Pts',(-11.4598615582757,-159.61175111262,2.04634498198559E-11));
#31987=CARTESIAN_POINT('Ctrl Pts',(-8.59489616869794,-159.43675111262,4.96226561667497));
#31988=CARTESIAN_POINT('Ctrl Pts',(-5.72993077912033,-159.26175111262,9.92453123332955));
#31989=CARTESIAN_POINT('Ctrl Pts',(1.76683711639905E-11,-159.08675111262,
9.92453123331945));
#31990=CARTESIAN_POINT('Ctrl Pts',(5.72993077915539,-158.91175111262,9.92453123330931));
#31991=CARTESIAN_POINT('Ctrl Pts',(8.59489616871561,-158.73675111262,4.96226561664437));
#31992=CARTESIAN_POINT('Ctrl Pts',(11.4598615582757,-158.56175111262,-2.03399055708326E-11));
#31993=CARTESIAN_POINT('Ctrl Pts',(8.594896168698,-158.38675111262,-4.96226561667488));
#31994=CARTESIAN_POINT('Ctrl Pts',(5.72993077912016,-158.21175111262,-9.92453123332965));
#31995=CARTESIAN_POINT('Ctrl Pts',(-1.75613787058448E-11,-158.03675111262,
-9.92453123331945));
#31996=CARTESIAN_POINT('Ctrl Pts',(-5.72993077915528,-157.86175111262,-9.92453123330937));
#31997=CARTESIAN_POINT('Ctrl Pts',(-8.59489616871556,-157.68675111262,-4.96226561664446));
#31998=CARTESIAN_POINT('Ctrl Pts',(-11.4598615582757,-157.51175111262,2.02163613218092E-11));
#31999=CARTESIAN_POINT('Ctrl Pts',(-8.59489616869791,-157.33675111262,4.96226561667503));
#32000=CARTESIAN_POINT('Ctrl Pts',(-5.72993077912026,-157.16175111262,9.92453123332959));
#32001=CARTESIAN_POINT('Ctrl Pts',(1.74543862476991E-11,-156.98675111262,
9.92453123331945));
#32002=CARTESIAN_POINT('Ctrl Pts',(5.72993077915546,-156.81175111262,9.92453123330927));
#32003=CARTESIAN_POINT('Ctrl Pts',(8.5948961687155,-156.63675111262,4.96226561664456));
#32004=CARTESIAN_POINT('Ctrl Pts',(11.4598615582757,-156.46175111262,-2.04185259281078E-11));
#32005=CARTESIAN_POINT('Ctrl Pts',(8.59489616869796,-156.28675111262,-4.96226561667494));
#32006=CARTESIAN_POINT('Ctrl Pts',(5.72993077912037,-156.11175111262,-9.92453123332953));
#32007=CARTESIAN_POINT('Ctrl Pts',(-1.76294659324998E-11,-155.93675111262,
-9.92453123331945));
#32008=CARTESIAN_POINT('Ctrl Pts',(-5.72993077915535,-155.76175111262,-9.92453123330933));
#32009=CARTESIAN_POINT('Ctrl Pts',(-8.59489616871559,-155.58675111262,-4.96226561664441));
#32010=CARTESIAN_POINT('Ctrl Pts',(-11.4598615582757,-155.41175111262,2.02949816790845E-11));
#32011=CARTESIAN_POINT('Ctrl Pts',(-8.59489616869802,-155.23675111262,4.96226561667485));
#32012=CARTESIAN_POINT('Ctrl Pts',(-5.7299307791202,-155.06175111262,9.92453123332963));
#32013=CARTESIAN_POINT('Ctrl Pts',(1.75224734743541E-11,-154.88675111262,
9.92453123331945));
#32014=CARTESIAN_POINT('Ctrl Pts',(5.72993077915552,-154.71175111262,9.92453123330923));
#32015=CARTESIAN_POINT('Ctrl Pts',(8.59489616871554,-154.53675111262,4.9622656166445));
#32016=CARTESIAN_POINT('Ctrl Pts',(11.4598615582757,-154.36175111262,-2.01714374300612E-11));
#32017=CARTESIAN_POINT('Ctrl Pts',(8.59489616869793,-154.18675111262,-4.962265616675));
#32018=CARTESIAN_POINT('Ctrl Pts',(5.7299307791203,-154.01175111262,-9.92453123332957));
#32019=CARTESIAN_POINT('Ctrl Pts',(-1.76975531591548E-11,-153.83675111262,
-9.92453123331945));
#32020=CARTESIAN_POINT('Ctrl Pts',(-5.72993077915542,-153.66175111262,-9.92453123330929));
#32021=CARTESIAN_POINT('Ctrl Pts',(-8.59489616871549,-153.48675111262,-4.96226561664459));
#32022=CARTESIAN_POINT('Ctrl Pts',(-11.4598615582757,-153.31175111262,2.03736020363598E-11));
#32023=CARTESIAN_POINT('Ctrl Pts',(-8.59489616869798,-153.13675111262,4.96226561667491));
#32024=CARTESIAN_POINT('Ctrl Pts',(-5.72993077912013,-152.96175111262,9.92453123332967));
#32025=CARTESIAN_POINT('Ctrl Pts',(1.75905607010091E-11,-152.78675111262,
9.92453123331945));
#32026=CARTESIAN_POINT('Ctrl Pts',(5.72993077915531,-152.61175111262,9.92453123330936));
#32027=CARTESIAN_POINT('Ctrl Pts',(8.59489616871557,-152.43675111262,4.96226561664444));
#32028=CARTESIAN_POINT('Ctrl Pts',(11.4598615582757,-152.26175111262,-2.02500577873365E-11));
#32029=CARTESIAN_POINT('Ctrl Pts',(8.59489616869789,-152.08675111262,-4.96226561667506));
#32030=CARTESIAN_POINT('Ctrl Pts',(5.72993077912024,-151.91175111262,-9.92453123332961));
#32031=CARTESIAN_POINT('Ctrl Pts',(-1.74835682428634E-11,-151.73675111262,
-9.92453123331945));
#32032=CARTESIAN_POINT('Ctrl Pts',(-5.72993077915548,-151.56175111262,-9.92453123330925));
#32033=CARTESIAN_POINT('Ctrl Pts',(-8.59489616871552,-151.38675111262,-4.96226561664453));
#32034=CARTESIAN_POINT('Ctrl Pts',(-11.4598615582757,-151.21175111262,2.01265135383131E-11));
#32035=CARTESIAN_POINT('Ctrl Pts',(-8.59489616869794,-151.03675111262,4.96226561667497));
#32036=CARTESIAN_POINT('Ctrl Pts',(-5.72993077912034,-150.86175111262,9.92453123332955));
#32037=CARTESIAN_POINT('Ctrl Pts',(1.76586479276641E-11,-150.68675111262,
9.92453123331945));
#32038=CARTESIAN_POINT('Ctrl Pts',(5.72993077915538,-150.51175111262,9.92453123330931));
#32039=CARTESIAN_POINT('Ctrl Pts',(8.59489616871547,-150.33675111262,4.96226561664462));
#32040=CARTESIAN_POINT('Ctrl Pts',(11.4598615582757,-150.16175111262,-2.03286781446117E-11));
#32041=CARTESIAN_POINT('Ctrl Pts',(8.594896168698,-149.98675111262,-4.96226561667487));
#32042=CARTESIAN_POINT('Ctrl Pts',(5.72993077912017,-149.81175111262,-9.92453123332965));
#32043=CARTESIAN_POINT('Ctrl Pts',(-1.75516554695184E-11,-149.63675111262,
-9.92453123331945));
#32044=CARTESIAN_POINT('Ctrl Pts',(-5.72993077915527,-149.46175111262,-9.92453123330938));
#32045=CARTESIAN_POINT('Ctrl Pts',(-8.59489616871555,-149.28675111262,-4.96226561664447));
#32046=CARTESIAN_POINT('Ctrl Pts',(-11.4598615582757,-149.11175111262,2.02051338955884E-11));
#32047=CARTESIAN_POINT('Ctrl Pts',(-8.59489616869791,-148.93675111262,4.96226561667503));
#32048=CARTESIAN_POINT('Ctrl Pts',(-5.72993077912027,-148.76175111262,9.92453123332958));
#32049=CARTESIAN_POINT('Ctrl Pts',(1.74446630113728E-11,-148.58675111262,
9.92453123331945));
#32050=CARTESIAN_POINT('Ctrl Pts',(5.72993077915545,-148.41175111262,9.92453123330928));
#32051=CARTESIAN_POINT('Ctrl Pts',(8.5948961687155,-148.23675111262,4.96226561664457));
#32052=CARTESIAN_POINT('Ctrl Pts',(11.4598615582757,-148.06175111262,-2.0407298501887E-11));
#32053=CARTESIAN_POINT('Ctrl Pts',(8.59489616869797,-147.88675111262,-4.96226561667493));
#32054=CARTESIAN_POINT('Ctrl Pts',(5.72993077912038,-147.71175111262,-9.92453123332952));
#32055=CARTESIAN_POINT('Ctrl Pts',(-1.76197426961734E-11,-147.53675111262,
-9.92453123331945));
#32056=CARTESIAN_POINT('Ctrl Pts',(-5.72993077915534,-147.36175111262,-9.92453123330934));
#32057=CARTESIAN_POINT('Ctrl Pts',(-8.59489616871559,-147.18675111262,-4.96226561664442));
#32058=CARTESIAN_POINT('Ctrl Pts',(-11.4598615582757,-147.01175111262,2.02837542528637E-11));
#32059=CARTESIAN_POINT('Ctrl Pts',(-8.59489616869802,-146.83675111262,4.96226561667484));
#32060=CARTESIAN_POINT('Ctrl Pts',(-5.72993077912021,-146.66175111262,9.92453123332962));
#32061=CARTESIAN_POINT('Ctrl Pts',(1.75127502380278E-11,-146.48675111262,
9.92453123331945));
#32062=CARTESIAN_POINT('Ctrl Pts',(5.72993077915551,-146.31175111262,9.92453123330924));
#32063=CARTESIAN_POINT('Ctrl Pts',(8.59489616871553,-146.13675111262,4.96226561664451));
#32064=CARTESIAN_POINT('Ctrl Pts',(11.4598615582757,-145.96175111262,-2.01602100038404E-11));
#32065=CARTESIAN_POINT('Ctrl Pts',(8.59489616869793,-145.78675111262,-4.96226561667499));
#32066=CARTESIAN_POINT('Ctrl Pts',(5.72993077912031,-145.61175111262,-9.92453123332956));
#32067=CARTESIAN_POINT('Ctrl Pts',(-1.76878299228285E-11,-145.43675111262,
-9.92453123331945));
#32068=CARTESIAN_POINT('Ctrl Pts',(-5.72993077915541,-145.26175111262,-9.9245312333093));
#32069=CARTESIAN_POINT('Ctrl Pts',(-8.59489616871548,-145.08675111262,-4.9622656166446));
#32070=CARTESIAN_POINT('Ctrl Pts',(-11.4598615582757,-144.91175111262,2.0362374610139E-11));
#32071=CARTESIAN_POINT('Ctrl Pts',(-8.59489616869799,-144.73675111262,4.9622656166749));
#32072=CARTESIAN_POINT('Ctrl Pts',(-5.72993077912042,-144.56175111262,9.9245312333295));
#32073=CARTESIAN_POINT('Ctrl Pts',(1.75808374646828E-11,-144.38675111262,
9.92453123331945));
#32074=CARTESIAN_POINT('Ctrl Pts',(5.7299307791553,-144.21175111262,9.92453123330936));
#32075=CARTESIAN_POINT('Ctrl Pts',(8.59489616871557,-144.03675111262,4.96226561664445));
#32076=CARTESIAN_POINT('Ctrl Pts',(11.4598615582757,-143.86175111262,-2.02388303611156E-11));
#32077=CARTESIAN_POINT('Ctrl Pts',(8.59489616869804,-143.68675111262,-4.96226561667481));
#32078=CARTESIAN_POINT('Ctrl Pts',(5.72993077912025,-143.51175111262,-9.9245312333296));
#32079=CARTESIAN_POINT('Ctrl Pts',(-1.74738450065371E-11,-143.33675111262,
-9.92453123331945));
#32080=CARTESIAN_POINT('Ctrl Pts',(-5.72993077915548,-143.16175111262,-9.92453123330926));
#32081=CARTESIAN_POINT('Ctrl Pts',(-8.59489616871551,-142.98675111262,-4.96226561664454));
#32082=CARTESIAN_POINT('Ctrl Pts',(-11.4598615582757,-142.81175111262,2.01152861120923E-11));
#32083=CARTESIAN_POINT('Ctrl Pts',(-8.59489616869795,-142.63675111262,4.96226561667496));
#32084=CARTESIAN_POINT('Ctrl Pts',(-5.72993077912035,-142.46175111262,9.92453123332954));
#32085=CARTESIAN_POINT('Ctrl Pts',(1.76489246913378E-11,-142.28675111262,
9.92453123331945));
#32086=CARTESIAN_POINT('Ctrl Pts',(5.72993077915537,-142.11175111262,9.92453123330932));
#32087=CARTESIAN_POINT('Ctrl Pts',(8.59489616871546,-141.93675111262,4.96226561664463));
#32088=CARTESIAN_POINT('Ctrl Pts',(11.4598615582757,-141.76175111262,-2.03174507183909E-11));
#32089=CARTESIAN_POINT('Ctrl Pts',(8.59489616869801,-141.58675111262,-4.96226561667487));
#32090=CARTESIAN_POINT('Ctrl Pts',(5.72993077912018,-141.41175111262,-9.92453123332964));
#32091=CARTESIAN_POINT('Ctrl Pts',(-1.75419322331921E-11,-141.23675111262,
-9.92453123331945));
#32092=CARTESIAN_POINT('Ctrl Pts',(-5.72993077915526,-141.06175111262,-9.92453123330938));
#32093=CARTESIAN_POINT('Ctrl Pts',(-8.59489616871555,-140.88675111262,-4.96226561664448));
#32094=CARTESIAN_POINT('Ctrl Pts',(-11.4598615582757,-140.71175111262,2.01939064693676E-11));
#32095=CARTESIAN_POINT('Ctrl Pts',(-8.59489616869792,-140.53675111262,4.96226561667502));
#32096=CARTESIAN_POINT('Ctrl Pts',(-5.72993077912029,-140.36175111262,9.92453123332958));
#32097=CARTESIAN_POINT('Ctrl Pts',(1.74349397750464E-11,-140.18675111262,
9.92453123331945));
#32098=CARTESIAN_POINT('Ctrl Pts',(5.72993077915544,-140.01175111262,9.92453123330928));
#32099=CARTESIAN_POINT('Ctrl Pts',(8.59489616871549,-139.83675111262,4.96226561664457));
#32100=CARTESIAN_POINT('Ctrl Pts',(11.4598615582757,-139.66175111262,-2.03960710756662E-11));
#32101=CARTESIAN_POINT('Ctrl Pts',(8.59489616869797,-139.48675111262,-4.96226561667492));
#32102=CARTESIAN_POINT('Ctrl Pts',(5.72993077912039,-139.31175111262,-9.92453123332952));
#32103=CARTESIAN_POINT('Ctrl Pts',(-1.76100194598471E-11,-139.13675111262,
-9.92453123331945));
#32104=CARTESIAN_POINT('Ctrl Pts',(-5.72993077915533,-138.96175111262,-9.92453123330935));
#32105=CARTESIAN_POINT('Ctrl Pts',(-8.59489616871544,-138.78675111262,-4.96226561664467));
#32106=CARTESIAN_POINT('Ctrl Pts',(-11.4598615582757,-138.61175111262,2.02725268266429E-11));
#32107=CARTESIAN_POINT('Ctrl Pts',(-8.59489616869802,-138.43675111262,4.96226561667483));
#32108=CARTESIAN_POINT('Ctrl Pts',(-5.72993077912022,-138.26175111262,9.92453123332962));
#32109=CARTESIAN_POINT('Ctrl Pts',(1.75030270017014E-11,-138.08675111262,
9.92453123331945));
#32110=CARTESIAN_POINT('Ctrl Pts',(5.72993077915522,-137.91175111262,9.92453123330941));
#32111=CARTESIAN_POINT('Ctrl Pts',(8.59489616871553,-137.73675111262,4.96226561664451));
#32112=CARTESIAN_POINT('Ctrl Pts',(11.4598615582757,-137.56175111262,-2.01489825776195E-11));
#32113=CARTESIAN_POINT('Ctrl Pts',(8.59489616869794,-137.38675111262,-4.96226561667498));
#32114=CARTESIAN_POINT('Ctrl Pts',(5.72993077912033,-137.21175111262,-9.92453123332955));
#32115=CARTESIAN_POINT('Ctrl Pts',(-1.73960345435557E-11,-137.03675111262,
-9.92453123331945));
#32116=CARTESIAN_POINT('Ctrl Pts',(-5.7299307791554,-136.86175111262,-9.92453123330931));
#32117=CARTESIAN_POINT('Ctrl Pts',(-8.59489616871548,-136.68675111262,-4.96226561664461));
#32118=CARTESIAN_POINT('Ctrl Pts',(-11.4598615582757,-136.51175111262,2.03511471839182E-11));
#32119=CARTESIAN_POINT('Ctrl Pts',(-8.59489616869799,-136.33675111262,4.96226561667489));
#32120=CARTESIAN_POINT('Ctrl Pts',(-5.72993077912043,-136.16175111262,9.92453123332949));
#32121=CARTESIAN_POINT('Ctrl Pts',(1.75711142283564E-11,-135.98675111262,
9.92453123331945));
#32122=CARTESIAN_POINT('Ctrl Pts',(5.72993077915529,-135.81175111262,9.92453123330937));
#32123=CARTESIAN_POINT('Ctrl Pts',(8.59489616871556,-135.63675111262,4.96226561664446));
#32124=CARTESIAN_POINT('Ctrl Pts',(11.4598615582757,-135.46175111262,-2.02276029348948E-11));
#32125=CARTESIAN_POINT('Ctrl Pts',(8.59489616869805,-135.28675111262,-4.9622656166748));
#32126=CARTESIAN_POINT('Ctrl Pts',(5.72993077912025,-135.11175111262,-9.9245312333296));
#32127=CARTESIAN_POINT('Ctrl Pts',(-1.74641217702107E-11,-134.93675111262,
-9.92453123331945));
#32128=CARTESIAN_POINT('Ctrl Pts',(-5.72993077915547,-134.76175111262,-9.92453123330927));
#32129=CARTESIAN_POINT('Ctrl Pts',(-8.59489616871551,-134.58675111262,-4.96226561664455));
#32130=CARTESIAN_POINT('Ctrl Pts',(-11.4598615582757,-134.41175111262,2.01040586858715E-11));
#32131=CARTESIAN_POINT('Ctrl Pts',(-8.59489616869796,-134.23675111262,4.96226561667495));
#32132=CARTESIAN_POINT('Ctrl Pts',(-5.72993077912036,-134.06175111262,9.92453123332954));
#32133=CARTESIAN_POINT('Ctrl Pts',(1.76392014550114E-11,-133.88675111262,
9.92453123331945));
#32134=CARTESIAN_POINT('Ctrl Pts',(5.72993077915536,-133.71175111262,9.92453123330933));
#32135=CARTESIAN_POINT('Ctrl Pts',(8.59489616871546,-133.53675111262,4.96226561664464));
#32136=CARTESIAN_POINT('Ctrl Pts',(11.4598615582757,-133.36175111262,-2.03062232921701E-11));
#32137=CARTESIAN_POINT('Ctrl Pts',(8.59489616869801,-133.18675111262,-4.96226561667486));
#32138=CARTESIAN_POINT('Ctrl Pts',(5.72993077912019,-133.01175111262,-9.92453123332963));
#32139=CARTESIAN_POINT('Ctrl Pts',(-1.75322089968658E-11,-132.83675111262,
-9.92453123331945));
#32140=CARTESIAN_POINT('Ctrl Pts',(-5.72993077915525,-132.66175111262,-9.92453123330939));
#32141=CARTESIAN_POINT('Ctrl Pts',(-8.59489616871554,-132.48675111262,-4.96226561664449));
#32142=CARTESIAN_POINT('Ctrl Pts',(-11.4598615582757,-132.31175111262,2.01826790431468E-11));
#32143=CARTESIAN_POINT('Ctrl Pts',(-8.59489616869806,-132.13675111262,4.96226561667476));
#32144=CARTESIAN_POINT('Ctrl Pts',(-5.7299307791203,-131.96175111262,9.92453123332957));
#32145=CARTESIAN_POINT('Ctrl Pts',(1.74252165387201E-11,-131.78675111262,
9.92453123331945));
#32146=CARTESIAN_POINT('Ctrl Pts',(5.72993077915543,-131.61175111262,9.92453123330929));
#32147=CARTESIAN_POINT('Ctrl Pts',(8.59489616871549,-131.43675111262,4.96226561664458));
#32148=CARTESIAN_POINT('Ctrl Pts',(11.4598615582757,-131.26175111262,-2.00591347941234E-11));
#32149=CARTESIAN_POINT('Ctrl Pts',(8.59489616869798,-131.08675111262,-4.96226561667492));
#32150=CARTESIAN_POINT('Ctrl Pts',(5.7299307791204,-130.91175111262,-9.92453123332951));
#32151=CARTESIAN_POINT('Ctrl Pts',(-1.76002962235208E-11,-130.73675111262,
-9.92453123331945));
#32152=CARTESIAN_POINT('Ctrl Pts',(-5.72993077915532,-130.56175111262,-9.92453123330935));
#32153=CARTESIAN_POINT('Ctrl Pts',(-8.59489616871544,-130.38675111262,-4.96226561664468));
#32154=CARTESIAN_POINT('Ctrl Pts',(-11.4598615582757,-130.21175111262,2.02612994004221E-11));
#32155=CARTESIAN_POINT('Ctrl Pts',(-8.59489616869803,-130.03675111262,4.96226561667482));
#32156=CARTESIAN_POINT('Ctrl Pts',(-5.72993077912023,-129.86175111262,9.92453123332961));
#32157=CARTESIAN_POINT('Ctrl Pts',(1.74933037653751E-11,-129.68675111262,
9.92453123331945));
#32158=CARTESIAN_POINT('Ctrl Pts',(5.72993077915521,-129.51175111262,9.92453123330941));
#32159=CARTESIAN_POINT('Ctrl Pts',(8.59489616871553,-129.33675111262,4.96226561664452));
#32160=CARTESIAN_POINT('Ctrl Pts',(11.4598615582757,-129.16175111262,-2.01377551513987E-11));
#32161=CARTESIAN_POINT('Ctrl Pts',(8.59489616869794,-128.98675111262,-4.96226561667497));
#32162=CARTESIAN_POINT('Ctrl Pts',(5.72993077912033,-128.81175111262,-9.92453123332955));
#32163=CARTESIAN_POINT('Ctrl Pts',(-1.73863113072294E-11,-128.63675111262,
-9.92453123331945));
#32164=CARTESIAN_POINT('Ctrl Pts',(-5.72993077915539,-128.46175111262,-9.92453123330931));
#32165=CARTESIAN_POINT('Ctrl Pts',(-8.59489616871547,-128.28675111262,-4.96226561664462));
#32166=CARTESIAN_POINT('Ctrl Pts',(-11.4598615582757,-128.11175111262,2.03399197576974E-11));
#32167=CARTESIAN_POINT('Ctrl Pts',(-8.59489616869799,-127.93675111262,4.96226561667488));
#32168=CARTESIAN_POINT('Ctrl Pts',(-5.72993077912044,-127.76175111262,9.92453123332949));
#32169=CARTESIAN_POINT('Ctrl Pts',(1.75613909920301E-11,-127.58675111262,
9.92453123331945));
#32170=CARTESIAN_POINT('Ctrl Pts',(5.72993077915528,-127.41175111262,9.92453123330937));
#32171=CARTESIAN_POINT('Ctrl Pts',(8.59489616871556,-127.23675111262,4.96226561664446));
#32172=CARTESIAN_POINT('Ctrl Pts',(11.4598615582757,-127.06175111262,-2.0216375508674E-11));
#32173=CARTESIAN_POINT('Ctrl Pts',(8.59489616869791,-126.88675111262,-4.96226561667503));
#32174=CARTESIAN_POINT('Ctrl Pts',(5.72993077912055,-126.71175111262,-9.92453123332943));
#32175=CARTESIAN_POINT('Ctrl Pts',(-1.74543985338844E-11,-126.53675111262,
-9.92453123331945));
#32176=CARTESIAN_POINT('Ctrl Pts',(-5.72993077915546,-126.36175111262,-9.92453123330927));
#32177=CARTESIAN_POINT('Ctrl Pts',(-8.59489616871537,-126.18675111262,-4.9622656166448));
#32178=CARTESIAN_POINT('Ctrl Pts',(-11.4598615582757,-126.01175111262,2.00928312596507E-11));
#32179=CARTESIAN_POINT('Ctrl Pts',(-8.59489616869796,-125.83675111262,4.96226561667494));
#32180=CARTESIAN_POINT('Ctrl Pts',(-5.72993077912009,-125.66175111262,9.92453123332969));
#32181=CARTESIAN_POINT('Ctrl Pts',(1.73474060757387E-11,-125.48675111262,
9.92453123331945));
#32182=CARTESIAN_POINT('Ctrl Pts',(5.72993077915535,-125.31175111262,9.92453123330933));
#32183=CARTESIAN_POINT('Ctrl Pts',(8.59489616871559,-125.13675111262,4.96226561664441));
#32184=CARTESIAN_POINT('Ctrl Pts',(11.4598615582757,-124.96175111262,-1.99692870106273E-11));
#32185=CARTESIAN_POINT('Ctrl Pts',(8.59489616869802,-124.78675111262,-4.96226561667485));
#32186=CARTESIAN_POINT('Ctrl Pts',(5.7299307791202,-124.61175111262,-9.92453123332963));
#32187=CARTESIAN_POINT('Ctrl Pts',(-1.7240413617593E-11,-124.43675111262,
-9.92453123331945));
#32188=CARTESIAN_POINT('Ctrl Pts',(-5.72993077915524,-124.26175111262,-9.92453123330939));
#32189=CARTESIAN_POINT('Ctrl Pts',(-8.59489616871554,-124.08675111262,-4.9622656166445));
#32190=CARTESIAN_POINT('Ctrl Pts',(-11.4598615582757,-123.91175111262,2.04971604722479E-11));
#32191=CARTESIAN_POINT('Ctrl Pts',(-8.59489616869807,-123.73675111262,4.96226561667476));
#32192=CARTESIAN_POINT('Ctrl Pts',(-5.7299307791203,-123.56175111262,9.92453123332957));
#32193=CARTESIAN_POINT('Ctrl Pts',(1.76975654453401E-11,-123.38675111262,
9.92453123331945));
#32194=CARTESIAN_POINT('Ctrl Pts',(5.72993077915513,-123.21175111262,9.92453123330946));
#32195=CARTESIAN_POINT('Ctrl Pts',(8.59489616871549,-123.03675111262,4.96226561664459));
#32196=CARTESIAN_POINT('Ctrl Pts',(11.4598615582757,-122.86175111262,-2.03736162232246E-11));
#32197=CARTESIAN_POINT('Ctrl Pts',(8.59489616869812,-122.68675111262,-4.96226561667466));
#32198=CARTESIAN_POINT('Ctrl Pts',(5.72993077912041,-122.51175111262,-9.92453123332951));
#32199=CARTESIAN_POINT('Ctrl Pts',(-1.75905729871944E-11,-122.33675111262,
-9.92453123331945));
#32200=CARTESIAN_POINT('Ctrl Pts',(-5.72993077915503,-122.16175111262,-9.92453123330952));
#32201=CARTESIAN_POINT('Ctrl Pts',(-8.59489616871543,-121.98675111262,-4.96226561664468));
#32202=CARTESIAN_POINT('Ctrl Pts',(-11.4598615582757,-121.81175111262,2.02500719742013E-11));
#32203=CARTESIAN_POINT('Ctrl Pts',(-8.59489616869789,-121.63675111262,4.96226561667506));
#32204=CARTESIAN_POINT('Ctrl Pts',(-5.72993077912052,-121.46175111262,9.92453123332944));
#32205=CARTESIAN_POINT('Ctrl Pts',(1.74835805290487E-11,-121.28675111262,
9.92453123331945));
#32206=CARTESIAN_POINT('Ctrl Pts',(5.72993077915548,-121.11175111262,9.92453123330925));
#32207=CARTESIAN_POINT('Ctrl Pts',(8.59489616871538,-120.93675111262,4.96226561664478));
#32208=CARTESIAN_POINT('Ctrl Pts',(11.4598615582757,-120.76175111262,-2.01265277251779E-11));
#32209=CARTESIAN_POINT('Ctrl Pts',(8.59489616869794,-120.58675111262,-4.96226561667497));
#32210=CARTESIAN_POINT('Ctrl Pts',(5.72993077912063,-120.41175111262,-9.92453123332938));
#32211=CARTESIAN_POINT('Ctrl Pts',(-1.73765880709031E-11,-120.23675111262,
-9.92453123331945));
#32212=CARTESIAN_POINT('Ctrl Pts',(-5.72993077915538,-120.06175111262,-9.92453123330931));
#32213=CARTESIAN_POINT('Ctrl Pts',(-8.59489616871561,-119.88675111262,-4.96226561664438));
#32214=CARTESIAN_POINT('Ctrl Pts',(-11.4598615582757,-119.71175111262,2.00029834761546E-11));
#32215=CARTESIAN_POINT('Ctrl Pts',(-8.594896168698,-119.53675111262,4.96226561667487));
#32216=CARTESIAN_POINT('Ctrl Pts',(-5.72993077912017,-119.36175111262,9.92453123332965));
#32217=CARTESIAN_POINT('Ctrl Pts',(1.72695956127574E-11,-119.18675111262,
9.92453123331945));
#32218=CARTESIAN_POINT('Ctrl Pts',(5.72993077915527,-119.01175111262,9.92453123330938));
#32219=CARTESIAN_POINT('Ctrl Pts',(8.59489616871555,-118.83675111262,4.96226561664447));
#32220=CARTESIAN_POINT('Ctrl Pts',(11.4598615582757,-118.66175111262,-1.98794392271312E-11));
#32221=CARTESIAN_POINT('Ctrl Pts',(8.59489616869805,-118.48675111262,-4.96226561667478));
#32222=CARTESIAN_POINT('Ctrl Pts',(5.72993077912027,-118.31175111262,-9.92453123332958));
#32223=CARTESIAN_POINT('Ctrl Pts',(-1.77267474405044E-11,-118.13675111262,
-9.92453123331945));
#32224=CARTESIAN_POINT('Ctrl Pts',(-5.72993077915516,-117.96175111262,-9.92453123330944));
#32225=CARTESIAN_POINT('Ctrl Pts',(-8.5948961687155,-117.78675111262,-4.96226561664457));
#32226=CARTESIAN_POINT('Ctrl Pts',(-11.4598615582757,-117.61175111262,2.04073126887518E-11));
#32227=CARTESIAN_POINT('Ctrl Pts',(-8.59489616869811,-117.43675111262,4.96226561667469));
#32228=CARTESIAN_POINT('Ctrl Pts',(-5.72993077912038,-117.26175111262,9.92453123332952));
#32229=CARTESIAN_POINT('Ctrl Pts',(1.76197549823588E-11,-117.08675111262,
9.92453123331945));
#32230=CARTESIAN_POINT('Ctrl Pts',(5.72993077915506,-116.91175111262,9.9245312333095));
#32231=CARTESIAN_POINT('Ctrl Pts',(8.59489616871545,-116.73675111262,4.96226561664466));
#32232=CARTESIAN_POINT('Ctrl Pts',(11.4598615582757,-116.56175111262,-2.02837684397285E-11));
#32233=CARTESIAN_POINT('Ctrl Pts',(8.59489616869816,-116.38675111262,-4.96226561667459));
#32234=CARTESIAN_POINT('Ctrl Pts',(5.72993077912049,-116.21175111262,-9.92453123332946));
#32235=CARTESIAN_POINT('Ctrl Pts',(-1.75127625242131E-11,-116.03675111262,
-9.92453123331945));
#32236=CARTESIAN_POINT('Ctrl Pts',(-5.72993077915551,-115.86175111262,-9.92453123330924));
#32237=CARTESIAN_POINT('Ctrl Pts',(-8.59489616871539,-115.68675111262,-4.96226561664475));
#32238=CARTESIAN_POINT('Ctrl Pts',(-11.4598615582757,-115.51175111262,2.01602241907052E-11));
#32239=CARTESIAN_POINT('Ctrl Pts',(-8.59489616869793,-115.33675111262,4.96226561667499));
#32240=CARTESIAN_POINT('Ctrl Pts',(-5.7299307791206,-115.16175111262,9.9245312333294));
#32241=CARTESIAN_POINT('Ctrl Pts',(1.74057700660674E-11,-114.98675111262,
9.92453123331945));
#32242=CARTESIAN_POINT('Ctrl Pts',(5.72993077915541,-114.81175111262,9.9245312333093));
#32243=CARTESIAN_POINT('Ctrl Pts',(8.59489616871534,-114.63675111262,4.96226561664484));
#32244=CARTESIAN_POINT('Ctrl Pts',(11.4598615582757,-114.46175111262,-2.00366799416818E-11));
#32245=CARTESIAN_POINT('Ctrl Pts',(8.59489616869799,-114.28675111262,-4.9622656166749));
#32246=CARTESIAN_POINT('Ctrl Pts',(5.72993077912014,-114.11175111262,-9.92453123332966));
#32247=CARTESIAN_POINT('Ctrl Pts',(-1.72987776079217E-11,-113.93675111262,
-9.92453123331945));
#32248=CARTESIAN_POINT('Ctrl Pts',(-5.7299307791553,-113.76175111262,-9.92453123330936));
#32249=CARTESIAN_POINT('Ctrl Pts',(-8.59489616871557,-113.58675111262,-4.96226561664445));
#32250=CARTESIAN_POINT('Ctrl Pts',(-11.4598615582757,-113.41175111262,1.99131356926585E-11));
#32251=CARTESIAN_POINT('Ctrl Pts',(-8.59489616869804,-113.23675111262,4.96226561667481));
#32252=CARTESIAN_POINT('Ctrl Pts',(-5.72993077912025,-113.06175111262,9.9245312333296));
#32253=CARTESIAN_POINT('Ctrl Pts',(1.7191785149776E-11,-112.88675111262,
9.92453123331945));
#32254=CARTESIAN_POINT('Ctrl Pts',(5.72993077915519,-112.71175111262,9.92453123330942));
#32255=CARTESIAN_POINT('Ctrl Pts',(8.59489616871551,-112.53675111262,4.96226561664454));
#32256=CARTESIAN_POINT('Ctrl Pts',(11.4598615582757,-112.36175111262,-2.04410091542791E-11));
#32257=CARTESIAN_POINT('Ctrl Pts',(8.59489616869809,-112.18675111262,-4.96226561667471));
#32258=CARTESIAN_POINT('Ctrl Pts',(5.72993077912035,-112.01175111262,-9.92453123332954));
#32259=CARTESIAN_POINT('Ctrl Pts',(-1.76489369775231E-11,-111.83675111262,
-9.92453123331945));
#32260=CARTESIAN_POINT('Ctrl Pts',(-5.72993077915509,-111.66175111262,-9.92453123330948));
#32261=CARTESIAN_POINT('Ctrl Pts',(-8.59489616871546,-111.48675111262,-4.96226561664463));
#32262=CARTESIAN_POINT('Ctrl Pts',(-11.4598615582757,-111.31175111262,2.03174649052557E-11));
#32263=CARTESIAN_POINT('Ctrl Pts',(-8.59489616869815,-111.13675111262,4.96226561667462));
#32264=CARTESIAN_POINT('Ctrl Pts',(-5.72993077912046,-110.96175111262,9.92453123332948));
#32265=CARTESIAN_POINT('Ctrl Pts',(1.75419445193774E-11,-110.78675111262,
9.92453123331945));
#32266=CARTESIAN_POINT('Ctrl Pts',(5.72993077915554,-110.61175111262,9.92453123330922));
#32267=CARTESIAN_POINT('Ctrl Pts',(8.59489616871541,-110.43675111262,4.96226561664473));
#32268=CARTESIAN_POINT('Ctrl Pts',(11.4598615582757,-110.26175111262,-2.01939206562324E-11));
#32269=CARTESIAN_POINT('Ctrl Pts',(8.59489616869792,-110.08675111262,-4.96226561667502));
#32270=CARTESIAN_POINT('Ctrl Pts',(5.72993077912057,-109.91175111262,-9.92453123332941));
#32271=CARTESIAN_POINT('Ctrl Pts',(-1.74349520612317E-11,-109.73675111262,
-9.92453123331945));
#32272=CARTESIAN_POINT('Ctrl Pts',(-5.72993077915544,-109.56175111262,-9.92453123330928));
#32273=CARTESIAN_POINT('Ctrl Pts',(-8.59489616871535,-109.38675111262,-4.96226561664482));
#32274=CARTESIAN_POINT('Ctrl Pts',(-11.4598615582757,-109.21175111262,2.00703764072091E-11));
#32275=CARTESIAN_POINT('Ctrl Pts',(-8.59489616869797,-109.03675111262,4.96226561667492));
#32276=CARTESIAN_POINT('Ctrl Pts',(-5.72993077912067,-108.86175111262,9.92453123332935));
#32277=CARTESIAN_POINT('Ctrl Pts',(1.73279596030861E-11,-108.68675111262,
9.92453123331945));
#32278=CARTESIAN_POINT('Ctrl Pts',(5.72993077915533,-108.51175111262,9.92453123330935));
#32279=CARTESIAN_POINT('Ctrl Pts',(8.59489616871558,-108.33675111262,4.96226561664442));
#32280=CARTESIAN_POINT('Ctrl Pts',(11.4598615582757,-108.16175111262,-1.99468321581857E-11));
#32281=CARTESIAN_POINT('Ctrl Pts',(8.59489616869802,-107.98675111262,-4.96226561667483));
#32282=CARTESIAN_POINT('Ctrl Pts',(5.72993077912022,-107.81175111262,-9.92453123332962));
#32283=CARTESIAN_POINT('Ctrl Pts',(-1.72209671449404E-11,-107.63675111262,
-9.92453123331945));
#32284=CARTESIAN_POINT('Ctrl Pts',(-5.72993077915522,-107.46175111262,-9.92453123330941));
#32285=CARTESIAN_POINT('Ctrl Pts',(-8.59489616871553,-107.28675111262,-4.96226561664451));
#32286=CARTESIAN_POINT('Ctrl Pts',(-11.4598615582757,-107.11175111262,1.98232879091624E-11));
#32287=CARTESIAN_POINT('Ctrl Pts',(-8.59489616869808,-106.93675111262,4.96226561667474));
#32288=CARTESIAN_POINT('Ctrl Pts',(-5.72993077912033,-106.76175111262,9.92453123332955));
#32289=CARTESIAN_POINT('Ctrl Pts',(1.76781189726874E-11,-106.58675111262,
9.92453123331945));
#32290=CARTESIAN_POINT('Ctrl Pts',(5.72993077915512,-106.41175111262,9.92453123330947));
#32291=CARTESIAN_POINT('Ctrl Pts',(8.59489616871548,-106.23675111262,4.96226561664461));
#32292=CARTESIAN_POINT('Ctrl Pts',(11.4598615582757,-106.06175111262,-2.0351161370783E-11));
#32293=CARTESIAN_POINT('Ctrl Pts',(8.59489616869813,-105.88675111262,-4.96226561667465));
#32294=CARTESIAN_POINT('Ctrl Pts',(5.72993077912043,-105.71175111262,-9.92453123332949));
#32295=CARTESIAN_POINT('Ctrl Pts',(-1.75711265145418E-11,-105.53675111262,
-9.92453123331945));
#32296=CARTESIAN_POINT('Ctrl Pts',(-5.72993077915501,-105.36175111262,-9.92453123330953));
#32297=CARTESIAN_POINT('Ctrl Pts',(-8.59489616871542,-105.18675111262,-4.9622656166447));
#32298=CARTESIAN_POINT('Ctrl Pts',(-11.4598615582757,-105.01175111262,2.02276171217596E-11));
#32299=CARTESIAN_POINT('Ctrl Pts',(-8.5948961686979,-104.83675111262,4.96226561667504));
#32300=CARTESIAN_POINT('Ctrl Pts',(-5.72993077912054,-104.66175111262,9.92453123332943));
#32301=CARTESIAN_POINT('Ctrl Pts',(1.74641340563961E-11,-104.48675111262,
9.92453123331945));
#32302=CARTESIAN_POINT('Ctrl Pts',(5.72993077915547,-104.31175111262,9.92453123330927));
#32303=CARTESIAN_POINT('Ctrl Pts',(8.59489616871537,-104.13675111262,4.96226561664479));
#32304=CARTESIAN_POINT('Ctrl Pts',(11.4598615582757,-103.96175111262,-2.01040728727363E-11));
#32305=CARTESIAN_POINT('Ctrl Pts',(8.59489616869796,-103.78675111262,-4.96226561667495));
#32306=CARTESIAN_POINT('Ctrl Pts',(5.72993077912064,-103.61175111262,-9.92453123332937));
#32307=CARTESIAN_POINT('Ctrl Pts',(-1.73571415982504E-11,-103.43675111262,
-9.92453123331945));
#32308=CARTESIAN_POINT('Ctrl Pts',(-5.72993077915536,-103.26175111262,-9.92453123330933));
#32309=CARTESIAN_POINT('Ctrl Pts',(-8.59489616871532,-103.08675111262,-4.96226561664489));
#32310=CARTESIAN_POINT('Ctrl Pts',(-11.4598615582757,-102.91175111262,1.9980528623713E-11));
#32311=CARTESIAN_POINT('Ctrl Pts',(-8.59489616869801,-102.73675111262,4.96226561667486));
#32312=CARTESIAN_POINT('Ctrl Pts',(-5.72993077912019,-102.56175111262,9.92453123332963));
#32313=CARTESIAN_POINT('Ctrl Pts',(1.72501491401047E-11,-102.38675111262,
9.92453123331945));
#32314=CARTESIAN_POINT('Ctrl Pts',(5.72993077915525,-102.21175111262,9.92453123330939));
#32315=CARTESIAN_POINT('Ctrl Pts',(8.59489616871554,-102.03675111262,4.96226561664449));
#32316=CARTESIAN_POINT('Ctrl Pts',(11.4598615582757,-101.86175111262,-1.98569843746896E-11));
#32317=CARTESIAN_POINT('Ctrl Pts',(8.59489616869806,-101.68675111262,-4.96226561667476));
#32318=CARTESIAN_POINT('Ctrl Pts',(5.7299307791203,-101.51175111262,-9.92453123332957));
#32319=CARTESIAN_POINT('Ctrl Pts',(-1.7143156681959E-11,-101.33675111262,
-9.92453123331945));
#32320=CARTESIAN_POINT('Ctrl Pts',(-5.72993077915514,-101.16175111262,-9.92453123330945));
#32321=CARTESIAN_POINT('Ctrl Pts',(-8.59489616871549,-100.98675111262,-4.96226561664458));
#32322=CARTESIAN_POINT('Ctrl Pts',(-11.4598615582757,-100.81175111262,2.03848578363102E-11));
#32323=CARTESIAN_POINT('Ctrl Pts',(-8.59489616869812,-100.63675111262,4.96226561667467));
#32324=CARTESIAN_POINT('Ctrl Pts',(-5.7299307791204,-100.46175111262,9.92453123332951));
#32325=CARTESIAN_POINT('Ctrl Pts',(1.76003085097061E-11,-100.28675111262,
9.92453123331945));
#32326=CARTESIAN_POINT('Ctrl Pts',(5.72993077915504,-100.11175111262,9.92453123330951));
#32327=CARTESIAN_POINT('Ctrl Pts',(8.59489616871544,-99.9367511126202,4.96226561664468));
#32328=CARTESIAN_POINT('Ctrl Pts',(11.4598615582757,-99.7617511126202,-2.02613135872869E-11));
#32329=CARTESIAN_POINT('Ctrl Pts',(8.59489616869817,-99.5867511126202,-4.96226561667458));
#32330=CARTESIAN_POINT('Ctrl Pts',(5.72993077912051,-99.4117511126202,-9.92453123332945));
#32331=CARTESIAN_POINT('Ctrl Pts',(-1.74933160515604E-11,-99.2367511126202,
-9.92453123331945));
#32332=CARTESIAN_POINT('Ctrl Pts',(-5.72993077915549,-99.0617511126202,
-9.92453123330925));
#32333=CARTESIAN_POINT('Ctrl Pts',(-8.59489616871538,-98.8867511126202,
-4.96226561664477));
#32334=CARTESIAN_POINT('Ctrl Pts',(-11.4598615582757,-98.7117511126202,
2.01377693382635E-11));
#32335=CARTESIAN_POINT('Ctrl Pts',(-8.59489616869794,-98.5367511126202,
4.96226561667497));
#32336=CARTESIAN_POINT('Ctrl Pts',(-5.72993077912062,-98.3617511126202,
9.92453123332939));
#32337=CARTESIAN_POINT('Ctrl Pts',(1.73863235934147E-11,-98.1867511126202,
9.92453123331945));
#32338=CARTESIAN_POINT('Ctrl Pts',(5.72993077915539,-98.0117511126202,9.92453123330931));
#32339=CARTESIAN_POINT('Ctrl Pts',(8.59489616871533,-97.8367511126202,4.96226561664486));
#32340=CARTESIAN_POINT('Ctrl Pts',(11.4598615582757,-97.6617511126202,-2.00142250892402E-11));
#32341=CARTESIAN_POINT('Ctrl Pts',(8.59489616869799,-97.4867511126202,-4.96226561667488));
#32342=CARTESIAN_POINT('Ctrl Pts',(5.72993077912072,-97.3117511126202,-9.92453123332933));
#32343=CARTESIAN_POINT('Ctrl Pts',(-1.7279331135269E-11,-97.1367511126202,
-9.92453123331945));
#32344=CARTESIAN_POINT('Ctrl Pts',(-5.72993077915528,-96.9617511126202,
-9.92453123330937));
#32345=CARTESIAN_POINT('Ctrl Pts',(-8.59489616871556,-96.7867511126202,
-4.96226561664446));
#32346=CARTESIAN_POINT('Ctrl Pts',(-11.4598615582757,-96.6117511126202,
1.98906808402169E-11));
#32347=CARTESIAN_POINT('Ctrl Pts',(-8.59489616869805,-96.4367511126202,
4.96226561667479));
#32348=CARTESIAN_POINT('Ctrl Pts',(-5.72993077912026,-96.2617511126202,
9.92453123332959));
#32349=CARTESIAN_POINT('Ctrl Pts',(1.71723386771234E-11,-96.0867511126202,
9.92453123331945));
#32350=CARTESIAN_POINT('Ctrl Pts',(5.72993077915517,-95.9117511126202,9.92453123330943));
#32351=CARTESIAN_POINT('Ctrl Pts',(8.5948961687155,-95.7367511126202,4.96226561664456));
#32352=CARTESIAN_POINT('Ctrl Pts',(11.4598615582757,-95.5617511126202,-1.97671365911935E-11));
#32353=CARTESIAN_POINT('Ctrl Pts',(8.5948961686981,-95.3867511126202,-4.9622656166747));
#32354=CARTESIAN_POINT('Ctrl Pts',(5.72993077912037,-95.2117511126202,-9.92453123332953));
#32355=CARTESIAN_POINT('Ctrl Pts',(-1.76294905048704E-11,-95.0367511126202,
-9.92453123331945));
#32356=CARTESIAN_POINT('Ctrl Pts',(-5.72993077915507,-94.8617511126203,
-9.9245312333095));
#32357=CARTESIAN_POINT('Ctrl Pts',(-8.59489616871545,-94.6867511126202,
-4.96226561664465));
#32358=CARTESIAN_POINT('Ctrl Pts',(-11.4598615582757,-94.5117511126202,
2.02950100528141E-11));
#32359=CARTESIAN_POINT('Ctrl Pts',(-8.59489616869816,-94.3367511126202,
4.9622656166746));
#32360=CARTESIAN_POINT('Ctrl Pts',(-5.72993077912048,-94.1617511126202,
9.92453123332946));
#32361=CARTESIAN_POINT('Ctrl Pts',(1.75224980467247E-11,-93.9867511126202,
9.92453123331945));
#32362=CARTESIAN_POINT('Ctrl Pts',(5.72993077915496,-93.8117511126202,9.92453123330956));
#32363=CARTESIAN_POINT('Ctrl Pts',(8.5948961687154,-93.6367511126202,4.96226561664474));
#32364=CARTESIAN_POINT('Ctrl Pts',(11.4598615582757,-93.4617511126202,-2.01714658037908E-11));
#32365=CARTESIAN_POINT('Ctrl Pts',(8.59489616869793,-93.2867511126202,-4.962265616675));
#32366=CARTESIAN_POINT('Ctrl Pts',(5.72993077912059,-93.1117511126202,-9.9245312333294));
#32367=CARTESIAN_POINT('Ctrl Pts',(-1.74155055885791E-11,-92.9367511126202,
-9.92453123331945));
#32368=CARTESIAN_POINT('Ctrl Pts',(-5.72993077915542,-92.7617511126202,
-9.92453123330929));
#32369=CARTESIAN_POINT('Ctrl Pts',(-8.59489616871534,-92.5867511126202,
-4.96226561664484));
#32370=CARTESIAN_POINT('Ctrl Pts',(-11.4598615582757,-92.4117511126203,
2.00479215547674E-11));
#32371=CARTESIAN_POINT('Ctrl Pts',(-8.59489616869798,-92.2367511126202,
4.96226561667491));
#32372=CARTESIAN_POINT('Ctrl Pts',(-5.72993077912069,-92.0617511126202,
9.92453123332934));
#32373=CARTESIAN_POINT('Ctrl Pts',(1.73085131304334E-11,-91.8867511126202,
9.92453123331945));
#32374=CARTESIAN_POINT('Ctrl Pts',(5.72993077915531,-91.7117511126202,9.92453123330936));
#32375=CARTESIAN_POINT('Ctrl Pts',(8.59489616871557,-91.5367511126202,4.96226561664444));
#32376=CARTESIAN_POINT('Ctrl Pts',(11.4598615582757,-91.3617511126203,-1.99243773057441E-11));
#32377=CARTESIAN_POINT('Ctrl Pts',(8.59489616869803,-91.1867511126202,-4.96226561667481));
#32378=CARTESIAN_POINT('Ctrl Pts',(5.72993077912024,-91.0117511126202,-9.92453123332961));
#32379=CARTESIAN_POINT('Ctrl Pts',(-1.72015206722877E-11,-90.8367511126202,
-9.92453123331945));
#32380=CARTESIAN_POINT('Ctrl Pts',(-5.7299307791552,-90.6617511126203,-9.92453123330942));
#32381=CARTESIAN_POINT('Ctrl Pts',(-8.59489616871552,-90.4867511126203,
-4.96226561664453));
#32382=CARTESIAN_POINT('Ctrl Pts',(-11.4598615582757,-90.3117511126203,
1.98008330567208E-11));
#32383=CARTESIAN_POINT('Ctrl Pts',(-8.59489616869809,-90.1367511126202,
4.96226561667472));
#32384=CARTESIAN_POINT('Ctrl Pts',(-5.72993077912034,-89.9617511126202,
9.92453123332955));
#32385=CARTESIAN_POINT('Ctrl Pts',(1.7094528214142E-11,-89.7867511126202,
9.92453123331945));
#32386=CARTESIAN_POINT('Ctrl Pts',(5.7299307791551,-89.6117511126202,9.92453123330948));
#32387=CARTESIAN_POINT('Ctrl Pts',(8.59489616871547,-89.4367511126202,4.96226561664462));
#32388=CARTESIAN_POINT('Ctrl Pts',(11.4598615582757,-89.2617511126203,-2.03287065183413E-11));
#32389=CARTESIAN_POINT('Ctrl Pts',(8.59489616869814,-89.0867511126202,-4.96226561667463));
#32390=CARTESIAN_POINT('Ctrl Pts',(5.72993077912045,-88.9117511126202,-9.92453123332948));
#32391=CARTESIAN_POINT('Ctrl Pts',(-1.75516800418891E-11,-88.7367511126203,
-9.92453123331945));
#32392=CARTESIAN_POINT('Ctrl Pts',(-5.72993077915499,-88.5617511126202,
-9.92453123330954));
#32393=CARTESIAN_POINT('Ctrl Pts',(-8.59489616871541,-88.3867511126203,
-4.96226561664472));
#32394=CARTESIAN_POINT('Ctrl Pts',(-11.4598615582757,-88.2117511126202,
2.0205162269318E-11));
#32395=CARTESIAN_POINT('Ctrl Pts',(-8.5948961686982,-88.0367511126202,4.96226561667454));
#32396=CARTESIAN_POINT('Ctrl Pts',(-5.72993077912056,-87.8617511126203,
9.92453123332942));
#32397=CARTESIAN_POINT('Ctrl Pts',(1.74446875837434E-11,-87.6867511126203,
9.92453123331945));
#32398=CARTESIAN_POINT('Ctrl Pts',(5.72993077915545,-87.5117511126203,9.92453123330928));
#32399=CARTESIAN_POINT('Ctrl Pts',(8.59489616871536,-87.3367511126202,4.96226561664481));
#32400=CARTESIAN_POINT('Ctrl Pts',(11.4598615582757,-87.1617511126203,-2.00816180202947E-11));
#32401=CARTESIAN_POINT('Ctrl Pts',(8.59489616869797,-86.9867511126203,-4.96226561667493));
#32402=CARTESIAN_POINT('Ctrl Pts',(5.72993077912066,-86.8117511126202,-9.92453123332936));
#32403=CARTESIAN_POINT('Ctrl Pts',(-1.73376951255977E-11,-86.6367511126203,
-9.92453123331945));
#32404=CARTESIAN_POINT('Ctrl Pts',(-5.72993077915534,-86.4617511126202,
-9.92453123330934));
#32405=CARTESIAN_POINT('Ctrl Pts',(-8.59489616871531,-86.2867511126203,
-4.9622656166449));
#32406=CARTESIAN_POINT('Ctrl Pts',(-11.4598615582757,-86.1117511126203,
1.99580737712713E-11));
#32407=CARTESIAN_POINT('Ctrl Pts',(-8.59489616869802,-85.9367511126203,
4.96226561667484));
#32408=CARTESIAN_POINT('Ctrl Pts',(-5.72993077912021,-85.7617511126202,
9.92453123332962));
#32409=CARTESIAN_POINT('Ctrl Pts',(1.7230702667452E-11,-85.5867511126203,
9.92453123331945));
#32410=CARTESIAN_POINT('Ctrl Pts',(5.72993077915523,-85.4117511126203,9.9245312333094));
#32411=CARTESIAN_POINT('Ctrl Pts',(8.59489616871553,-85.2367511126202,4.96226561664451));
#32412=CARTESIAN_POINT('Ctrl Pts',(11.4598615582757,-85.0617511126203,-1.9834529522248E-11));
#32413=CARTESIAN_POINT('Ctrl Pts',(8.59489616869807,-84.8867511126203,-4.96226561667475));
#32414=CARTESIAN_POINT('Ctrl Pts',(5.72993077912031,-84.7117511126203,-9.92453123332956));
#32415=CARTESIAN_POINT('Ctrl Pts',(-1.71237102093063E-11,-84.5367511126202,
-9.92453123331945));
#32416=CARTESIAN_POINT('Ctrl Pts',(-5.72993077915512,-84.3617511126203,
-9.92453123330946));
#32417=CARTESIAN_POINT('Ctrl Pts',(-8.59489616871548,-84.1867511126203,
-4.9622656166446));
#32418=CARTESIAN_POINT('Ctrl Pts',(-11.4598615582757,-84.0117511126203,
1.97109852732247E-11));
#32419=CARTESIAN_POINT('Ctrl Pts',(-8.59489616869813,-83.8367511126203,
4.96226561667465));
#32420=CARTESIAN_POINT('Ctrl Pts',(-5.72993077912042,-83.6617511126203,
9.9245312333295));
#32421=CARTESIAN_POINT('Ctrl Pts',(1.75808620370534E-11,-83.4867511126202,
9.92453123331945));
#32422=CARTESIAN_POINT('Ctrl Pts',(5.72993077915502,-83.3117511126203,9.92453123330952));
#32423=CARTESIAN_POINT('Ctrl Pts',(8.59489616871543,-83.1367511126203,4.96226561664469));
#32424=CARTESIAN_POINT('Ctrl Pts',(11.4598615582757,-82.9617511126202,-2.02388587348453E-11));
#32425=CARTESIAN_POINT('Ctrl Pts',(8.59489616869818,-82.7867511126203,-4.96226561667456));
#32426=CARTESIAN_POINT('Ctrl Pts',(5.72993077912053,-82.6117511126203,-9.92453123332944));
#32427=CARTESIAN_POINT('Ctrl Pts',(-1.74738695789077E-11,-82.4367511126202,
-9.92453123331945));
#32428=CARTESIAN_POINT('Ctrl Pts',(-5.72993077915491,-82.2617511126203,
-9.92453123330959));
#32429=CARTESIAN_POINT('Ctrl Pts',(-8.59489616871537,-82.0867511126203,
-4.96226561664478));
#32430=CARTESIAN_POINT('Ctrl Pts',(-11.4598615582757,-81.9117511126203,
2.01153144858219E-11));
#32431=CARTESIAN_POINT('Ctrl Pts',(-8.59489616869795,-81.7367511126203,
4.96226561667496));
#32432=CARTESIAN_POINT('Ctrl Pts',(-5.72993077912063,-81.5617511126202,
9.92453123332938));
#32433=CARTESIAN_POINT('Ctrl Pts',(1.7366877120762E-11,-81.3867511126203,
9.92453123331945));
#32434=CARTESIAN_POINT('Ctrl Pts',(5.72993077915537,-81.2117511126203,9.92453123330932));
#32435=CARTESIAN_POINT('Ctrl Pts',(8.59489616871532,-81.0367511126203,4.96226561664488));
#32436=CARTESIAN_POINT('Ctrl Pts',(11.4598615582757,-80.8617511126203,-1.99917702367986E-11));
#32437=CARTESIAN_POINT('Ctrl Pts',(8.59489616869801,-80.6867511126203,-4.96226561667487));
#32438=CARTESIAN_POINT('Ctrl Pts',(5.72993077912074,-80.5117511126203,-9.92453123332931));
#32439=CARTESIAN_POINT('Ctrl Pts',(-1.72598846626164E-11,-80.3367511126203,
-9.92453123331945));
#32440=CARTESIAN_POINT('Ctrl Pts',(-5.72993077915526,-80.1617511126203,
-9.92453123330938));
#32441=CARTESIAN_POINT('Ctrl Pts',(-8.59489616871555,-79.9867511126203,
-4.96226561664448));
#32442=CARTESIAN_POINT('Ctrl Pts',(-11.4598615582757,-79.8117511126203,
1.98682259877752E-11));
#32443=CARTESIAN_POINT('Ctrl Pts',(-8.59489616869806,-79.6367511126202,
4.96226561667477));
#32444=CARTESIAN_POINT('Ctrl Pts',(-5.72993077912029,-79.4617511126203,
9.92453123332958));
#32445=CARTESIAN_POINT('Ctrl Pts',(1.71528922044707E-11,-79.2867511126203,
9.92453123331945));
#32446=CARTESIAN_POINT('Ctrl Pts',(5.72993077915515,-79.1117511126203,9.92453123330944));
#32447=CARTESIAN_POINT('Ctrl Pts',(8.59489616871549,-78.9367511126203,4.96226561664457));
#32448=CARTESIAN_POINT('Ctrl Pts',(11.4598615582757,-78.7617511126203,-1.97446817387519E-11));
#32449=CARTESIAN_POINT('Ctrl Pts',(8.59489616869811,-78.5867511126203,-4.96226561667468));
#32450=CARTESIAN_POINT('Ctrl Pts',(5.72993077912039,-78.4117511126203,-9.92453123332952));
#32451=CARTESIAN_POINT('Ctrl Pts',(-1.76100440322177E-11,-78.2367511126203,
-9.92453123331945));
#32452=CARTESIAN_POINT('Ctrl Pts',(-5.72993077915505,-78.0617511126203,
-9.92453123330951));
#32453=CARTESIAN_POINT('Ctrl Pts',(-8.59489616871544,-77.8867511126203,
-4.96226561664467));
#32454=CARTESIAN_POINT('Ctrl Pts',(-11.4598615582757,-77.7117511126203,
2.02725552003725E-11));
#32455=CARTESIAN_POINT('Ctrl Pts',(-8.59489616869817,-77.5367511126203,
4.96226561667459));
#32456=CARTESIAN_POINT('Ctrl Pts',(-5.7299307791205,-77.3617511126203,9.92453123332946));
#32457=CARTESIAN_POINT('Ctrl Pts',(1.75030515740721E-11,-77.1867511126203,
9.92453123331945));
#32458=CARTESIAN_POINT('Ctrl Pts',(5.72993077915494,-77.0117511126203,9.92453123330957));
#32459=CARTESIAN_POINT('Ctrl Pts',(8.59489616871539,-76.8367511126203,4.96226561664476));
#32460=CARTESIAN_POINT('Ctrl Pts',(11.4598615582757,-76.6617511126203,-2.01490109513492E-11));
#32461=CARTESIAN_POINT('Ctrl Pts',(8.59489616869822,-76.4867511126203,-4.96226561667449));
#32462=CARTESIAN_POINT('Ctrl Pts',(5.72993077912061,-76.3117511126203,-9.92453123332939));
#32463=CARTESIAN_POINT('Ctrl Pts',(-1.73960591159264E-11,-76.1367511126203,
-9.92453123331945));
#32464=CARTESIAN_POINT('Ctrl Pts',(-5.7299307791554,-75.9617511126203,-9.92453123330931));
#32465=CARTESIAN_POINT('Ctrl Pts',(-8.59489616871534,-75.7867511126203,
-4.96226561664485));
#32466=CARTESIAN_POINT('Ctrl Pts',(-11.4598615582757,-75.6117511126203,
2.00254667023258E-11));
#32467=CARTESIAN_POINT('Ctrl Pts',(-8.59489616869799,-75.4367511126203,
4.96226561667489));
#32468=CARTESIAN_POINT('Ctrl Pts',(-5.72993077912071,-75.2617511126203,
9.92453123332933));
#32469=CARTESIAN_POINT('Ctrl Pts',(1.72890666577807E-11,-75.0867511126203,
9.92453123331945));
#32470=CARTESIAN_POINT('Ctrl Pts',(5.72993077915529,-74.9117511126203,9.92453123330937));
#32471=CARTESIAN_POINT('Ctrl Pts',(8.59489616871528,-74.7367511126203,4.96226561664494));
#32472=CARTESIAN_POINT('Ctrl Pts',(11.4598615582757,-74.5617511126203,-1.99019224533025E-11));
#32473=CARTESIAN_POINT('Ctrl Pts',(8.59489616869805,-74.3867511126203,-4.9622656166748));
#32474=CARTESIAN_POINT('Ctrl Pts',(5.72993077912025,-74.2117511126203,-9.9245312333296));
#32475=CARTESIAN_POINT('Ctrl Pts',(-1.7182074199635E-11,-74.0367511126203,
-9.92453123331945));
#32476=CARTESIAN_POINT('Ctrl Pts',(-5.72993077915518,-73.8617511126203,
-9.92453123330943));
#32477=CARTESIAN_POINT('Ctrl Pts',(-8.59489616871551,-73.6867511126203,
-4.96226561664455));
#32478=CARTESIAN_POINT('Ctrl Pts',(-11.4598615582757,-73.5117511126203,
1.97783782042791E-11));
#32479=CARTESIAN_POINT('Ctrl Pts',(-8.5948961686981,-73.3367511126203,4.9622656166747));
#32480=CARTESIAN_POINT('Ctrl Pts',(-5.72993077912036,-73.1617511126203,
9.92453123332954));
#32481=CARTESIAN_POINT('Ctrl Pts',(1.70750817414893E-11,-72.9867511126203,
9.92453123331945));
#32482=CARTESIAN_POINT('Ctrl Pts',(5.72993077915508,-72.8117511126203,9.92453123330949));
#32483=CARTESIAN_POINT('Ctrl Pts',(8.59489616871546,-72.6367511126203,4.96226561664464));
#32484=CARTESIAN_POINT('Ctrl Pts',(11.4598615582757,-72.4617511126203,-2.03062516658997E-11));
#32485=CARTESIAN_POINT('Ctrl Pts',(8.59489616869815,-72.2867511126203,-4.96226561667461));
#32486=CARTESIAN_POINT('Ctrl Pts',(5.72993077912047,-72.1117511126203,-9.92453123332947));
#32487=CARTESIAN_POINT('Ctrl Pts',(-1.75322335692364E-11,-71.9367511126203,
-9.92453123331945));
#32488=CARTESIAN_POINT('Ctrl Pts',(-5.72993077915497,-71.7617511126203,
-9.92453123330955));
#32489=CARTESIAN_POINT('Ctrl Pts',(-8.5948961687154,-71.5867511126203,-4.96226561664473));
#32490=CARTESIAN_POINT('Ctrl Pts',(-11.4598615582757,-71.4117511126203,
2.01827074168764E-11));
#32491=CARTESIAN_POINT('Ctrl Pts',(-8.59489616869821,-71.2367511126203,
4.96226561667452));
#32492=CARTESIAN_POINT('Ctrl Pts',(-5.72993077912058,-71.0617511126203,
9.92453123332941));
#32493=CARTESIAN_POINT('Ctrl Pts',(1.74252411110907E-11,-70.8867511126203,
9.92453123331945));
#32494=CARTESIAN_POINT('Ctrl Pts',(5.72993077915486,-70.7117511126203,9.92453123330961));
#32495=CARTESIAN_POINT('Ctrl Pts',(8.59489616871535,-70.5367511126203,4.96226561664483));
#32496=CARTESIAN_POINT('Ctrl Pts',(11.4598615582757,-70.3617511126203,-2.0059163167853E-11));
#32497=CARTESIAN_POINT('Ctrl Pts',(8.59489616869798,-70.1867511126203,-4.96226561667492));
#32498=CARTESIAN_POINT('Ctrl Pts',(5.72993077912068,-70.0117511126203,-9.92453123332935));
#32499=CARTESIAN_POINT('Ctrl Pts',(-1.7318248652945E-11,-69.8367511126203,
-9.92453123331945));
#32500=CARTESIAN_POINT('Ctrl Pts',(-5.72993077915532,-69.6617511126203,
-9.92453123330935));
#32501=CARTESIAN_POINT('Ctrl Pts',(-8.59489616871529,-69.4867511126203,
-4.96226561664492));
#32502=CARTESIAN_POINT('Ctrl Pts',(-11.4598615582757,-69.3117511126203,
1.99356189188297E-11));
#32503=CARTESIAN_POINT('Ctrl Pts',(-8.59489616869803,-69.1367511126203,
4.96226561667482));
#32504=CARTESIAN_POINT('Ctrl Pts',(-5.72993077912079,-68.9617511126203,
9.92453123332929));
#32505=CARTESIAN_POINT('Ctrl Pts',(1.72112561947994E-11,-68.7867511126203,
9.92453123331945));
#32506=CARTESIAN_POINT('Ctrl Pts',(5.72993077915521,-68.6117511126203,9.92453123330941));
#32507=CARTESIAN_POINT('Ctrl Pts',(8.59489616871553,-68.4367511126203,4.96226561664452));
#32508=CARTESIAN_POINT('Ctrl Pts',(11.4598615582757,-68.2617511126203,-1.98120746698064E-11));
#32509=CARTESIAN_POINT('Ctrl Pts',(8.59489616869808,-68.0867511126203,-4.96226561667473));
#32510=CARTESIAN_POINT('Ctrl Pts',(5.72993077912033,-67.9117511126203,-9.92453123332955));
#32511=CARTESIAN_POINT('Ctrl Pts',(-1.71042637366537E-11,-67.7367511126203,
-9.92453123331945));
#32512=CARTESIAN_POINT('Ctrl Pts',(-5.72993077915511,-67.5617511126203,
-9.92453123330947));
#32513=CARTESIAN_POINT('Ctrl Pts',(-8.59489616871547,-67.3867511126203,
-4.96226561664462));
#32514=CARTESIAN_POINT('Ctrl Pts',(-11.4598615582757,-67.2117511126203,
1.9688530420783E-11));
#32515=CARTESIAN_POINT('Ctrl Pts',(-8.59489616869814,-67.0367511126203,
4.96226561667464));
#32516=CARTESIAN_POINT('Ctrl Pts',(-5.72993077912044,-66.8617511126203,
9.92453123332949));
#32517=CARTESIAN_POINT('Ctrl Pts',(1.75614155644007E-11,-66.6867511126203,
9.92453123331945));
#32518=CARTESIAN_POINT('Ctrl Pts',(5.729930779155,-66.5117511126203,9.92453123330953));
#32519=CARTESIAN_POINT('Ctrl Pts',(8.59489616871542,-66.3367511126203,4.96226561664471));
#32520=CARTESIAN_POINT('Ctrl Pts',(11.4598615582757,-66.1617511126203,-2.02164038824036E-11));
#32521=CARTESIAN_POINT('Ctrl Pts',(8.59489616869819,-65.9867511126203,-4.96226561667455));
#32522=CARTESIAN_POINT('Ctrl Pts',(5.72993077912055,-65.8117511126203,-9.92453123332943));
#32523=CARTESIAN_POINT('Ctrl Pts',(-1.74544231062551E-11,-65.6367511126203,
-9.92453123331945));
#32524=CARTESIAN_POINT('Ctrl Pts',(-5.72993077915489,-65.4617511126203,
-9.9245312333096));
#32525=CARTESIAN_POINT('Ctrl Pts',(-8.59489616871537,-65.2867511126203,
-4.9622656166448));
#32526=CARTESIAN_POINT('Ctrl Pts',(-11.4598615582757,-65.1117511126203,
2.00928596333803E-11));
#32527=CARTESIAN_POINT('Ctrl Pts',(-8.59489616869824,-64.9367511126203,
4.96226561667445));
#32528=CARTESIAN_POINT('Ctrl Pts',(-5.72993077912065,-64.7617511126203,
9.92453123332936));
#32529=CARTESIAN_POINT('Ctrl Pts',(1.73474306481094E-11,-64.5867511126203,
9.92453123331945));
#32530=CARTESIAN_POINT('Ctrl Pts',(5.72993077915535,-64.4117511126203,9.92453123330933));
#32531=CARTESIAN_POINT('Ctrl Pts',(8.59489616871531,-64.2367511126203,4.96226561664489));
#32532=CARTESIAN_POINT('Ctrl Pts',(11.4598615582757,-64.0617511126203,-1.9969315384357E-11));
#32533=CARTESIAN_POINT('Ctrl Pts',(8.59489616869802,-63.8867511126203,-4.96226561667485));
#32534=CARTESIAN_POINT('Ctrl Pts',(5.72993077912076,-63.7117511126203,-9.9245312333293));
#32535=CARTESIAN_POINT('Ctrl Pts',(-1.72404381899637E-11,-63.5367511126203,
-9.92453123331945));
#32536=CARTESIAN_POINT('Ctrl Pts',(-5.72993077915524,-63.3617511126203,
-9.92453123330939));
#32537=CARTESIAN_POINT('Ctrl Pts',(-8.59489616871526,-63.1867511126203,
-4.96226561664499));
#32538=CARTESIAN_POINT('Ctrl Pts',(-11.4598615582757,-63.0117511126203,
1.98457711353336E-11));
#32539=CARTESIAN_POINT('Ctrl Pts',(-8.59489616869807,-62.8367511126203,
4.96226561667476));
#32540=CARTESIAN_POINT('Ctrl Pts',(-5.7299307791203,-62.6617511126203,9.92453123332957));
#32541=CARTESIAN_POINT('Ctrl Pts',(1.7133445731818E-11,-62.4867511126203,
9.92453123331945));
#32542=CARTESIAN_POINT('Ctrl Pts',(5.72993077915513,-62.3117511126203,9.92453123330946));
#32543=CARTESIAN_POINT('Ctrl Pts',(8.59489616871549,-62.1367511126203,4.96226561664459));
#32544=CARTESIAN_POINT('Ctrl Pts',(11.4598615582757,-61.9617511126203,-1.97222268863103E-11));
#32545=CARTESIAN_POINT('Ctrl Pts',(8.59489616869812,-61.7867511126203,-4.96226561667466));
#32546=CARTESIAN_POINT('Ctrl Pts',(5.72993077912041,-61.6117511126203,-9.92453123332951));
#32547=CARTESIAN_POINT('Ctrl Pts',(-1.70264532736723E-11,-61.4367511126203,
-9.92453123331945));
#32548=CARTESIAN_POINT('Ctrl Pts',(-5.72993077915503,-61.2617511126203,
-9.92453123330952));
#32549=CARTESIAN_POINT('Ctrl Pts',(-8.59489616871543,-61.0867511126203,
-4.96226561664468));
#32550=CARTESIAN_POINT('Ctrl Pts',(-11.4598615582757,-60.9117511126203,
2.02501003479309E-11));
#32551=CARTESIAN_POINT('Ctrl Pts',(-8.59489616869817,-60.7367511126203,
4.96226561667457));
#32552=CARTESIAN_POINT('Ctrl Pts',(-5.72993077912052,-60.5617511126203,
9.92453123332944));
#32553=CARTESIAN_POINT('Ctrl Pts',(1.74836051014194E-11,-60.3867511126203,
9.92453123331945));
#32554=CARTESIAN_POINT('Ctrl Pts',(5.72993077915492,-60.2117511126203,9.92453123330958));
#32555=CARTESIAN_POINT('Ctrl Pts',(8.59489616871538,-60.0367511126203,4.96226561664478));
#32556=CARTESIAN_POINT('Ctrl Pts',(11.4598615582757,-59.8617511126203,-2.01265560989075E-11));
#32557=CARTESIAN_POINT('Ctrl Pts',(8.59489616869823,-59.6867511126203,-4.96226561667448));
#32558=CARTESIAN_POINT('Ctrl Pts',(5.72993077912063,-59.5117511126203,-9.92453123332938));
#32559=CARTESIAN_POINT('Ctrl Pts',(-1.73766126432737E-11,-59.3367511126203,
-9.92453123331945));
#32560=CARTESIAN_POINT('Ctrl Pts',(-5.72993077915538,-59.1617511126203,
-9.92453123330931));
#32561=CARTESIAN_POINT('Ctrl Pts',(-8.59489616871532,-58.9867511126203,
-4.96226561664487));
#32562=CARTESIAN_POINT('Ctrl Pts',(-11.4598615582757,-58.8117511126203,
2.00030118498842E-11));
#32563=CARTESIAN_POINT('Ctrl Pts',(-8.594896168698,-58.6367511126203,4.96226561667487));
#32564=CARTESIAN_POINT('Ctrl Pts',(-5.72993077912073,-58.4617511126203,
9.92453123332932));
#32565=CARTESIAN_POINT('Ctrl Pts',(1.7269620185128E-11,-58.2867511126203,
9.92453123331945));
#32566=CARTESIAN_POINT('Ctrl Pts',(5.72993077915527,-58.1117511126203,9.92453123330938));
#32567=CARTESIAN_POINT('Ctrl Pts',(8.59489616871527,-57.9367511126203,4.96226561664496));
#32568=CARTESIAN_POINT('Ctrl Pts',(11.4598615582757,-57.7617511126203,-1.98794676008609E-11));
#32569=CARTESIAN_POINT('Ctrl Pts',(8.59489616869805,-57.5867511126203,-4.96226561667478));
#32570=CARTESIAN_POINT('Ctrl Pts',(5.72993077912084,-57.4117511126203,-9.92453123332926));
#32571=CARTESIAN_POINT('Ctrl Pts',(-1.71626277269823E-11,-57.2367511126203,
-9.92453123331945));
#32572=CARTESIAN_POINT('Ctrl Pts',(-5.72993077915516,-57.0617511126203,
-9.92453123330944));
#32573=CARTESIAN_POINT('Ctrl Pts',(-8.5948961687155,-56.8867511126203,-4.96226561664457));
#32574=CARTESIAN_POINT('Ctrl Pts',(-11.4598615582757,-56.7117511126203,
1.97559233518375E-11));
#32575=CARTESIAN_POINT('Ctrl Pts',(-8.59489616869811,-56.5367511126203,
4.96226561667469));
#32576=CARTESIAN_POINT('Ctrl Pts',(-5.72993077912038,-56.3617511126203,
9.92453123332952));
#32577=CARTESIAN_POINT('Ctrl Pts',(1.70556352688367E-11,-56.1867511126203,
9.92453123331945));
#32578=CARTESIAN_POINT('Ctrl Pts',(5.72993077915506,-56.0117511126203,9.9245312333095));
#32579=CARTESIAN_POINT('Ctrl Pts',(8.59489616871545,-55.8367511126203,4.96226561664466));
#32580=CARTESIAN_POINT('Ctrl Pts',(11.4598615582757,-55.6617511126203,-1.96323791028142E-11));
#32581=CARTESIAN_POINT('Ctrl Pts',(8.59489616869816,-55.4867511126203,-4.96226561667459));
#32582=CARTESIAN_POINT('Ctrl Pts',(5.72993077912049,-55.3117511126203,-9.92453123332946));
#32583=CARTESIAN_POINT('Ctrl Pts',(-1.75127870965837E-11,-55.1367511126203,
-9.92453123331945));
#32584=CARTESIAN_POINT('Ctrl Pts',(-5.72993077915495,-54.9617511126203,
-9.92453123330957));
#32585=CARTESIAN_POINT('Ctrl Pts',(-8.59489616871539,-54.7867511126203,
-4.96226561664475));
#32586=CARTESIAN_POINT('Ctrl Pts',(-11.4598615582757,-54.6117511126203,
2.01602525644348E-11));
#32587=CARTESIAN_POINT('Ctrl Pts',(-8.59489616869821,-54.4367511126203,
4.9622656166745));
#32588=CARTESIAN_POINT('Ctrl Pts',(-5.7299307791206,-54.2617511126203,9.9245312333294));
#32589=CARTESIAN_POINT('Ctrl Pts',(1.7405794638438E-11,-54.0867511126203,
9.92453123331945));
#32590=CARTESIAN_POINT('Ctrl Pts',(5.72993077915484,-53.9117511126203,9.92453123330963));
#32591=CARTESIAN_POINT('Ctrl Pts',(8.59489616871534,-53.7367511126203,4.96226561664484));
#32592=CARTESIAN_POINT('Ctrl Pts',(11.4598615582757,-53.5617511126203,-2.00367083154114E-11));
#32593=CARTESIAN_POINT('Ctrl Pts',(8.59489616869799,-53.3867511126203,-4.9622656166749));
#32594=CARTESIAN_POINT('Ctrl Pts',(5.7299307791207,-53.2117511126203,-9.92453123332934));
#32595=CARTESIAN_POINT('Ctrl Pts',(-1.72988021802924E-11,-53.0367511126203,
-9.92453123331945));
#32596=CARTESIAN_POINT('Ctrl Pts',(-5.7299307791553,-52.8617511126203,-9.92453123330936));
#32597=CARTESIAN_POINT('Ctrl Pts',(-8.59489616871529,-52.6867511126203,
-4.96226561664494));
#32598=CARTESIAN_POINT('Ctrl Pts',(-11.4598615582757,-52.5117511126203,
1.99131640663881E-11));
#32599=CARTESIAN_POINT('Ctrl Pts',(-8.59489616869804,-52.3367511126203,
4.96226561667481));
#32600=CARTESIAN_POINT('Ctrl Pts',(-5.72993077912081,-52.1617511126203,
9.92453123332928));
#32601=CARTESIAN_POINT('Ctrl Pts',(1.71918097221467E-11,-51.9867511126203,
9.92453123331945));
#32602=CARTESIAN_POINT('Ctrl Pts',(5.72993077915519,-51.8117511126203,9.92453123330942));
#32603=CARTESIAN_POINT('Ctrl Pts',(8.59489616871523,-51.6367511126203,4.96226561664503));
#32604=CARTESIAN_POINT('Ctrl Pts',(11.4598615582757,-51.4617511126203,-1.97896198173647E-11));
#32605=CARTESIAN_POINT('Ctrl Pts',(8.59489616869809,-51.2867511126203,-4.96226561667471));
#32606=CARTESIAN_POINT('Ctrl Pts',(5.72993077912035,-51.1117511126203,-9.92453123332954));
#32607=CARTESIAN_POINT('Ctrl Pts',(-1.7084817264001E-11,-50.9367511126203,
-9.92453123331945));
#32608=CARTESIAN_POINT('Ctrl Pts',(-5.72993077915509,-50.7617511126203,
-9.92453123330948));
#32609=CARTESIAN_POINT('Ctrl Pts',(-8.59489616871546,-50.5867511126203,
-4.96226561664463));
#32610=CARTESIAN_POINT('Ctrl Pts',(-11.4598615582757,-50.4117511126204,
1.96660755683414E-11));
#32611=CARTESIAN_POINT('Ctrl Pts',(-8.59489616869815,-50.2367511126203,
4.96226561667462));
#32612=CARTESIAN_POINT('Ctrl Pts',(-5.72993077912046,-50.0617511126203,
9.92453123332948));
#32613=CARTESIAN_POINT('Ctrl Pts',(1.69778248058553E-11,-49.8867511126203,
9.92453123331945));
#32614=CARTESIAN_POINT('Ctrl Pts',(5.72993077915498,-49.7117511126203,9.92453123330955));
#32615=CARTESIAN_POINT('Ctrl Pts',(8.59489616871541,-49.5367511126204,4.96226561664473));
#32616=CARTESIAN_POINT('Ctrl Pts',(11.4598615582757,-49.3617511126203,-2.0193949029962E-11));
#32617=CARTESIAN_POINT('Ctrl Pts',(8.5948961686982,-49.1867511126203,-4.96226561667453));
#32618=CARTESIAN_POINT('Ctrl Pts',(5.72993077912057,-49.0117511126203,-9.92453123332941));
#32619=CARTESIAN_POINT('Ctrl Pts',(-1.74349766336024E-11,-48.8367511126203,
-9.92453123331945));
#32620=CARTESIAN_POINT('Ctrl Pts',(-5.72993077915487,-48.6617511126203,
-9.92453123330961));
#32621=CARTESIAN_POINT('Ctrl Pts',(-8.59489616871535,-48.4867511126203,
-4.96226561664482));
#32622=CARTESIAN_POINT('Ctrl Pts',(-11.4598615582757,-48.3117511126203,
2.00704047809387E-11));
#32623=CARTESIAN_POINT('Ctrl Pts',(-8.59489616869825,-48.1367511126203,
4.96226561667444));
#32624=CARTESIAN_POINT('Ctrl Pts',(-5.72993077912067,-47.9617511126203,
9.92453123332935));
#32625=CARTESIAN_POINT('Ctrl Pts',(1.73279841754567E-11,-47.7867511126204,
9.92453123331945));
#32626=CARTESIAN_POINT('Ctrl Pts',(2.38370069761474,-47.7139496010212,9.92453123331524));
#32627=CARTESIAN_POINT('Ctrl Pts',(4.50738083181344,-47.63,8.84193633985987));
#32628=CARTESIAN_POINT('Ctrl Pts',(-1.51301075899711E-11,-213.943984254242,
-8.40164026751963));
#32629=CARTESIAN_POINT('Ctrl Pts',(-4.85068927010199,-213.768984254242,
-8.4016402675109));
#32630=CARTESIAN_POINT('Ctrl Pts',(-7.27603390513785,-213.593984254242,
-4.20082013374671));
#32631=CARTESIAN_POINT('Ctrl Pts',(-9.70137854017372,-213.418984254242,
1.74701493417668E-11));
#32632=CARTESIAN_POINT('Ctrl Pts',(-7.27603390512272,-213.243984254242,
4.20082013377292));
#32633=CARTESIAN_POINT('Ctrl Pts',(-4.85068927007173,-213.068984254242,
8.40164026752836));
#32634=CARTESIAN_POINT('Ctrl Pts',(1.5129078685785E-11,-212.893984254242,
8.40164026751963));
#32635=CARTESIAN_POINT('Ctrl Pts',(4.85068927010198,-212.718984254242,8.4016402675109));
#32636=CARTESIAN_POINT('Ctrl Pts',(7.27603390513785,-212.543984254242,4.20082013374672));
#32637=CARTESIAN_POINT('Ctrl Pts',(9.70137854017372,-212.368984254242,-1.74689612655491E-11));
#32638=CARTESIAN_POINT('Ctrl Pts',(7.27603390512273,-212.193984254242,-4.20082013377291));
#32639=CARTESIAN_POINT('Ctrl Pts',(4.85068927007173,-212.018984254242,-8.40164026752836));
#32640=CARTESIAN_POINT('Ctrl Pts',(-1.51301075899711E-11,-211.843984254242,
-8.40164026751963));
#32641=CARTESIAN_POINT('Ctrl Pts',(-4.85068927010199,-211.668984254242,
-8.4016402675109));
#32642=CARTESIAN_POINT('Ctrl Pts',(-7.27603390513785,-211.493984254242,
-4.20082013374671));
#32643=CARTESIAN_POINT('Ctrl Pts',(-9.70137854017372,-211.318984254242,
1.74701493417668E-11));
#32644=CARTESIAN_POINT('Ctrl Pts',(-7.27603390512272,-211.143984254242,
4.20082013377292));
#32645=CARTESIAN_POINT('Ctrl Pts',(-4.85068927007173,-210.968984254242,
8.40164026752836));
#32646=CARTESIAN_POINT('Ctrl Pts',(1.5129078685785E-11,-210.793984254242,
8.40164026751963));
#32647=CARTESIAN_POINT('Ctrl Pts',(4.85068927010198,-210.618984254242,8.4016402675109));
#32648=CARTESIAN_POINT('Ctrl Pts',(7.27603390513785,-210.443984254242,4.20082013374672));
#32649=CARTESIAN_POINT('Ctrl Pts',(9.70137854017372,-210.268984254242,-1.74689612655491E-11));
#32650=CARTESIAN_POINT('Ctrl Pts',(7.27603390512273,-210.093984254242,-4.20082013377291));
#32651=CARTESIAN_POINT('Ctrl Pts',(4.85068927007173,-209.918984254242,-8.40164026752836));
#32652=CARTESIAN_POINT('Ctrl Pts',(-1.51301075899711E-11,-209.743984254242,
-8.40164026751963));
#32653=CARTESIAN_POINT('Ctrl Pts',(-4.85068927010199,-209.568984254242,
-8.4016402675109));
#32654=CARTESIAN_POINT('Ctrl Pts',(-7.27603390513785,-209.393984254242,
-4.20082013374671));
#32655=CARTESIAN_POINT('Ctrl Pts',(-9.70137854017372,-209.218984254242,
1.74701493417668E-11));
#32656=CARTESIAN_POINT('Ctrl Pts',(-7.27603390512272,-209.043984254242,
4.20082013377292));
#32657=CARTESIAN_POINT('Ctrl Pts',(-4.85068927007173,-208.868984254242,
8.40164026752836));
#32658=CARTESIAN_POINT('Ctrl Pts',(1.5129078685785E-11,-208.693984254242,
8.40164026751963));
#32659=CARTESIAN_POINT('Ctrl Pts',(4.85068927010198,-208.518984254242,8.4016402675109));
#32660=CARTESIAN_POINT('Ctrl Pts',(7.27603390513785,-208.343984254242,4.20082013374672));
#32661=CARTESIAN_POINT('Ctrl Pts',(9.70137854017372,-208.168984254242,-1.74689612655491E-11));
#32662=CARTESIAN_POINT('Ctrl Pts',(7.27603390512273,-207.993984254242,-4.20082013377291));
#32663=CARTESIAN_POINT('Ctrl Pts',(4.85068927007173,-207.818984254242,-8.40164026752836));
#32664=CARTESIAN_POINT('Ctrl Pts',(-1.51301075899711E-11,-207.643984254242,
-8.40164026751963));
#32665=CARTESIAN_POINT('Ctrl Pts',(-4.85068927010199,-207.468984254242,
-8.4016402675109));
#32666=CARTESIAN_POINT('Ctrl Pts',(-7.27603390513785,-207.293984254242,
-4.20082013374671));
#32667=CARTESIAN_POINT('Ctrl Pts',(-9.70137854017372,-207.118984254242,
1.74701493417668E-11));
#32668=CARTESIAN_POINT('Ctrl Pts',(-7.27603390512272,-206.943984254242,
4.20082013377292));
#32669=CARTESIAN_POINT('Ctrl Pts',(-4.85068927007173,-206.768984254242,
8.40164026752836));
#32670=CARTESIAN_POINT('Ctrl Pts',(1.5129078685785E-11,-206.593984254242,
8.40164026751963));
#32671=CARTESIAN_POINT('Ctrl Pts',(4.85068927010198,-206.418984254242,8.4016402675109));
#32672=CARTESIAN_POINT('Ctrl Pts',(7.27603390513785,-206.243984254242,4.20082013374672));
#32673=CARTESIAN_POINT('Ctrl Pts',(9.70137854017372,-206.068984254242,-1.74689612655491E-11));
#32674=CARTESIAN_POINT('Ctrl Pts',(7.27603390512273,-205.893984254242,-4.20082013377291));
#32675=CARTESIAN_POINT('Ctrl Pts',(4.85068927007173,-205.718984254242,-8.40164026752836));
#32676=CARTESIAN_POINT('Ctrl Pts',(-1.51301075899711E-11,-205.543984254242,
-8.40164026751963));
#32677=CARTESIAN_POINT('Ctrl Pts',(-4.85068927010199,-205.368984254242,
-8.4016402675109));
#32678=CARTESIAN_POINT('Ctrl Pts',(-7.27603390513785,-205.193984254242,
-4.20082013374671));
#32679=CARTESIAN_POINT('Ctrl Pts',(-9.70137854017372,-205.018984254242,
1.74701493417668E-11));
#32680=CARTESIAN_POINT('Ctrl Pts',(-7.27603390512272,-204.843984254242,
4.20082013377292));
#32681=CARTESIAN_POINT('Ctrl Pts',(-4.85068927007173,-204.668984254242,
8.40164026752836));
#32682=CARTESIAN_POINT('Ctrl Pts',(1.5129078685785E-11,-204.493984254242,
8.40164026751963));
#32683=CARTESIAN_POINT('Ctrl Pts',(4.85068927010198,-204.318984254242,8.4016402675109));
#32684=CARTESIAN_POINT('Ctrl Pts',(7.27603390513785,-204.143984254242,4.20082013374672));
#32685=CARTESIAN_POINT('Ctrl Pts',(9.70137854017372,-203.968984254242,-1.74689612655491E-11));
#32686=CARTESIAN_POINT('Ctrl Pts',(7.27603390512273,-203.793984254242,-4.20082013377291));
#32687=CARTESIAN_POINT('Ctrl Pts',(4.85068927007173,-203.618984254242,-8.40164026752836));
#32688=CARTESIAN_POINT('Ctrl Pts',(-1.51301075899711E-11,-203.443984254242,
-8.40164026751963));
#32689=CARTESIAN_POINT('Ctrl Pts',(-4.85068927010199,-203.268984254242,
-8.4016402675109));
#32690=CARTESIAN_POINT('Ctrl Pts',(-7.27603390513785,-203.093984254242,
-4.20082013374671));
#32691=CARTESIAN_POINT('Ctrl Pts',(-9.70137854017372,-202.918984254242,
1.74701493417668E-11));
#32692=CARTESIAN_POINT('Ctrl Pts',(-7.27603390512272,-202.743984254242,
4.20082013377292));
#32693=CARTESIAN_POINT('Ctrl Pts',(-4.85068927007173,-202.568984254242,
8.40164026752836));
#32694=CARTESIAN_POINT('Ctrl Pts',(1.5129078685785E-11,-202.393984254242,
8.40164026751963));
#32695=CARTESIAN_POINT('Ctrl Pts',(4.85068927010198,-202.218984254242,8.4016402675109));
#32696=CARTESIAN_POINT('Ctrl Pts',(7.27603390513785,-202.043984254242,4.20082013374672));
#32697=CARTESIAN_POINT('Ctrl Pts',(9.70137854017372,-201.868984254242,-1.74689612655491E-11));
#32698=CARTESIAN_POINT('Ctrl Pts',(7.27603390512273,-201.693984254242,-4.20082013377291));
#32699=CARTESIAN_POINT('Ctrl Pts',(4.85068927007173,-201.518984254242,-8.40164026752836));
#32700=CARTESIAN_POINT('Ctrl Pts',(-1.51301075899711E-11,-201.343984254242,
-8.40164026751963));
#32701=CARTESIAN_POINT('Ctrl Pts',(-4.85068927010199,-201.168984254242,
-8.4016402675109));
#32702=CARTESIAN_POINT('Ctrl Pts',(-7.27603390513785,-200.993984254242,
-4.20082013374671));
#32703=CARTESIAN_POINT('Ctrl Pts',(-9.70137854017372,-200.818984254242,
1.74701493417668E-11));
#32704=CARTESIAN_POINT('Ctrl Pts',(-7.27603390512272,-200.643984254242,
4.20082013377292));
#32705=CARTESIAN_POINT('Ctrl Pts',(-4.85068927007173,-200.468984254242,
8.40164026752836));
#32706=CARTESIAN_POINT('Ctrl Pts',(1.5129078685785E-11,-200.293984254242,
8.40164026751963));
#32707=CARTESIAN_POINT('Ctrl Pts',(4.85068927010198,-200.118984254242,8.4016402675109));
#32708=CARTESIAN_POINT('Ctrl Pts',(7.27603390513785,-199.943984254242,4.20082013374672));
#32709=CARTESIAN_POINT('Ctrl Pts',(9.70137854017372,-199.768984254242,-1.74689612655491E-11));
#32710=CARTESIAN_POINT('Ctrl Pts',(7.27603390512273,-199.593984254242,-4.20082013377291));
#32711=CARTESIAN_POINT('Ctrl Pts',(4.85068927007173,-199.418984254242,-8.40164026752836));
#32712=CARTESIAN_POINT('Ctrl Pts',(-1.51301075899711E-11,-199.243984254242,
-8.40164026751963));
#32713=CARTESIAN_POINT('Ctrl Pts',(-4.85068927010199,-199.068984254242,
-8.4016402675109));
#32714=CARTESIAN_POINT('Ctrl Pts',(-7.27603390513785,-198.893984254242,
-4.20082013374671));
#32715=CARTESIAN_POINT('Ctrl Pts',(-9.70137854017372,-198.718984254242,
1.74701493417668E-11));
#32716=CARTESIAN_POINT('Ctrl Pts',(-7.27603390512272,-198.543984254242,
4.20082013377292));
#32717=CARTESIAN_POINT('Ctrl Pts',(-4.85068927007173,-198.368984254242,
8.40164026752836));
#32718=CARTESIAN_POINT('Ctrl Pts',(1.5129078685785E-11,-198.193984254242,
8.40164026751963));
#32719=CARTESIAN_POINT('Ctrl Pts',(4.85068927010198,-198.018984254242,8.4016402675109));
#32720=CARTESIAN_POINT('Ctrl Pts',(7.27603390513785,-197.843984254242,4.20082013374672));
#32721=CARTESIAN_POINT('Ctrl Pts',(9.70137854017372,-197.668984254242,-1.74689612655491E-11));
#32722=CARTESIAN_POINT('Ctrl Pts',(7.27603390512273,-197.493984254242,-4.20082013377291));
#32723=CARTESIAN_POINT('Ctrl Pts',(4.85068927007173,-197.318984254242,-8.40164026752836));
#32724=CARTESIAN_POINT('Ctrl Pts',(-1.51301075899711E-11,-197.143984254242,
-8.40164026751963));
#32725=CARTESIAN_POINT('Ctrl Pts',(-4.85068927010199,-196.968984254242,
-8.4016402675109));
#32726=CARTESIAN_POINT('Ctrl Pts',(-7.27603390513785,-196.793984254242,
-4.20082013374671));
#32727=CARTESIAN_POINT('Ctrl Pts',(-9.70137854017372,-196.618984254242,
1.74701493417668E-11));
#32728=CARTESIAN_POINT('Ctrl Pts',(-7.27603390512272,-196.443984254242,
4.20082013377292));
#32729=CARTESIAN_POINT('Ctrl Pts',(-4.85068927007173,-196.268984254242,
8.40164026752836));
#32730=CARTESIAN_POINT('Ctrl Pts',(1.5129078685785E-11,-196.093984254242,
8.40164026751963));
#32731=CARTESIAN_POINT('Ctrl Pts',(4.85068927010198,-195.918984254242,8.4016402675109));
#32732=CARTESIAN_POINT('Ctrl Pts',(7.27603390513785,-195.743984254242,4.20082013374672));
#32733=CARTESIAN_POINT('Ctrl Pts',(9.70137854017372,-195.568984254242,-1.74689612655491E-11));
#32734=CARTESIAN_POINT('Ctrl Pts',(7.27603390512273,-195.393984254242,-4.20082013377291));
#32735=CARTESIAN_POINT('Ctrl Pts',(4.85068927007173,-195.218984254242,-8.40164026752836));
#32736=CARTESIAN_POINT('Ctrl Pts',(-1.51301075899711E-11,-195.043984254242,
-8.40164026751963));
#32737=CARTESIAN_POINT('Ctrl Pts',(-4.85068927010199,-194.868984254242,
-8.4016402675109));
#32738=CARTESIAN_POINT('Ctrl Pts',(-7.27603390513785,-194.693984254242,
-4.20082013374671));
#32739=CARTESIAN_POINT('Ctrl Pts',(-9.70137854017372,-194.518984254242,
1.74701493417668E-11));
#32740=CARTESIAN_POINT('Ctrl Pts',(-7.27603390512272,-194.343984254242,
4.20082013377292));
#32741=CARTESIAN_POINT('Ctrl Pts',(-4.85068927007173,-194.168984254242,
8.40164026752836));
#32742=CARTESIAN_POINT('Ctrl Pts',(1.5129078685785E-11,-193.993984254242,
8.40164026751963));
#32743=CARTESIAN_POINT('Ctrl Pts',(4.85068927010198,-193.818984254242,8.4016402675109));
#32744=CARTESIAN_POINT('Ctrl Pts',(7.27603390513785,-193.643984254242,4.20082013374672));
#32745=CARTESIAN_POINT('Ctrl Pts',(9.70137854017372,-193.468984254242,-1.74689612655491E-11));
#32746=CARTESIAN_POINT('Ctrl Pts',(7.27603390512273,-193.293984254242,-4.20082013377291));
#32747=CARTESIAN_POINT('Ctrl Pts',(4.85068927007173,-193.118984254242,-8.40164026752836));
#32748=CARTESIAN_POINT('Ctrl Pts',(-1.51301075899711E-11,-192.943984254242,
-8.40164026751963));
#32749=CARTESIAN_POINT('Ctrl Pts',(-4.85068927010199,-192.768984254242,
-8.4016402675109));
#32750=CARTESIAN_POINT('Ctrl Pts',(-7.27603390513785,-192.593984254242,
-4.20082013374671));
#32751=CARTESIAN_POINT('Ctrl Pts',(-9.70137854017372,-192.418984254242,
1.74701493417668E-11));
#32752=CARTESIAN_POINT('Ctrl Pts',(-7.27603390512272,-192.243984254242,
4.20082013377292));
#32753=CARTESIAN_POINT('Ctrl Pts',(-4.85068927007173,-192.068984254242,
8.40164026752836));
#32754=CARTESIAN_POINT('Ctrl Pts',(1.5129078685785E-11,-191.893984254242,
8.40164026751963));
#32755=CARTESIAN_POINT('Ctrl Pts',(4.85068927010198,-191.718984254242,8.4016402675109));
#32756=CARTESIAN_POINT('Ctrl Pts',(7.27603390513785,-191.543984254242,4.20082013374672));
#32757=CARTESIAN_POINT('Ctrl Pts',(9.70137854017372,-191.368984254242,-1.74689612655491E-11));
#32758=CARTESIAN_POINT('Ctrl Pts',(7.27603390512273,-191.193984254242,-4.20082013377291));
#32759=CARTESIAN_POINT('Ctrl Pts',(4.85068927007173,-191.018984254242,-8.40164026752836));
#32760=CARTESIAN_POINT('Ctrl Pts',(-1.51301075899711E-11,-190.843984254242,
-8.40164026751963));
#32761=CARTESIAN_POINT('Ctrl Pts',(-4.85068927010199,-190.668984254242,
-8.4016402675109));
#32762=CARTESIAN_POINT('Ctrl Pts',(-7.27603390513785,-190.493984254242,
-4.20082013374671));
#32763=CARTESIAN_POINT('Ctrl Pts',(-9.70137854017372,-190.318984254242,
1.74701493417668E-11));
#32764=CARTESIAN_POINT('Ctrl Pts',(-7.27603390512272,-190.143984254242,
4.20082013377292));
#32765=CARTESIAN_POINT('Ctrl Pts',(-4.85068927007173,-189.968984254242,
8.40164026752836));
#32766=CARTESIAN_POINT('Ctrl Pts',(1.5129078685785E-11,-189.793984254242,
8.40164026751963));
#32767=CARTESIAN_POINT('Ctrl Pts',(4.85068927010198,-189.618984254242,8.4016402675109));
#32768=CARTESIAN_POINT('Ctrl Pts',(7.27603390513785,-189.443984254242,4.20082013374672));
#32769=CARTESIAN_POINT('Ctrl Pts',(9.70137854017372,-189.268984254242,-1.74689612655491E-11));
#32770=CARTESIAN_POINT('Ctrl Pts',(7.27603390512273,-189.093984254242,-4.20082013377291));
#32771=CARTESIAN_POINT('Ctrl Pts',(4.85068927007173,-188.918984254242,-8.40164026752836));
#32772=CARTESIAN_POINT('Ctrl Pts',(-1.51301075899711E-11,-188.743984254242,
-8.40164026751963));
#32773=CARTESIAN_POINT('Ctrl Pts',(-4.85068927010199,-188.568984254242,
-8.4016402675109));
#32774=CARTESIAN_POINT('Ctrl Pts',(-7.27603390513785,-188.393984254242,
-4.20082013374671));
#32775=CARTESIAN_POINT('Ctrl Pts',(-9.70137854017372,-188.218984254242,
1.74701493417668E-11));
#32776=CARTESIAN_POINT('Ctrl Pts',(-7.27603390512272,-188.043984254242,
4.20082013377292));
#32777=CARTESIAN_POINT('Ctrl Pts',(-4.85068927007173,-187.868984254242,
8.40164026752836));
#32778=CARTESIAN_POINT('Ctrl Pts',(1.5129078685785E-11,-187.693984254242,
8.40164026751963));
#32779=CARTESIAN_POINT('Ctrl Pts',(4.85068927010198,-187.518984254242,8.4016402675109));
#32780=CARTESIAN_POINT('Ctrl Pts',(7.27603390513785,-187.343984254242,4.20082013374672));
#32781=CARTESIAN_POINT('Ctrl Pts',(9.70137854017372,-187.168984254242,-1.74689612655491E-11));
#32782=CARTESIAN_POINT('Ctrl Pts',(7.27603390512273,-186.993984254242,-4.20082013377291));
#32783=CARTESIAN_POINT('Ctrl Pts',(4.85068927007173,-186.818984254242,-8.40164026752836));
#32784=CARTESIAN_POINT('Ctrl Pts',(-1.51301075899711E-11,-186.643984254242,
-8.40164026751963));
#32785=CARTESIAN_POINT('Ctrl Pts',(-4.85068927010199,-186.468984254242,
-8.4016402675109));
#32786=CARTESIAN_POINT('Ctrl Pts',(-7.27603390513785,-186.293984254242,
-4.20082013374671));
#32787=CARTESIAN_POINT('Ctrl Pts',(-9.70137854017372,-186.118984254242,
1.74701493417668E-11));
#32788=CARTESIAN_POINT('Ctrl Pts',(-7.27603390512272,-185.943984254242,
4.20082013377292));
#32789=CARTESIAN_POINT('Ctrl Pts',(-4.85068927007173,-185.768984254242,
8.40164026752836));
#32790=CARTESIAN_POINT('Ctrl Pts',(1.5129078685785E-11,-185.593984254242,
8.40164026751963));
#32791=CARTESIAN_POINT('Ctrl Pts',(4.85068927010198,-185.418984254242,8.4016402675109));
#32792=CARTESIAN_POINT('Ctrl Pts',(7.27603390513785,-185.243984254242,4.20082013374672));
#32793=CARTESIAN_POINT('Ctrl Pts',(9.70137854017372,-185.068984254242,-1.74689612655491E-11));
#32794=CARTESIAN_POINT('Ctrl Pts',(7.27603390512273,-184.893984254242,-4.20082013377291));
#32795=CARTESIAN_POINT('Ctrl Pts',(4.85068927007173,-184.718984254242,-8.40164026752836));
#32796=CARTESIAN_POINT('Ctrl Pts',(-1.51301075899711E-11,-184.543984254242,
-8.40164026751963));
#32797=CARTESIAN_POINT('Ctrl Pts',(-4.85068927010199,-184.368984254242,
-8.4016402675109));
#32798=CARTESIAN_POINT('Ctrl Pts',(-7.27603390513785,-184.193984254242,
-4.20082013374671));
#32799=CARTESIAN_POINT('Ctrl Pts',(-9.70137854017372,-184.018984254242,
1.74701493417668E-11));
#32800=CARTESIAN_POINT('Ctrl Pts',(-7.27603390512272,-183.843984254242,
4.20082013377292));
#32801=CARTESIAN_POINT('Ctrl Pts',(-4.85068927007173,-183.668984254242,
8.40164026752836));
#32802=CARTESIAN_POINT('Ctrl Pts',(1.5129078685785E-11,-183.493984254242,
8.40164026751963));
#32803=CARTESIAN_POINT('Ctrl Pts',(4.85068927010198,-183.318984254242,8.4016402675109));
#32804=CARTESIAN_POINT('Ctrl Pts',(7.27603390513785,-183.143984254242,4.20082013374672));
#32805=CARTESIAN_POINT('Ctrl Pts',(9.70137854017372,-182.968984254242,-1.74689612655491E-11));
#32806=CARTESIAN_POINT('Ctrl Pts',(7.27603390512273,-182.793984254242,-4.20082013377291));
#32807=CARTESIAN_POINT('Ctrl Pts',(4.85068927007173,-182.618984254242,-8.40164026752836));
#32808=CARTESIAN_POINT('Ctrl Pts',(-1.51301075899711E-11,-182.443984254242,
-8.40164026751963));
#32809=CARTESIAN_POINT('Ctrl Pts',(-4.85068927010199,-182.268984254242,
-8.4016402675109));
#32810=CARTESIAN_POINT('Ctrl Pts',(-7.27603390513785,-182.093984254242,
-4.20082013374671));
#32811=CARTESIAN_POINT('Ctrl Pts',(-9.70137854017372,-181.918984254242,
1.74701493417668E-11));
#32812=CARTESIAN_POINT('Ctrl Pts',(-7.27603390512272,-181.743984254242,
4.20082013377292));
#32813=CARTESIAN_POINT('Ctrl Pts',(-4.85068927007173,-181.568984254242,
8.40164026752836));
#32814=CARTESIAN_POINT('Ctrl Pts',(1.5129078685785E-11,-181.393984254242,
8.40164026751963));
#32815=CARTESIAN_POINT('Ctrl Pts',(4.85068927010198,-181.218984254242,8.4016402675109));
#32816=CARTESIAN_POINT('Ctrl Pts',(7.27603390513785,-181.043984254242,4.20082013374672));
#32817=CARTESIAN_POINT('Ctrl Pts',(9.70137854017372,-180.868984254242,-1.74689612655491E-11));
#32818=CARTESIAN_POINT('Ctrl Pts',(7.27603390512273,-180.693984254242,-4.20082013377291));
#32819=CARTESIAN_POINT('Ctrl Pts',(4.85068927007173,-180.518984254242,-8.40164026752836));
#32820=CARTESIAN_POINT('Ctrl Pts',(-1.51301075899711E-11,-180.343984254242,
-8.40164026751963));
#32821=CARTESIAN_POINT('Ctrl Pts',(-4.85068927010199,-180.168984254242,
-8.4016402675109));
#32822=CARTESIAN_POINT('Ctrl Pts',(-7.27603390513785,-179.993984254242,
-4.20082013374671));
#32823=CARTESIAN_POINT('Ctrl Pts',(-9.70137854017372,-179.818984254242,
1.74701493417668E-11));
#32824=CARTESIAN_POINT('Ctrl Pts',(-7.27603390512272,-179.643984254242,
4.20082013377292));
#32825=CARTESIAN_POINT('Ctrl Pts',(-4.85068927007173,-179.468984254242,
8.40164026752836));
#32826=CARTESIAN_POINT('Ctrl Pts',(1.5129078685785E-11,-179.293984254242,
8.40164026751963));
#32827=CARTESIAN_POINT('Ctrl Pts',(4.85068927010198,-179.118984254242,8.4016402675109));
#32828=CARTESIAN_POINT('Ctrl Pts',(7.27603390513785,-178.943984254242,4.20082013374672));
#32829=CARTESIAN_POINT('Ctrl Pts',(9.70137854017372,-178.768984254242,-1.74689612655491E-11));
#32830=CARTESIAN_POINT('Ctrl Pts',(7.27603390512273,-178.593984254242,-4.20082013377291));
#32831=CARTESIAN_POINT('Ctrl Pts',(4.85068927007173,-178.418984254242,-8.40164026752836));
#32832=CARTESIAN_POINT('Ctrl Pts',(-1.51301075899711E-11,-178.243984254242,
-8.40164026751963));
#32833=CARTESIAN_POINT('Ctrl Pts',(-4.85068927010199,-178.068984254242,
-8.4016402675109));
#32834=CARTESIAN_POINT('Ctrl Pts',(-7.27603390513785,-177.893984254242,
-4.20082013374671));
#32835=CARTESIAN_POINT('Ctrl Pts',(-9.70137854017372,-177.718984254242,
1.74701493417668E-11));
#32836=CARTESIAN_POINT('Ctrl Pts',(-7.27603390512272,-177.543984254242,
4.20082013377292));
#32837=CARTESIAN_POINT('Ctrl Pts',(-4.85068927007173,-177.368984254242,
8.40164026752836));
#32838=CARTESIAN_POINT('Ctrl Pts',(1.5129078685785E-11,-177.193984254242,
8.40164026751963));
#32839=CARTESIAN_POINT('Ctrl Pts',(4.85068927010198,-177.018984254242,8.4016402675109));
#32840=CARTESIAN_POINT('Ctrl Pts',(7.27603390513785,-176.843984254242,4.20082013374672));
#32841=CARTESIAN_POINT('Ctrl Pts',(9.70137854017372,-176.668984254242,-1.74689612655491E-11));
#32842=CARTESIAN_POINT('Ctrl Pts',(7.27603390512273,-176.493984254242,-4.20082013377291));
#32843=CARTESIAN_POINT('Ctrl Pts',(4.85068927007173,-176.318984254242,-8.40164026752836));
#32844=CARTESIAN_POINT('Ctrl Pts',(-1.51301075899711E-11,-176.143984254242,
-8.40164026751963));
#32845=CARTESIAN_POINT('Ctrl Pts',(-4.85068927010199,-175.968984254242,
-8.4016402675109));
#32846=CARTESIAN_POINT('Ctrl Pts',(-7.27603390513785,-175.793984254242,
-4.20082013374671));
#32847=CARTESIAN_POINT('Ctrl Pts',(-9.70137854017372,-175.618984254242,
1.74701493417668E-11));
#32848=CARTESIAN_POINT('Ctrl Pts',(-7.27603390512272,-175.443984254242,
4.20082013377292));
#32849=CARTESIAN_POINT('Ctrl Pts',(-4.85068927007173,-175.268984254242,
8.40164026752836));
#32850=CARTESIAN_POINT('Ctrl Pts',(1.5129078685785E-11,-175.093984254242,
8.40164026751963));
#32851=CARTESIAN_POINT('Ctrl Pts',(4.85068927010198,-174.918984254242,8.4016402675109));
#32852=CARTESIAN_POINT('Ctrl Pts',(7.27603390513785,-174.743984254242,4.20082013374672));
#32853=CARTESIAN_POINT('Ctrl Pts',(9.70137854017372,-174.568984254242,-1.74689612655491E-11));
#32854=CARTESIAN_POINT('Ctrl Pts',(7.27603390512273,-174.393984254242,-4.20082013377291));
#32855=CARTESIAN_POINT('Ctrl Pts',(4.85068927007173,-174.218984254242,-8.40164026752836));
#32856=CARTESIAN_POINT('Ctrl Pts',(-1.51301075899711E-11,-174.043984254242,
-8.40164026751963));
#32857=CARTESIAN_POINT('Ctrl Pts',(-4.85068927010199,-173.868984254242,
-8.4016402675109));
#32858=CARTESIAN_POINT('Ctrl Pts',(-7.27603390513785,-173.693984254242,
-4.20082013374671));
#32859=CARTESIAN_POINT('Ctrl Pts',(-9.70137854017372,-173.518984254242,
1.74701493417668E-11));
#32860=CARTESIAN_POINT('Ctrl Pts',(-7.27603390512272,-173.343984254242,
4.20082013377292));
#32861=CARTESIAN_POINT('Ctrl Pts',(-4.85068927007173,-173.168984254242,
8.40164026752836));
#32862=CARTESIAN_POINT('Ctrl Pts',(1.5129078685785E-11,-172.993984254242,
8.40164026751963));
#32863=CARTESIAN_POINT('Ctrl Pts',(4.85068927010198,-172.818984254242,8.4016402675109));
#32864=CARTESIAN_POINT('Ctrl Pts',(7.27603390513785,-172.643984254242,4.20082013374672));
#32865=CARTESIAN_POINT('Ctrl Pts',(9.70137854017372,-172.468984254242,-1.74689612655491E-11));
#32866=CARTESIAN_POINT('Ctrl Pts',(7.27603390512273,-172.293984254242,-4.20082013377291));
#32867=CARTESIAN_POINT('Ctrl Pts',(4.85068927007173,-172.118984254242,-8.40164026752836));
#32868=CARTESIAN_POINT('Ctrl Pts',(-1.51301075899711E-11,-171.943984254242,
-8.40164026751963));
#32869=CARTESIAN_POINT('Ctrl Pts',(-4.85068927010199,-171.768984254242,
-8.4016402675109));
#32870=CARTESIAN_POINT('Ctrl Pts',(-7.27603390513785,-171.593984254242,
-4.20082013374671));
#32871=CARTESIAN_POINT('Ctrl Pts',(-9.70137854017372,-171.418984254242,
1.74701493417668E-11));
#32872=CARTESIAN_POINT('Ctrl Pts',(-7.27603390512272,-171.243984254242,
4.20082013377292));
#32873=CARTESIAN_POINT('Ctrl Pts',(-4.85068927007173,-171.068984254242,
8.40164026752836));
#32874=CARTESIAN_POINT('Ctrl Pts',(1.5129078685785E-11,-170.893984254242,
8.40164026751963));
#32875=CARTESIAN_POINT('Ctrl Pts',(4.85068927010198,-170.718984254242,8.4016402675109));
#32876=CARTESIAN_POINT('Ctrl Pts',(7.27603390513785,-170.543984254242,4.20082013374672));
#32877=CARTESIAN_POINT('Ctrl Pts',(9.70137854017372,-170.368984254242,-1.74689612655491E-11));
#32878=CARTESIAN_POINT('Ctrl Pts',(7.27603390512273,-170.193984254242,-4.20082013377291));
#32879=CARTESIAN_POINT('Ctrl Pts',(4.85068927007173,-170.018984254242,-8.40164026752836));
#32880=CARTESIAN_POINT('Ctrl Pts',(-1.51301075899711E-11,-169.843984254242,
-8.40164026751963));
#32881=CARTESIAN_POINT('Ctrl Pts',(-4.85068927010199,-169.668984254242,
-8.4016402675109));
#32882=CARTESIAN_POINT('Ctrl Pts',(-7.27603390513785,-169.493984254242,
-4.20082013374671));
#32883=CARTESIAN_POINT('Ctrl Pts',(-9.70137854017372,-169.318984254242,
1.74701493417668E-11));
#32884=CARTESIAN_POINT('Ctrl Pts',(-7.27603390512272,-169.143984254242,
4.20082013377292));
#32885=CARTESIAN_POINT('Ctrl Pts',(-4.85068927007173,-168.968984254242,
8.40164026752836));
#32886=CARTESIAN_POINT('Ctrl Pts',(1.5129078685785E-11,-168.793984254242,
8.40164026751963));
#32887=CARTESIAN_POINT('Ctrl Pts',(4.85068927010198,-168.618984254242,8.4016402675109));
#32888=CARTESIAN_POINT('Ctrl Pts',(7.27603390513785,-168.443984254242,4.20082013374672));
#32889=CARTESIAN_POINT('Ctrl Pts',(9.70137854017372,-168.268984254242,-1.74689612655491E-11));
#32890=CARTESIAN_POINT('Ctrl Pts',(7.27603390512273,-168.093984254242,-4.20082013377291));
#32891=CARTESIAN_POINT('Ctrl Pts',(4.85068927007173,-167.918984254242,-8.40164026752836));
#32892=CARTESIAN_POINT('Ctrl Pts',(-1.51301075899711E-11,-167.743984254242,
-8.40164026751963));
#32893=CARTESIAN_POINT('Ctrl Pts',(-4.85068927010199,-167.568984254242,
-8.4016402675109));
#32894=CARTESIAN_POINT('Ctrl Pts',(-7.27603390513785,-167.393984254242,
-4.20082013374671));
#32895=CARTESIAN_POINT('Ctrl Pts',(-9.70137854017372,-167.218984254242,
1.74701493417668E-11));
#32896=CARTESIAN_POINT('Ctrl Pts',(-7.27603390512272,-167.043984254242,
4.20082013377292));
#32897=CARTESIAN_POINT('Ctrl Pts',(-4.85068927007173,-166.868984254242,
8.40164026752836));
#32898=CARTESIAN_POINT('Ctrl Pts',(1.5129078685785E-11,-166.693984254242,
8.40164026751963));
#32899=CARTESIAN_POINT('Ctrl Pts',(4.85068927010198,-166.518984254242,8.4016402675109));
#32900=CARTESIAN_POINT('Ctrl Pts',(7.27603390513785,-166.343984254242,4.20082013374672));
#32901=CARTESIAN_POINT('Ctrl Pts',(9.70137854017372,-166.168984254242,-1.74689612655491E-11));
#32902=CARTESIAN_POINT('Ctrl Pts',(7.27603390512273,-165.993984254242,-4.20082013377291));
#32903=CARTESIAN_POINT('Ctrl Pts',(4.85068927007173,-165.818984254242,-8.40164026752836));
#32904=CARTESIAN_POINT('Ctrl Pts',(-1.51301075899711E-11,-165.643984254242,
-8.40164026751963));
#32905=CARTESIAN_POINT('Ctrl Pts',(-4.85068927010199,-165.468984254242,
-8.4016402675109));
#32906=CARTESIAN_POINT('Ctrl Pts',(-7.27603390513785,-165.293984254242,
-4.20082013374671));
#32907=CARTESIAN_POINT('Ctrl Pts',(-9.70137854017372,-165.118984254242,
1.74701493417668E-11));
#32908=CARTESIAN_POINT('Ctrl Pts',(-7.27603390512272,-164.943984254242,
4.20082013377292));
#32909=CARTESIAN_POINT('Ctrl Pts',(-4.85068927007173,-164.768984254242,
8.40164026752836));
#32910=CARTESIAN_POINT('Ctrl Pts',(1.5129078685785E-11,-164.593984254242,
8.40164026751963));
#32911=CARTESIAN_POINT('Ctrl Pts',(4.85068927010198,-164.418984254242,8.4016402675109));
#32912=CARTESIAN_POINT('Ctrl Pts',(7.27603390513785,-164.243984254242,4.20082013374672));
#32913=CARTESIAN_POINT('Ctrl Pts',(9.70137854017372,-164.068984254242,-1.74689612655491E-11));
#32914=CARTESIAN_POINT('Ctrl Pts',(7.27603390512273,-163.893984254242,-4.20082013377291));
#32915=CARTESIAN_POINT('Ctrl Pts',(4.85068927007173,-163.718984254242,-8.40164026752836));
#32916=CARTESIAN_POINT('Ctrl Pts',(-1.51301075899711E-11,-163.543984254242,
-8.40164026751963));
#32917=CARTESIAN_POINT('Ctrl Pts',(-4.85068927010199,-163.368984254242,
-8.4016402675109));
#32918=CARTESIAN_POINT('Ctrl Pts',(-7.27603390513785,-163.193984254242,
-4.20082013374671));
#32919=CARTESIAN_POINT('Ctrl Pts',(-9.70137854017372,-163.018984254242,
1.74701493417668E-11));
#32920=CARTESIAN_POINT('Ctrl Pts',(-7.27603390512272,-162.843984254242,
4.20082013377292));
#32921=CARTESIAN_POINT('Ctrl Pts',(-4.85068927007173,-162.668984254242,
8.40164026752836));
#32922=CARTESIAN_POINT('Ctrl Pts',(1.5129078685785E-11,-162.493984254242,
8.40164026751963));
#32923=CARTESIAN_POINT('Ctrl Pts',(4.85068927010198,-162.318984254242,8.4016402675109));
#32924=CARTESIAN_POINT('Ctrl Pts',(7.27603390513785,-162.143984254242,4.20082013374672));
#32925=CARTESIAN_POINT('Ctrl Pts',(9.70137854017372,-161.968984254242,-1.74689612655491E-11));
#32926=CARTESIAN_POINT('Ctrl Pts',(7.27603390512273,-161.793984254242,-4.20082013377291));
#32927=CARTESIAN_POINT('Ctrl Pts',(4.85068927007173,-161.618984254242,-8.40164026752836));
#32928=CARTESIAN_POINT('Ctrl Pts',(-1.51301075899711E-11,-161.443984254242,
-8.40164026751963));
#32929=CARTESIAN_POINT('Ctrl Pts',(-4.85068927010199,-161.268984254242,
-8.4016402675109));
#32930=CARTESIAN_POINT('Ctrl Pts',(-7.27603390513785,-161.093984254242,
-4.20082013374671));
#32931=CARTESIAN_POINT('Ctrl Pts',(-9.70137854017372,-160.918984254242,
1.74701493417668E-11));
#32932=CARTESIAN_POINT('Ctrl Pts',(-7.27603390512272,-160.743984254242,
4.20082013377292));
#32933=CARTESIAN_POINT('Ctrl Pts',(-4.85068927007173,-160.568984254242,
8.40164026752836));
#32934=CARTESIAN_POINT('Ctrl Pts',(1.5129078685785E-11,-160.393984254242,
8.40164026751963));
#32935=CARTESIAN_POINT('Ctrl Pts',(4.85068927010198,-160.218984254242,8.4016402675109));
#32936=CARTESIAN_POINT('Ctrl Pts',(7.27603390513785,-160.043984254242,4.20082013374672));
#32937=CARTESIAN_POINT('Ctrl Pts',(9.70137854017372,-159.868984254242,-1.74689612655491E-11));
#32938=CARTESIAN_POINT('Ctrl Pts',(7.27603390512273,-159.693984254242,-4.20082013377291));
#32939=CARTESIAN_POINT('Ctrl Pts',(4.85068927007173,-159.518984254242,-8.40164026752836));
#32940=CARTESIAN_POINT('Ctrl Pts',(-1.51301075899711E-11,-159.343984254242,
-8.40164026751963));
#32941=CARTESIAN_POINT('Ctrl Pts',(-4.85068927010199,-159.168984254242,
-8.4016402675109));
#32942=CARTESIAN_POINT('Ctrl Pts',(-7.27603390513785,-158.993984254242,
-4.20082013374671));
#32943=CARTESIAN_POINT('Ctrl Pts',(-9.70137854017372,-158.818984254242,
1.74701493417668E-11));
#32944=CARTESIAN_POINT('Ctrl Pts',(-7.27603390512272,-158.643984254242,
4.20082013377292));
#32945=CARTESIAN_POINT('Ctrl Pts',(-4.85068927007173,-158.468984254242,
8.40164026752836));
#32946=CARTESIAN_POINT('Ctrl Pts',(1.5129078685785E-11,-158.293984254242,
8.40164026751963));
#32947=CARTESIAN_POINT('Ctrl Pts',(4.85068927010198,-158.118984254242,8.4016402675109));
#32948=CARTESIAN_POINT('Ctrl Pts',(7.27603390513785,-157.943984254242,4.20082013374672));
#32949=CARTESIAN_POINT('Ctrl Pts',(9.70137854017372,-157.768984254242,-1.74689612655491E-11));
#32950=CARTESIAN_POINT('Ctrl Pts',(7.27603390512273,-157.593984254242,-4.20082013377291));
#32951=CARTESIAN_POINT('Ctrl Pts',(4.85068927007173,-157.418984254242,-8.40164026752836));
#32952=CARTESIAN_POINT('Ctrl Pts',(-1.51301075899711E-11,-157.243984254242,
-8.40164026751963));
#32953=CARTESIAN_POINT('Ctrl Pts',(-4.85068927010199,-157.068984254242,
-8.4016402675109));
#32954=CARTESIAN_POINT('Ctrl Pts',(-7.27603390513785,-156.893984254242,
-4.20082013374671));
#32955=CARTESIAN_POINT('Ctrl Pts',(-9.70137854017372,-156.718984254242,
1.74701493417668E-11));
#32956=CARTESIAN_POINT('Ctrl Pts',(-7.27603390512272,-156.543984254242,
4.20082013377292));
#32957=CARTESIAN_POINT('Ctrl Pts',(-4.85068927007173,-156.368984254242,
8.40164026752836));
#32958=CARTESIAN_POINT('Ctrl Pts',(1.5129078685785E-11,-156.193984254242,
8.40164026751963));
#32959=CARTESIAN_POINT('Ctrl Pts',(4.85068927010198,-156.018984254242,8.4016402675109));
#32960=CARTESIAN_POINT('Ctrl Pts',(7.27603390513785,-155.843984254242,4.20082013374672));
#32961=CARTESIAN_POINT('Ctrl Pts',(9.70137854017372,-155.668984254242,-1.74689612655491E-11));
#32962=CARTESIAN_POINT('Ctrl Pts',(7.27603390512273,-155.493984254242,-4.20082013377291));
#32963=CARTESIAN_POINT('Ctrl Pts',(4.85068927007173,-155.318984254242,-8.40164026752836));
#32964=CARTESIAN_POINT('Ctrl Pts',(-1.51301075899711E-11,-155.143984254242,
-8.40164026751963));
#32965=CARTESIAN_POINT('Ctrl Pts',(-4.85068927010199,-154.968984254242,
-8.4016402675109));
#32966=CARTESIAN_POINT('Ctrl Pts',(-7.27603390513785,-154.793984254242,
-4.20082013374671));
#32967=CARTESIAN_POINT('Ctrl Pts',(-9.70137854017372,-154.618984254242,
1.74701493417668E-11));
#32968=CARTESIAN_POINT('Ctrl Pts',(-7.27603390512272,-154.443984254242,
4.20082013377292));
#32969=CARTESIAN_POINT('Ctrl Pts',(-4.85068927007173,-154.268984254242,
8.40164026752836));
#32970=CARTESIAN_POINT('Ctrl Pts',(1.5129078685785E-11,-154.093984254242,
8.40164026751963));
#32971=CARTESIAN_POINT('Ctrl Pts',(4.85068927010198,-153.918984254242,8.4016402675109));
#32972=CARTESIAN_POINT('Ctrl Pts',(7.27603390513785,-153.743984254242,4.20082013374672));
#32973=CARTESIAN_POINT('Ctrl Pts',(9.70137854017372,-153.568984254242,-1.74689612655491E-11));
#32974=CARTESIAN_POINT('Ctrl Pts',(7.27603390512273,-153.393984254242,-4.20082013377291));
#32975=CARTESIAN_POINT('Ctrl Pts',(4.85068927007173,-153.218984254242,-8.40164026752836));
#32976=CARTESIAN_POINT('Ctrl Pts',(-1.51301075899711E-11,-153.043984254242,
-8.40164026751963));
#32977=CARTESIAN_POINT('Ctrl Pts',(-4.85068927010199,-152.868984254242,
-8.4016402675109));
#32978=CARTESIAN_POINT('Ctrl Pts',(-7.27603390513785,-152.693984254242,
-4.20082013374671));
#32979=CARTESIAN_POINT('Ctrl Pts',(-9.70137854017372,-152.518984254242,
1.74701493417668E-11));
#32980=CARTESIAN_POINT('Ctrl Pts',(-7.27603390512272,-152.343984254242,
4.20082013377292));
#32981=CARTESIAN_POINT('Ctrl Pts',(-4.85068927007173,-152.168984254242,
8.40164026752836));
#32982=CARTESIAN_POINT('Ctrl Pts',(1.5129078685785E-11,-151.993984254242,
8.40164026751963));
#32983=CARTESIAN_POINT('Ctrl Pts',(4.85068927010198,-151.818984254242,8.4016402675109));
#32984=CARTESIAN_POINT('Ctrl Pts',(7.27603390513785,-151.643984254242,4.20082013374672));
#32985=CARTESIAN_POINT('Ctrl Pts',(9.70137854017372,-151.468984254242,-1.74689612655491E-11));
#32986=CARTESIAN_POINT('Ctrl Pts',(7.27603390512273,-151.293984254242,-4.20082013377291));
#32987=CARTESIAN_POINT('Ctrl Pts',(4.85068927007173,-151.118984254242,-8.40164026752836));
#32988=CARTESIAN_POINT('Ctrl Pts',(-1.51301075899711E-11,-150.943984254242,
-8.40164026751963));
#32989=CARTESIAN_POINT('Ctrl Pts',(-4.85068927010199,-150.768984254242,
-8.4016402675109));
#32990=CARTESIAN_POINT('Ctrl Pts',(-7.27603390513785,-150.593984254242,
-4.20082013374671));
#32991=CARTESIAN_POINT('Ctrl Pts',(-9.70137854017372,-150.418984254242,
1.74701493417668E-11));
#32992=CARTESIAN_POINT('Ctrl Pts',(-7.27603390512272,-150.243984254242,
4.20082013377292));
#32993=CARTESIAN_POINT('Ctrl Pts',(-4.85068927007173,-150.068984254242,
8.40164026752836));
#32994=CARTESIAN_POINT('Ctrl Pts',(1.5129078685785E-11,-149.893984254242,
8.40164026751963));
#32995=CARTESIAN_POINT('Ctrl Pts',(4.85068927010198,-149.718984254242,8.4016402675109));
#32996=CARTESIAN_POINT('Ctrl Pts',(7.27603390513785,-149.543984254242,4.20082013374672));
#32997=CARTESIAN_POINT('Ctrl Pts',(9.70137854017372,-149.368984254242,-1.74689612655491E-11));
#32998=CARTESIAN_POINT('Ctrl Pts',(7.27603390512273,-149.193984254242,-4.20082013377291));
#32999=CARTESIAN_POINT('Ctrl Pts',(4.85068927007173,-149.018984254242,-8.40164026752836));
#33000=CARTESIAN_POINT('Ctrl Pts',(-1.51301075899711E-11,-148.843984254242,
-8.40164026751963));
#33001=CARTESIAN_POINT('Ctrl Pts',(-4.85068927010199,-148.668984254242,
-8.4016402675109));
#33002=CARTESIAN_POINT('Ctrl Pts',(-7.27603390513785,-148.493984254242,
-4.20082013374671));
#33003=CARTESIAN_POINT('Ctrl Pts',(-9.70137854017372,-148.318984254242,
1.74701493417668E-11));
#33004=CARTESIAN_POINT('Ctrl Pts',(-7.27603390512272,-148.143984254242,
4.20082013377292));
#33005=CARTESIAN_POINT('Ctrl Pts',(-4.85068927007173,-147.968984254242,
8.40164026752836));
#33006=CARTESIAN_POINT('Ctrl Pts',(1.5129078685785E-11,-147.793984254242,
8.40164026751963));
#33007=CARTESIAN_POINT('Ctrl Pts',(4.85068927010198,-147.618984254242,8.4016402675109));
#33008=CARTESIAN_POINT('Ctrl Pts',(7.27603390513785,-147.443984254242,4.20082013374672));
#33009=CARTESIAN_POINT('Ctrl Pts',(9.70137854017372,-147.268984254242,-1.74689612655491E-11));
#33010=CARTESIAN_POINT('Ctrl Pts',(7.27603390512273,-147.093984254242,-4.20082013377291));
#33011=CARTESIAN_POINT('Ctrl Pts',(4.85068927007173,-146.918984254242,-8.40164026752836));
#33012=CARTESIAN_POINT('Ctrl Pts',(-1.51301075899711E-11,-146.743984254242,
-8.40164026751963));
#33013=CARTESIAN_POINT('Ctrl Pts',(-4.85068927010199,-146.568984254242,
-8.4016402675109));
#33014=CARTESIAN_POINT('Ctrl Pts',(-7.27603390513785,-146.393984254242,
-4.20082013374671));
#33015=CARTESIAN_POINT('Ctrl Pts',(-9.70137854017372,-146.218984254242,
1.74701493417668E-11));
#33016=CARTESIAN_POINT('Ctrl Pts',(-7.27603390512272,-146.043984254242,
4.20082013377292));
#33017=CARTESIAN_POINT('Ctrl Pts',(-4.85068927007173,-145.868984254242,
8.40164026752836));
#33018=CARTESIAN_POINT('Ctrl Pts',(1.5129078685785E-11,-145.693984254242,
8.40164026751963));
#33019=CARTESIAN_POINT('Ctrl Pts',(4.85068927010198,-145.518984254242,8.4016402675109));
#33020=CARTESIAN_POINT('Ctrl Pts',(7.27603390513785,-145.343984254242,4.20082013374672));
#33021=CARTESIAN_POINT('Ctrl Pts',(9.70137854017372,-145.168984254242,-1.74689612655491E-11));
#33022=CARTESIAN_POINT('Ctrl Pts',(7.27603390512273,-144.993984254242,-4.20082013377291));
#33023=CARTESIAN_POINT('Ctrl Pts',(4.85068927007173,-144.818984254242,-8.40164026752836));
#33024=CARTESIAN_POINT('Ctrl Pts',(-1.51301075899711E-11,-144.643984254242,
-8.40164026751963));
#33025=CARTESIAN_POINT('Ctrl Pts',(-4.85068927010199,-144.468984254242,
-8.4016402675109));
#33026=CARTESIAN_POINT('Ctrl Pts',(-7.27603390513785,-144.293984254242,
-4.20082013374671));
#33027=CARTESIAN_POINT('Ctrl Pts',(-9.70137854017372,-144.118984254242,
1.74701493417668E-11));
#33028=CARTESIAN_POINT('Ctrl Pts',(-7.27603390512272,-143.943984254242,
4.20082013377292));
#33029=CARTESIAN_POINT('Ctrl Pts',(-4.85068927007173,-143.768984254242,
8.40164026752836));
#33030=CARTESIAN_POINT('Ctrl Pts',(1.5129078685785E-11,-143.593984254242,
8.40164026751963));
#33031=CARTESIAN_POINT('Ctrl Pts',(4.85068927010198,-143.418984254242,8.4016402675109));
#33032=CARTESIAN_POINT('Ctrl Pts',(7.27603390513785,-143.243984254242,4.20082013374672));
#33033=CARTESIAN_POINT('Ctrl Pts',(9.70137854017372,-143.068984254242,-1.74689612655491E-11));
#33034=CARTESIAN_POINT('Ctrl Pts',(7.27603390512273,-142.893984254242,-4.20082013377291));
#33035=CARTESIAN_POINT('Ctrl Pts',(4.85068927007173,-142.718984254242,-8.40164026752836));
#33036=CARTESIAN_POINT('Ctrl Pts',(-1.51301075899711E-11,-142.543984254242,
-8.40164026751963));
#33037=CARTESIAN_POINT('Ctrl Pts',(-4.85068927010199,-142.368984254242,
-8.4016402675109));
#33038=CARTESIAN_POINT('Ctrl Pts',(-7.27603390513785,-142.193984254242,
-4.20082013374671));
#33039=CARTESIAN_POINT('Ctrl Pts',(-9.70137854017372,-142.018984254242,
1.74701493417668E-11));
#33040=CARTESIAN_POINT('Ctrl Pts',(-7.27603390512272,-141.843984254242,
4.20082013377292));
#33041=CARTESIAN_POINT('Ctrl Pts',(-4.85068927007173,-141.668984254242,
8.40164026752836));
#33042=CARTESIAN_POINT('Ctrl Pts',(1.5129078685785E-11,-141.493984254242,
8.40164026751963));
#33043=CARTESIAN_POINT('Ctrl Pts',(4.85068927010198,-141.318984254242,8.4016402675109));
#33044=CARTESIAN_POINT('Ctrl Pts',(7.27603390513785,-141.143984254242,4.20082013374672));
#33045=CARTESIAN_POINT('Ctrl Pts',(9.70137854017372,-140.968984254242,-1.74689612655491E-11));
#33046=CARTESIAN_POINT('Ctrl Pts',(7.27603390512273,-140.793984254242,-4.20082013377291));
#33047=CARTESIAN_POINT('Ctrl Pts',(4.85068927007173,-140.618984254242,-8.40164026752836));
#33048=CARTESIAN_POINT('Ctrl Pts',(-1.51301075899711E-11,-140.443984254242,
-8.40164026751963));
#33049=CARTESIAN_POINT('Ctrl Pts',(-4.85068927010199,-140.268984254242,
-8.4016402675109));
#33050=CARTESIAN_POINT('Ctrl Pts',(-7.27603390513785,-140.093984254242,
-4.20082013374671));
#33051=CARTESIAN_POINT('Ctrl Pts',(-9.70137854017372,-139.918984254242,
1.74701493417668E-11));
#33052=CARTESIAN_POINT('Ctrl Pts',(-7.27603390512272,-139.743984254242,
4.20082013377292));
#33053=CARTESIAN_POINT('Ctrl Pts',(-4.85068927007173,-139.568984254242,
8.40164026752836));
#33054=CARTESIAN_POINT('Ctrl Pts',(1.5129078685785E-11,-139.393984254242,
8.40164026751963));
#33055=CARTESIAN_POINT('Ctrl Pts',(4.85068927010198,-139.218984254242,8.4016402675109));
#33056=CARTESIAN_POINT('Ctrl Pts',(7.27603390513785,-139.043984254242,4.20082013374672));
#33057=CARTESIAN_POINT('Ctrl Pts',(9.70137854017372,-138.868984254242,-1.74689612655491E-11));
#33058=CARTESIAN_POINT('Ctrl Pts',(7.27603390512273,-138.693984254242,-4.20082013377291));
#33059=CARTESIAN_POINT('Ctrl Pts',(4.85068927007173,-138.518984254242,-8.40164026752836));
#33060=CARTESIAN_POINT('Ctrl Pts',(-1.51301075899711E-11,-138.343984254242,
-8.40164026751963));
#33061=CARTESIAN_POINT('Ctrl Pts',(-4.85068927010199,-138.168984254242,
-8.4016402675109));
#33062=CARTESIAN_POINT('Ctrl Pts',(-7.27603390513785,-137.993984254242,
-4.20082013374671));
#33063=CARTESIAN_POINT('Ctrl Pts',(-9.70137854017372,-137.818984254242,
1.74701493417668E-11));
#33064=CARTESIAN_POINT('Ctrl Pts',(-7.27603390512272,-137.643984254242,
4.20082013377292));
#33065=CARTESIAN_POINT('Ctrl Pts',(-4.85068927007173,-137.468984254242,
8.40164026752836));
#33066=CARTESIAN_POINT('Ctrl Pts',(1.5129078685785E-11,-137.293984254242,
8.40164026751963));
#33067=CARTESIAN_POINT('Ctrl Pts',(4.85068927010198,-137.118984254242,8.4016402675109));
#33068=CARTESIAN_POINT('Ctrl Pts',(7.27603390513785,-136.943984254242,4.20082013374672));
#33069=CARTESIAN_POINT('Ctrl Pts',(9.70137854017372,-136.768984254242,-1.74689612655491E-11));
#33070=CARTESIAN_POINT('Ctrl Pts',(7.27603390512273,-136.593984254242,-4.20082013377291));
#33071=CARTESIAN_POINT('Ctrl Pts',(4.85068927007173,-136.418984254242,-8.40164026752836));
#33072=CARTESIAN_POINT('Ctrl Pts',(-1.51301075899711E-11,-136.243984254242,
-8.40164026751963));
#33073=CARTESIAN_POINT('Ctrl Pts',(-4.85068927010199,-136.068984254242,
-8.4016402675109));
#33074=CARTESIAN_POINT('Ctrl Pts',(-7.27603390513785,-135.893984254242,
-4.20082013374671));
#33075=CARTESIAN_POINT('Ctrl Pts',(-9.70137854017372,-135.718984254242,
1.74701493417668E-11));
#33076=CARTESIAN_POINT('Ctrl Pts',(-7.27603390512272,-135.543984254242,
4.20082013377292));
#33077=CARTESIAN_POINT('Ctrl Pts',(-4.85068927007173,-135.368984254242,
8.40164026752836));
#33078=CARTESIAN_POINT('Ctrl Pts',(1.5129078685785E-11,-135.193984254242,
8.40164026751963));
#33079=CARTESIAN_POINT('Ctrl Pts',(4.85068927010198,-135.018984254242,8.4016402675109));
#33080=CARTESIAN_POINT('Ctrl Pts',(7.27603390513785,-134.843984254242,4.20082013374672));
#33081=CARTESIAN_POINT('Ctrl Pts',(9.70137854017372,-134.668984254242,-1.74689612655491E-11));
#33082=CARTESIAN_POINT('Ctrl Pts',(7.27603390512273,-134.493984254242,-4.20082013377291));
#33083=CARTESIAN_POINT('Ctrl Pts',(4.85068927007173,-134.318984254242,-8.40164026752836));
#33084=CARTESIAN_POINT('Ctrl Pts',(-1.51301075899711E-11,-134.143984254242,
-8.40164026751963));
#33085=CARTESIAN_POINT('Ctrl Pts',(-4.85068927010199,-133.968984254242,
-8.4016402675109));
#33086=CARTESIAN_POINT('Ctrl Pts',(-7.27603390513785,-133.793984254242,
-4.20082013374671));
#33087=CARTESIAN_POINT('Ctrl Pts',(-9.70137854017372,-133.618984254242,
1.74701493417668E-11));
#33088=CARTESIAN_POINT('Ctrl Pts',(-7.27603390512272,-133.443984254242,
4.20082013377292));
#33089=CARTESIAN_POINT('Ctrl Pts',(-4.85068927007173,-133.268984254242,
8.40164026752836));
#33090=CARTESIAN_POINT('Ctrl Pts',(1.5129078685785E-11,-133.093984254242,
8.40164026751963));
#33091=CARTESIAN_POINT('Ctrl Pts',(4.85068927010198,-132.918984254242,8.4016402675109));
#33092=CARTESIAN_POINT('Ctrl Pts',(7.27603390513785,-132.743984254242,4.20082013374672));
#33093=CARTESIAN_POINT('Ctrl Pts',(9.70137854017372,-132.568984254242,-1.74689612655491E-11));
#33094=CARTESIAN_POINT('Ctrl Pts',(7.27603390512273,-132.393984254242,-4.20082013377291));
#33095=CARTESIAN_POINT('Ctrl Pts',(4.85068927007173,-132.218984254242,-8.40164026752836));
#33096=CARTESIAN_POINT('Ctrl Pts',(-1.51301075899711E-11,-132.043984254242,
-8.40164026751963));
#33097=CARTESIAN_POINT('Ctrl Pts',(-4.85068927010199,-131.868984254242,
-8.4016402675109));
#33098=CARTESIAN_POINT('Ctrl Pts',(-7.27603390513785,-131.693984254242,
-4.20082013374671));
#33099=CARTESIAN_POINT('Ctrl Pts',(-9.70137854017372,-131.518984254242,
1.74701493417668E-11));
#33100=CARTESIAN_POINT('Ctrl Pts',(-7.27603390512272,-131.343984254242,
4.20082013377292));
#33101=CARTESIAN_POINT('Ctrl Pts',(-4.85068927007173,-131.168984254242,
8.40164026752836));
#33102=CARTESIAN_POINT('Ctrl Pts',(1.5129078685785E-11,-130.993984254242,
8.40164026751963));
#33103=CARTESIAN_POINT('Ctrl Pts',(4.85068927010198,-130.818984254242,8.4016402675109));
#33104=CARTESIAN_POINT('Ctrl Pts',(7.27603390513785,-130.643984254242,4.20082013374672));
#33105=CARTESIAN_POINT('Ctrl Pts',(9.70137854017372,-130.468984254242,-1.74689612655491E-11));
#33106=CARTESIAN_POINT('Ctrl Pts',(7.27603390512273,-130.293984254242,-4.20082013377291));
#33107=CARTESIAN_POINT('Ctrl Pts',(4.85068927007173,-130.118984254242,-8.40164026752836));
#33108=CARTESIAN_POINT('Ctrl Pts',(-1.51301075899711E-11,-129.943984254242,
-8.40164026751963));
#33109=CARTESIAN_POINT('Ctrl Pts',(-4.85068927010199,-129.768984254242,
-8.4016402675109));
#33110=CARTESIAN_POINT('Ctrl Pts',(-7.27603390513785,-129.593984254242,
-4.20082013374671));
#33111=CARTESIAN_POINT('Ctrl Pts',(-9.70137854017372,-129.418984254242,
1.74701493417668E-11));
#33112=CARTESIAN_POINT('Ctrl Pts',(-7.27603390512272,-129.243984254242,
4.20082013377292));
#33113=CARTESIAN_POINT('Ctrl Pts',(-4.85068927007173,-129.068984254242,
8.40164026752836));
#33114=CARTESIAN_POINT('Ctrl Pts',(1.5129078685785E-11,-128.893984254242,
8.40164026751963));
#33115=CARTESIAN_POINT('Ctrl Pts',(4.85068927010198,-128.718984254242,8.4016402675109));
#33116=CARTESIAN_POINT('Ctrl Pts',(7.27603390513785,-128.543984254242,4.20082013374672));
#33117=CARTESIAN_POINT('Ctrl Pts',(9.70137854017372,-128.368984254242,-1.74689612655491E-11));
#33118=CARTESIAN_POINT('Ctrl Pts',(7.27603390512273,-128.193984254242,-4.20082013377291));
#33119=CARTESIAN_POINT('Ctrl Pts',(4.85068927007173,-128.018984254242,-8.40164026752836));
#33120=CARTESIAN_POINT('Ctrl Pts',(-1.51301075899711E-11,-127.843984254242,
-8.40164026751963));
#33121=CARTESIAN_POINT('Ctrl Pts',(-4.85068927010199,-127.668984254242,
-8.4016402675109));
#33122=CARTESIAN_POINT('Ctrl Pts',(-7.27603390513785,-127.493984254242,
-4.20082013374671));
#33123=CARTESIAN_POINT('Ctrl Pts',(-9.70137854017372,-127.318984254242,
1.74701493417668E-11));
#33124=CARTESIAN_POINT('Ctrl Pts',(-7.27603390512272,-127.143984254242,
4.20082013377292));
#33125=CARTESIAN_POINT('Ctrl Pts',(-4.85068927007173,-126.968984254242,
8.40164026752836));
#33126=CARTESIAN_POINT('Ctrl Pts',(1.5129078685785E-11,-126.793984254242,
8.40164026751963));
#33127=CARTESIAN_POINT('Ctrl Pts',(4.85068927010198,-126.618984254242,8.4016402675109));
#33128=CARTESIAN_POINT('Ctrl Pts',(7.27603390513785,-126.443984254242,4.20082013374672));
#33129=CARTESIAN_POINT('Ctrl Pts',(9.70137854017372,-126.268984254242,-1.74689612655491E-11));
#33130=CARTESIAN_POINT('Ctrl Pts',(7.27603390512273,-126.093984254242,-4.20082013377291));
#33131=CARTESIAN_POINT('Ctrl Pts',(4.85068927007173,-125.918984254242,-8.40164026752836));
#33132=CARTESIAN_POINT('Ctrl Pts',(-1.51301075899711E-11,-125.743984254242,
-8.40164026751963));
#33133=CARTESIAN_POINT('Ctrl Pts',(-4.85068927010199,-125.568984254242,
-8.4016402675109));
#33134=CARTESIAN_POINT('Ctrl Pts',(-7.27603390513785,-125.393984254242,
-4.20082013374671));
#33135=CARTESIAN_POINT('Ctrl Pts',(-9.70137854017372,-125.218984254242,
1.74701493417668E-11));
#33136=CARTESIAN_POINT('Ctrl Pts',(-7.27603390512272,-125.043984254242,
4.20082013377292));
#33137=CARTESIAN_POINT('Ctrl Pts',(-4.85068927007173,-124.868984254242,
8.40164026752836));
#33138=CARTESIAN_POINT('Ctrl Pts',(1.5129078685785E-11,-124.693984254242,
8.40164026751963));
#33139=CARTESIAN_POINT('Ctrl Pts',(4.85068927010198,-124.518984254242,8.4016402675109));
#33140=CARTESIAN_POINT('Ctrl Pts',(7.27603390513785,-124.343984254242,4.20082013374672));
#33141=CARTESIAN_POINT('Ctrl Pts',(9.70137854017372,-124.168984254242,-1.74689612655491E-11));
#33142=CARTESIAN_POINT('Ctrl Pts',(7.27603390512273,-123.993984254242,-4.20082013377291));
#33143=CARTESIAN_POINT('Ctrl Pts',(4.85068927007173,-123.818984254242,-8.40164026752836));
#33144=CARTESIAN_POINT('Ctrl Pts',(-1.51301075899711E-11,-123.643984254242,
-8.40164026751963));
#33145=CARTESIAN_POINT('Ctrl Pts',(-4.85068927010199,-123.468984254242,
-8.4016402675109));
#33146=CARTESIAN_POINT('Ctrl Pts',(-7.27603390513785,-123.293984254242,
-4.20082013374671));
#33147=CARTESIAN_POINT('Ctrl Pts',(-9.70137854017372,-123.118984254242,
1.74701493417668E-11));
#33148=CARTESIAN_POINT('Ctrl Pts',(-7.27603390512272,-122.943984254242,
4.20082013377292));
#33149=CARTESIAN_POINT('Ctrl Pts',(-4.85068927007173,-122.768984254242,
8.40164026752836));
#33150=CARTESIAN_POINT('Ctrl Pts',(1.5129078685785E-11,-122.593984254242,
8.40164026751963));
#33151=CARTESIAN_POINT('Ctrl Pts',(4.85068927010198,-122.418984254242,8.4016402675109));
#33152=CARTESIAN_POINT('Ctrl Pts',(7.27603390513785,-122.243984254242,4.20082013374672));
#33153=CARTESIAN_POINT('Ctrl Pts',(9.70137854017372,-122.068984254242,-1.74689612655491E-11));
#33154=CARTESIAN_POINT('Ctrl Pts',(7.27603390512273,-121.893984254242,-4.20082013377291));
#33155=CARTESIAN_POINT('Ctrl Pts',(4.85068927007173,-121.718984254242,-8.40164026752836));
#33156=CARTESIAN_POINT('Ctrl Pts',(-1.51301075899711E-11,-121.543984254242,
-8.40164026751963));
#33157=CARTESIAN_POINT('Ctrl Pts',(-4.85068927010199,-121.368984254242,
-8.4016402675109));
#33158=CARTESIAN_POINT('Ctrl Pts',(-7.27603390513785,-121.193984254242,
-4.20082013374671));
#33159=CARTESIAN_POINT('Ctrl Pts',(-9.70137854017372,-121.018984254242,
1.74701493417668E-11));
#33160=CARTESIAN_POINT('Ctrl Pts',(-7.27603390512272,-120.843984254242,
4.20082013377292));
#33161=CARTESIAN_POINT('Ctrl Pts',(-4.85068927007173,-120.668984254242,
8.40164026752836));
#33162=CARTESIAN_POINT('Ctrl Pts',(1.5129078685785E-11,-120.493984254242,
8.40164026751963));
#33163=CARTESIAN_POINT('Ctrl Pts',(4.85068927010198,-120.318984254242,8.4016402675109));
#33164=CARTESIAN_POINT('Ctrl Pts',(7.27603390513785,-120.143984254242,4.20082013374672));
#33165=CARTESIAN_POINT('Ctrl Pts',(9.70137854017372,-119.968984254242,-1.74689612655491E-11));
#33166=CARTESIAN_POINT('Ctrl Pts',(7.27603390512273,-119.793984254242,-4.20082013377291));
#33167=CARTESIAN_POINT('Ctrl Pts',(4.85068927007173,-119.618984254242,-8.40164026752836));
#33168=CARTESIAN_POINT('Ctrl Pts',(-1.51301075899711E-11,-119.443984254242,
-8.40164026751963));
#33169=CARTESIAN_POINT('Ctrl Pts',(-4.85068927010199,-119.268984254242,
-8.4016402675109));
#33170=CARTESIAN_POINT('Ctrl Pts',(-7.27603390513785,-119.093984254242,
-4.20082013374671));
#33171=CARTESIAN_POINT('Ctrl Pts',(-9.70137854017372,-118.918984254242,
1.74701493417668E-11));
#33172=CARTESIAN_POINT('Ctrl Pts',(-7.27603390512272,-118.743984254242,
4.20082013377292));
#33173=CARTESIAN_POINT('Ctrl Pts',(-4.85068927007173,-118.568984254242,
8.40164026752836));
#33174=CARTESIAN_POINT('Ctrl Pts',(1.5129078685785E-11,-118.393984254242,
8.40164026751963));
#33175=CARTESIAN_POINT('Ctrl Pts',(4.85068927010198,-118.218984254242,8.4016402675109));
#33176=CARTESIAN_POINT('Ctrl Pts',(7.27603390513785,-118.043984254242,4.20082013374672));
#33177=CARTESIAN_POINT('Ctrl Pts',(9.70137854017372,-117.868984254242,-1.74689612655491E-11));
#33178=CARTESIAN_POINT('Ctrl Pts',(7.27603390512273,-117.693984254242,-4.20082013377291));
#33179=CARTESIAN_POINT('Ctrl Pts',(4.85068927007173,-117.518984254242,-8.40164026752836));
#33180=CARTESIAN_POINT('Ctrl Pts',(-1.51301075899711E-11,-117.343984254242,
-8.40164026751963));
#33181=CARTESIAN_POINT('Ctrl Pts',(-4.85068927010199,-117.168984254242,
-8.4016402675109));
#33182=CARTESIAN_POINT('Ctrl Pts',(-7.27603390513785,-116.993984254242,
-4.20082013374671));
#33183=CARTESIAN_POINT('Ctrl Pts',(-9.70137854017372,-116.818984254242,
1.74701493417668E-11));
#33184=CARTESIAN_POINT('Ctrl Pts',(-7.27603390512272,-116.643984254242,
4.20082013377292));
#33185=CARTESIAN_POINT('Ctrl Pts',(-4.85068927007173,-116.468984254242,
8.40164026752836));
#33186=CARTESIAN_POINT('Ctrl Pts',(1.5129078685785E-11,-116.293984254242,
8.40164026751963));
#33187=CARTESIAN_POINT('Ctrl Pts',(4.85068927010198,-116.118984254242,8.4016402675109));
#33188=CARTESIAN_POINT('Ctrl Pts',(7.27603390513785,-115.943984254242,4.20082013374672));
#33189=CARTESIAN_POINT('Ctrl Pts',(9.70137854017372,-115.768984254242,-1.74689612655491E-11));
#33190=CARTESIAN_POINT('Ctrl Pts',(7.27603390512273,-115.593984254242,-4.20082013377291));
#33191=CARTESIAN_POINT('Ctrl Pts',(4.85068927007173,-115.418984254242,-8.40164026752836));
#33192=CARTESIAN_POINT('Ctrl Pts',(-1.51301075899711E-11,-115.243984254242,
-8.40164026751963));
#33193=CARTESIAN_POINT('Ctrl Pts',(-4.85068927010199,-115.068984254242,
-8.4016402675109));
#33194=CARTESIAN_POINT('Ctrl Pts',(-7.27603390513785,-114.893984254242,
-4.20082013374671));
#33195=CARTESIAN_POINT('Ctrl Pts',(-9.70137854017372,-114.718984254242,
1.74701493417668E-11));
#33196=CARTESIAN_POINT('Ctrl Pts',(-7.27603390512272,-114.543984254242,
4.20082013377292));
#33197=CARTESIAN_POINT('Ctrl Pts',(-4.85068927007173,-114.368984254242,
8.40164026752836));
#33198=CARTESIAN_POINT('Ctrl Pts',(1.5129078685785E-11,-114.193984254242,
8.40164026751963));
#33199=CARTESIAN_POINT('Ctrl Pts',(4.85068927010198,-114.018984254242,8.4016402675109));
#33200=CARTESIAN_POINT('Ctrl Pts',(7.27603390513785,-113.843984254242,4.20082013374672));
#33201=CARTESIAN_POINT('Ctrl Pts',(9.70137854017372,-113.668984254242,-1.74689612655491E-11));
#33202=CARTESIAN_POINT('Ctrl Pts',(7.27603390512273,-113.493984254242,-4.20082013377291));
#33203=CARTESIAN_POINT('Ctrl Pts',(4.85068927007173,-113.318984254242,-8.40164026752836));
#33204=CARTESIAN_POINT('Ctrl Pts',(-1.51301075899711E-11,-113.143984254242,
-8.40164026751963));
#33205=CARTESIAN_POINT('Ctrl Pts',(-4.85068927010199,-112.968984254242,
-8.4016402675109));
#33206=CARTESIAN_POINT('Ctrl Pts',(-7.27603390513785,-112.793984254242,
-4.20082013374671));
#33207=CARTESIAN_POINT('Ctrl Pts',(-9.70137854017372,-112.618984254242,
1.74701493417668E-11));
#33208=CARTESIAN_POINT('Ctrl Pts',(-7.27603390512272,-112.443984254242,
4.20082013377292));
#33209=CARTESIAN_POINT('Ctrl Pts',(-4.85068927007173,-112.268984254242,
8.40164026752836));
#33210=CARTESIAN_POINT('Ctrl Pts',(1.5129078685785E-11,-112.093984254242,
8.40164026751963));
#33211=CARTESIAN_POINT('Ctrl Pts',(4.85068927010198,-111.918984254242,8.4016402675109));
#33212=CARTESIAN_POINT('Ctrl Pts',(7.27603390513785,-111.743984254242,4.20082013374672));
#33213=CARTESIAN_POINT('Ctrl Pts',(9.70137854017372,-111.568984254242,-1.74689612655491E-11));
#33214=CARTESIAN_POINT('Ctrl Pts',(7.27603390512273,-111.393984254242,-4.20082013377291));
#33215=CARTESIAN_POINT('Ctrl Pts',(4.85068927007173,-111.218984254242,-8.40164026752836));
#33216=CARTESIAN_POINT('Ctrl Pts',(-1.51301075899711E-11,-111.043984254242,
-8.40164026751963));
#33217=CARTESIAN_POINT('Ctrl Pts',(-4.85068927010199,-110.868984254242,
-8.4016402675109));
#33218=CARTESIAN_POINT('Ctrl Pts',(-7.27603390513785,-110.693984254242,
-4.20082013374671));
#33219=CARTESIAN_POINT('Ctrl Pts',(-9.70137854017372,-110.518984254242,
1.74701493417668E-11));
#33220=CARTESIAN_POINT('Ctrl Pts',(-7.27603390512272,-110.343984254242,
4.20082013377292));
#33221=CARTESIAN_POINT('Ctrl Pts',(-4.85068927007173,-110.168984254242,
8.40164026752836));
#33222=CARTESIAN_POINT('Ctrl Pts',(1.5129078685785E-11,-109.993984254242,
8.40164026751963));
#33223=CARTESIAN_POINT('Ctrl Pts',(4.85068927010198,-109.818984254242,8.4016402675109));
#33224=CARTESIAN_POINT('Ctrl Pts',(7.27603390513785,-109.643984254242,4.20082013374672));
#33225=CARTESIAN_POINT('Ctrl Pts',(9.70137854017372,-109.468984254242,-1.74689612655491E-11));
#33226=CARTESIAN_POINT('Ctrl Pts',(7.27603390512273,-109.293984254242,-4.20082013377291));
#33227=CARTESIAN_POINT('Ctrl Pts',(4.85068927007173,-109.118984254242,-8.40164026752836));
#33228=CARTESIAN_POINT('Ctrl Pts',(-1.51301075899711E-11,-108.943984254242,
-8.40164026751963));
#33229=CARTESIAN_POINT('Ctrl Pts',(-4.85068927010199,-108.768984254242,
-8.4016402675109));
#33230=CARTESIAN_POINT('Ctrl Pts',(-7.27603390513785,-108.593984254242,
-4.20082013374671));
#33231=CARTESIAN_POINT('Ctrl Pts',(-9.70137854017372,-108.418984254242,
1.74701493417668E-11));
#33232=CARTESIAN_POINT('Ctrl Pts',(-7.27603390512272,-108.243984254242,
4.20082013377292));
#33233=CARTESIAN_POINT('Ctrl Pts',(-4.85068927007173,-108.068984254242,
8.40164026752836));
#33234=CARTESIAN_POINT('Ctrl Pts',(1.5129078685785E-11,-107.893984254242,
8.40164026751963));
#33235=CARTESIAN_POINT('Ctrl Pts',(4.85068927010198,-107.718984254242,8.4016402675109));
#33236=CARTESIAN_POINT('Ctrl Pts',(7.27603390513785,-107.543984254242,4.20082013374672));
#33237=CARTESIAN_POINT('Ctrl Pts',(9.70137854017372,-107.368984254242,-1.74689612655491E-11));
#33238=CARTESIAN_POINT('Ctrl Pts',(7.27603390512273,-107.193984254242,-4.20082013377291));
#33239=CARTESIAN_POINT('Ctrl Pts',(4.85068927007173,-107.018984254242,-8.40164026752836));
#33240=CARTESIAN_POINT('Ctrl Pts',(-1.51301075899711E-11,-106.843984254242,
-8.40164026751963));
#33241=CARTESIAN_POINT('Ctrl Pts',(-4.85068927010199,-106.668984254242,
-8.4016402675109));
#33242=CARTESIAN_POINT('Ctrl Pts',(-7.27603390513785,-106.493984254242,
-4.20082013374671));
#33243=CARTESIAN_POINT('Ctrl Pts',(-9.70137854017372,-106.318984254242,
1.74701493417668E-11));
#33244=CARTESIAN_POINT('Ctrl Pts',(-7.27603390512272,-106.143984254242,
4.20082013377292));
#33245=CARTESIAN_POINT('Ctrl Pts',(-4.85068927007173,-105.968984254242,
8.40164026752836));
#33246=CARTESIAN_POINT('Ctrl Pts',(1.5129078685785E-11,-105.793984254242,
8.40164026751963));
#33247=CARTESIAN_POINT('Ctrl Pts',(4.85068927010198,-105.618984254242,8.4016402675109));
#33248=CARTESIAN_POINT('Ctrl Pts',(7.27603390513785,-105.443984254242,4.20082013374672));
#33249=CARTESIAN_POINT('Ctrl Pts',(9.70137854017372,-105.268984254242,-1.74689612655491E-11));
#33250=CARTESIAN_POINT('Ctrl Pts',(7.27603390512273,-105.093984254242,-4.20082013377291));
#33251=CARTESIAN_POINT('Ctrl Pts',(4.85068927007173,-104.918984254242,-8.40164026752836));
#33252=CARTESIAN_POINT('Ctrl Pts',(-1.51301075899711E-11,-104.743984254242,
-8.40164026751963));
#33253=CARTESIAN_POINT('Ctrl Pts',(-4.85068927010199,-104.568984254242,
-8.4016402675109));
#33254=CARTESIAN_POINT('Ctrl Pts',(-7.27603390513785,-104.393984254242,
-4.20082013374671));
#33255=CARTESIAN_POINT('Ctrl Pts',(-9.70137854017372,-104.218984254242,
1.74701493417668E-11));
#33256=CARTESIAN_POINT('Ctrl Pts',(-7.27603390512272,-104.043984254242,
4.20082013377292));
#33257=CARTESIAN_POINT('Ctrl Pts',(-4.85068927007173,-103.868984254242,
8.40164026752836));
#33258=CARTESIAN_POINT('Ctrl Pts',(1.5129078685785E-11,-103.693984254242,
8.40164026751963));
#33259=CARTESIAN_POINT('Ctrl Pts',(4.85068927010198,-103.518984254242,8.4016402675109));
#33260=CARTESIAN_POINT('Ctrl Pts',(7.27603390513785,-103.343984254242,4.20082013374672));
#33261=CARTESIAN_POINT('Ctrl Pts',(9.70137854017372,-103.168984254242,-1.74689612655491E-11));
#33262=CARTESIAN_POINT('Ctrl Pts',(7.27603390512273,-102.993984254242,-4.20082013377291));
#33263=CARTESIAN_POINT('Ctrl Pts',(4.85068927007173,-102.818984254242,-8.40164026752836));
#33264=CARTESIAN_POINT('Ctrl Pts',(-1.51301075899711E-11,-102.643984254242,
-8.40164026751963));
#33265=CARTESIAN_POINT('Ctrl Pts',(-4.85068927010199,-102.468984254242,
-8.4016402675109));
#33266=CARTESIAN_POINT('Ctrl Pts',(-7.27603390513785,-102.293984254242,
-4.20082013374671));
#33267=CARTESIAN_POINT('Ctrl Pts',(-9.70137854017372,-102.118984254242,
1.74701493417668E-11));
#33268=CARTESIAN_POINT('Ctrl Pts',(-7.27603390512272,-101.943984254242,
4.20082013377292));
#33269=CARTESIAN_POINT('Ctrl Pts',(-4.85068927007173,-101.768984254242,
8.40164026752836));
#33270=CARTESIAN_POINT('Ctrl Pts',(1.5129078685785E-11,-101.593984254242,
8.40164026751963));
#33271=CARTESIAN_POINT('Ctrl Pts',(4.85068927010198,-101.418984254242,8.4016402675109));
#33272=CARTESIAN_POINT('Ctrl Pts',(7.27603390513785,-101.243984254242,4.20082013374672));
#33273=CARTESIAN_POINT('Ctrl Pts',(9.70137854017372,-101.068984254242,-1.74689612655491E-11));
#33274=CARTESIAN_POINT('Ctrl Pts',(7.27603390512273,-100.893984254242,-4.20082013377291));
#33275=CARTESIAN_POINT('Ctrl Pts',(4.85068927007173,-100.718984254242,-8.40164026752836));
#33276=CARTESIAN_POINT('Ctrl Pts',(-1.51301075899711E-11,-100.543984254242,
-8.40164026751963));
#33277=CARTESIAN_POINT('Ctrl Pts',(-4.85068927010199,-100.368984254242,
-8.4016402675109));
#33278=CARTESIAN_POINT('Ctrl Pts',(-7.27603390513785,-100.193984254242,
-4.20082013374671));
#33279=CARTESIAN_POINT('Ctrl Pts',(-9.70137854017372,-100.018984254242,
1.74701493417668E-11));
#33280=CARTESIAN_POINT('Ctrl Pts',(-7.27603390512272,-99.8439842542419,
4.20082013377292));
#33281=CARTESIAN_POINT('Ctrl Pts',(-4.85068927007173,-99.6689842542419,
8.40164026752836));
#33282=CARTESIAN_POINT('Ctrl Pts',(1.5129078685785E-11,-99.4939842542419,
8.40164026751963));
#33283=CARTESIAN_POINT('Ctrl Pts',(4.85068927010198,-99.3189842542419,8.4016402675109));
#33284=CARTESIAN_POINT('Ctrl Pts',(7.27603390513785,-99.1439842542419,4.20082013374672));
#33285=CARTESIAN_POINT('Ctrl Pts',(9.70137854017372,-98.9689842542419,-1.74689612655491E-11));
#33286=CARTESIAN_POINT('Ctrl Pts',(7.27603390512273,-98.7939842542419,-4.20082013377291));
#33287=CARTESIAN_POINT('Ctrl Pts',(4.85068927007173,-98.6189842542419,-8.40164026752836));
#33288=CARTESIAN_POINT('Ctrl Pts',(-1.51301075899711E-11,-98.4439842542419,
-8.40164026751963));
#33289=CARTESIAN_POINT('Ctrl Pts',(-4.85068927010199,-98.2689842542419,
-8.4016402675109));
#33290=CARTESIAN_POINT('Ctrl Pts',(-7.27603390513785,-98.0939842542419,
-4.20082013374671));
#33291=CARTESIAN_POINT('Ctrl Pts',(-9.70137854017372,-97.9189842542419,
1.74701493417668E-11));
#33292=CARTESIAN_POINT('Ctrl Pts',(-7.27603390512272,-97.7439842542419,
4.20082013377292));
#33293=CARTESIAN_POINT('Ctrl Pts',(-4.85068927007173,-97.5689842542419,
8.40164026752836));
#33294=CARTESIAN_POINT('Ctrl Pts',(1.5129078685785E-11,-97.3939842542419,
8.40164026751963));
#33295=CARTESIAN_POINT('Ctrl Pts',(4.85068927010198,-97.2189842542419,8.4016402675109));
#33296=CARTESIAN_POINT('Ctrl Pts',(7.27603390513785,-97.0439842542419,4.20082013374672));
#33297=CARTESIAN_POINT('Ctrl Pts',(9.70137854017372,-96.8689842542419,-1.74689612655491E-11));
#33298=CARTESIAN_POINT('Ctrl Pts',(7.27603390512273,-96.6939842542419,-4.20082013377291));
#33299=CARTESIAN_POINT('Ctrl Pts',(4.85068927007173,-96.5189842542419,-8.40164026752836));
#33300=CARTESIAN_POINT('Ctrl Pts',(-1.51301075899711E-11,-96.3439842542419,
-8.40164026751963));
#33301=CARTESIAN_POINT('Ctrl Pts',(-4.85068927010199,-96.1689842542419,
-8.4016402675109));
#33302=CARTESIAN_POINT('Ctrl Pts',(-7.27603390513785,-95.9939842542419,
-4.20082013374671));
#33303=CARTESIAN_POINT('Ctrl Pts',(-9.70137854017372,-95.8189842542419,
1.74701493417668E-11));
#33304=CARTESIAN_POINT('Ctrl Pts',(-7.27603390512272,-95.6439842542419,
4.20082013377292));
#33305=CARTESIAN_POINT('Ctrl Pts',(-4.85068927007173,-95.4689842542419,
8.40164026752836));
#33306=CARTESIAN_POINT('Ctrl Pts',(1.5129078685785E-11,-95.2939842542419,
8.40164026751963));
#33307=CARTESIAN_POINT('Ctrl Pts',(4.85068927010198,-95.1189842542419,8.4016402675109));
#33308=CARTESIAN_POINT('Ctrl Pts',(7.27603390513785,-94.9439842542419,4.20082013374672));
#33309=CARTESIAN_POINT('Ctrl Pts',(9.70137854017372,-94.7689842542419,-1.74689612655491E-11));
#33310=CARTESIAN_POINT('Ctrl Pts',(7.27603390512273,-94.5939842542419,-4.20082013377291));
#33311=CARTESIAN_POINT('Ctrl Pts',(4.85068927007173,-94.4189842542419,-8.40164026752836));
#33312=CARTESIAN_POINT('Ctrl Pts',(-1.51301075899711E-11,-94.2439842542419,
-8.40164026751963));
#33313=CARTESIAN_POINT('Ctrl Pts',(-4.85068927010199,-94.0689842542419,
-8.4016402675109));
#33314=CARTESIAN_POINT('Ctrl Pts',(-7.27603390513785,-93.8939842542419,
-4.20082013374671));
#33315=CARTESIAN_POINT('Ctrl Pts',(-9.70137854017372,-93.7189842542419,
1.74701493417668E-11));
#33316=CARTESIAN_POINT('Ctrl Pts',(-7.27603390512272,-93.5439842542419,
4.20082013377292));
#33317=CARTESIAN_POINT('Ctrl Pts',(-4.85068927007173,-93.3689842542419,
8.40164026752836));
#33318=CARTESIAN_POINT('Ctrl Pts',(1.5129078685785E-11,-93.1939842542419,
8.40164026751963));
#33319=CARTESIAN_POINT('Ctrl Pts',(4.85068927010198,-93.0189842542419,8.4016402675109));
#33320=CARTESIAN_POINT('Ctrl Pts',(7.27603390513785,-92.8439842542419,4.20082013374672));
#33321=CARTESIAN_POINT('Ctrl Pts',(9.70137854017372,-92.6689842542419,-1.74689612655491E-11));
#33322=CARTESIAN_POINT('Ctrl Pts',(7.27603390512273,-92.4939842542419,-4.20082013377291));
#33323=CARTESIAN_POINT('Ctrl Pts',(4.85068927007173,-92.3189842542419,-8.40164026752836));
#33324=CARTESIAN_POINT('Ctrl Pts',(-1.51301075899711E-11,-92.1439842542419,
-8.40164026751963));
#33325=CARTESIAN_POINT('Ctrl Pts',(-4.85068927010199,-91.9689842542419,
-8.4016402675109));
#33326=CARTESIAN_POINT('Ctrl Pts',(-7.27603390513785,-91.7939842542419,
-4.20082013374671));
#33327=CARTESIAN_POINT('Ctrl Pts',(-9.70137854017372,-91.6189842542419,
1.74701493417668E-11));
#33328=CARTESIAN_POINT('Ctrl Pts',(-7.27603390512272,-91.4439842542419,
4.20082013377292));
#33329=CARTESIAN_POINT('Ctrl Pts',(-4.85068927007173,-91.2689842542419,
8.40164026752836));
#33330=CARTESIAN_POINT('Ctrl Pts',(1.5129078685785E-11,-91.0939842542419,
8.40164026751963));
#33331=CARTESIAN_POINT('Ctrl Pts',(4.85068927010198,-90.9189842542419,8.4016402675109));
#33332=CARTESIAN_POINT('Ctrl Pts',(7.27603390513785,-90.7439842542419,4.20082013374672));
#33333=CARTESIAN_POINT('Ctrl Pts',(9.70137854017372,-90.5689842542419,-1.74689612655491E-11));
#33334=CARTESIAN_POINT('Ctrl Pts',(7.27603390512273,-90.3939842542419,-4.20082013377291));
#33335=CARTESIAN_POINT('Ctrl Pts',(4.85068927007173,-90.2189842542419,-8.40164026752836));
#33336=CARTESIAN_POINT('Ctrl Pts',(-1.51301075899711E-11,-90.0439842542419,
-8.40164026751963));
#33337=CARTESIAN_POINT('Ctrl Pts',(-4.85068927010199,-89.8689842542419,
-8.4016402675109));
#33338=CARTESIAN_POINT('Ctrl Pts',(-7.27603390513785,-89.6939842542419,
-4.20082013374671));
#33339=CARTESIAN_POINT('Ctrl Pts',(-9.70137854017372,-89.5189842542419,
1.74701493417668E-11));
#33340=CARTESIAN_POINT('Ctrl Pts',(-7.27603390512272,-89.3439842542419,
4.20082013377292));
#33341=CARTESIAN_POINT('Ctrl Pts',(-4.85068927007173,-89.1689842542419,
8.40164026752836));
#33342=CARTESIAN_POINT('Ctrl Pts',(1.5129078685785E-11,-88.9939842542419,
8.40164026751963));
#33343=CARTESIAN_POINT('Ctrl Pts',(4.85068927010198,-88.8189842542419,8.4016402675109));
#33344=CARTESIAN_POINT('Ctrl Pts',(7.27603390513785,-88.6439842542419,4.20082013374672));
#33345=CARTESIAN_POINT('Ctrl Pts',(9.70137854017372,-88.4689842542419,-1.74689612655491E-11));
#33346=CARTESIAN_POINT('Ctrl Pts',(7.27603390512273,-88.2939842542419,-4.20082013377291));
#33347=CARTESIAN_POINT('Ctrl Pts',(4.85068927007173,-88.1189842542419,-8.40164026752836));
#33348=CARTESIAN_POINT('Ctrl Pts',(-1.51301075899711E-11,-87.9439842542419,
-8.40164026751963));
#33349=CARTESIAN_POINT('Ctrl Pts',(-4.85068927010199,-87.7689842542419,
-8.4016402675109));
#33350=CARTESIAN_POINT('Ctrl Pts',(-7.27603390513785,-87.5939842542419,
-4.20082013374671));
#33351=CARTESIAN_POINT('Ctrl Pts',(-9.70137854017372,-87.4189842542419,
1.74701493417668E-11));
#33352=CARTESIAN_POINT('Ctrl Pts',(-7.27603390512272,-87.2439842542419,
4.20082013377292));
#33353=CARTESIAN_POINT('Ctrl Pts',(-4.85068927007173,-87.0689842542419,
8.40164026752836));
#33354=CARTESIAN_POINT('Ctrl Pts',(1.5129078685785E-11,-86.8939842542419,
8.40164026751963));
#33355=CARTESIAN_POINT('Ctrl Pts',(4.85068927010198,-86.7189842542419,8.4016402675109));
#33356=CARTESIAN_POINT('Ctrl Pts',(7.27603390513785,-86.5439842542419,4.20082013374672));
#33357=CARTESIAN_POINT('Ctrl Pts',(9.70137854017372,-86.3689842542419,-1.74689612655491E-11));
#33358=CARTESIAN_POINT('Ctrl Pts',(7.27603390512273,-86.1939842542419,-4.20082013377291));
#33359=CARTESIAN_POINT('Ctrl Pts',(4.85068927007173,-86.0189842542419,-8.40164026752836));
#33360=CARTESIAN_POINT('Ctrl Pts',(-1.51301075899711E-11,-85.8439842542419,
-8.40164026751963));
#33361=CARTESIAN_POINT('Ctrl Pts',(-4.85068927010199,-85.6689842542419,
-8.4016402675109));
#33362=CARTESIAN_POINT('Ctrl Pts',(-7.27603390513785,-85.4939842542419,
-4.20082013374671));
#33363=CARTESIAN_POINT('Ctrl Pts',(-9.70137854017372,-85.3189842542419,
1.74701493417668E-11));
#33364=CARTESIAN_POINT('Ctrl Pts',(-7.27603390512272,-85.143984254242,4.20082013377292));
#33365=CARTESIAN_POINT('Ctrl Pts',(-4.85068927007173,-84.9689842542419,
8.40164026752836));
#33366=CARTESIAN_POINT('Ctrl Pts',(1.5129078685785E-11,-84.7939842542419,
8.40164026751963));
#33367=CARTESIAN_POINT('Ctrl Pts',(4.85068927010198,-84.6189842542419,8.4016402675109));
#33368=CARTESIAN_POINT('Ctrl Pts',(7.27603390513785,-84.443984254242,4.20082013374672));
#33369=CARTESIAN_POINT('Ctrl Pts',(9.70137854017372,-84.2689842542419,-1.74689612655491E-11));
#33370=CARTESIAN_POINT('Ctrl Pts',(7.27603390512273,-84.0939842542419,-4.20082013377291));
#33371=CARTESIAN_POINT('Ctrl Pts',(4.85068927007173,-83.9189842542419,-8.40164026752836));
#33372=CARTESIAN_POINT('Ctrl Pts',(-1.51301075899711E-11,-83.7439842542419,
-8.40164026751963));
#33373=CARTESIAN_POINT('Ctrl Pts',(-4.85068927010199,-83.5689842542419,
-8.4016402675109));
#33374=CARTESIAN_POINT('Ctrl Pts',(-7.27603390513785,-83.3939842542419,
-4.20082013374671));
#33375=CARTESIAN_POINT('Ctrl Pts',(-9.70137854017372,-83.2189842542419,
1.74701493417668E-11));
#33376=CARTESIAN_POINT('Ctrl Pts',(-7.27603390512272,-83.0439842542419,
4.20082013377292));
#33377=CARTESIAN_POINT('Ctrl Pts',(-4.85068927007173,-82.868984254242,8.40164026752836));
#33378=CARTESIAN_POINT('Ctrl Pts',(1.5129078685785E-11,-82.6939842542419,
8.40164026751963));
#33379=CARTESIAN_POINT('Ctrl Pts',(4.85068927010198,-82.5189842542419,8.4016402675109));
#33380=CARTESIAN_POINT('Ctrl Pts',(7.27603390513785,-82.3439842542419,4.20082013374672));
#33381=CARTESIAN_POINT('Ctrl Pts',(9.70137854017372,-82.1689842542419,-1.74689612655491E-11));
#33382=CARTESIAN_POINT('Ctrl Pts',(7.27603390512273,-81.993984254242,-4.20082013377291));
#33383=CARTESIAN_POINT('Ctrl Pts',(4.85068927007173,-81.8189842542419,-8.40164026752836));
#33384=CARTESIAN_POINT('Ctrl Pts',(-1.51301075899711E-11,-81.6439842542419,
-8.40164026751963));
#33385=CARTESIAN_POINT('Ctrl Pts',(-4.85068927010199,-81.4689842542419,
-8.4016402675109));
#33386=CARTESIAN_POINT('Ctrl Pts',(-7.27603390513785,-81.293984254242,-4.20082013374671));
#33387=CARTESIAN_POINT('Ctrl Pts',(-9.70137854017372,-81.1189842542419,
1.74701493417668E-11));
#33388=CARTESIAN_POINT('Ctrl Pts',(-7.27603390512272,-80.9439842542419,
4.20082013377292));
#33389=CARTESIAN_POINT('Ctrl Pts',(-4.85068927007173,-80.768984254242,8.40164026752836));
#33390=CARTESIAN_POINT('Ctrl Pts',(1.5129078685785E-11,-80.5939842542419,
8.40164026751963));
#33391=CARTESIAN_POINT('Ctrl Pts',(4.85068927010198,-80.4189842542419,8.4016402675109));
#33392=CARTESIAN_POINT('Ctrl Pts',(7.27603390513785,-80.243984254242,4.20082013374672));
#33393=CARTESIAN_POINT('Ctrl Pts',(9.70137854017372,-80.068984254242,-1.74689612655491E-11));
#33394=CARTESIAN_POINT('Ctrl Pts',(7.27603390512273,-79.8939842542419,-4.20082013377291));
#33395=CARTESIAN_POINT('Ctrl Pts',(4.85068927007173,-79.7189842542419,-8.40164026752836));
#33396=CARTESIAN_POINT('Ctrl Pts',(-1.51301075899711E-11,-79.5439842542419,
-8.40164026751963));
#33397=CARTESIAN_POINT('Ctrl Pts',(-4.85068927010199,-79.368984254242,-8.4016402675109));
#33398=CARTESIAN_POINT('Ctrl Pts',(-7.27603390513785,-79.193984254242,-4.20082013374671));
#33399=CARTESIAN_POINT('Ctrl Pts',(-9.70137854017372,-79.0189842542419,
1.74701493417668E-11));
#33400=CARTESIAN_POINT('Ctrl Pts',(-7.27603390512272,-78.8439842542419,
4.20082013377292));
#33401=CARTESIAN_POINT('Ctrl Pts',(-4.85068927007173,-78.668984254242,8.40164026752836));
#33402=CARTESIAN_POINT('Ctrl Pts',(1.5129078685785E-11,-78.493984254242,
8.40164026751963));
#33403=CARTESIAN_POINT('Ctrl Pts',(4.85068927010198,-78.3189842542419,8.4016402675109));
#33404=CARTESIAN_POINT('Ctrl Pts',(7.27603390513785,-78.143984254242,4.20082013374672));
#33405=CARTESIAN_POINT('Ctrl Pts',(9.70137854017372,-77.968984254242,-1.74689612655491E-11));
#33406=CARTESIAN_POINT('Ctrl Pts',(7.27603390512273,-77.7939842542419,-4.20082013377291));
#33407=CARTESIAN_POINT('Ctrl Pts',(4.85068927007173,-77.618984254242,-8.40164026752836));
#33408=CARTESIAN_POINT('Ctrl Pts',(-1.51301075899711E-11,-77.443984254242,
-8.40164026751963));
#33409=CARTESIAN_POINT('Ctrl Pts',(-4.85068927010199,-77.268984254242,-8.4016402675109));
#33410=CARTESIAN_POINT('Ctrl Pts',(-7.27603390513785,-77.0939842542419,
-4.20082013374671));
#33411=CARTESIAN_POINT('Ctrl Pts',(-9.70137854017372,-76.918984254242,1.74701493417668E-11));
#33412=CARTESIAN_POINT('Ctrl Pts',(-7.27603390512272,-76.743984254242,4.20082013377292));
#33413=CARTESIAN_POINT('Ctrl Pts',(-4.85068927007173,-76.5689842542419,
8.40164026752836));
#33414=CARTESIAN_POINT('Ctrl Pts',(1.5129078685785E-11,-76.393984254242,
8.40164026751963));
#33415=CARTESIAN_POINT('Ctrl Pts',(4.85068927010198,-76.218984254242,8.4016402675109));
#33416=CARTESIAN_POINT('Ctrl Pts',(7.27603390513785,-76.0439842542419,4.20082013374672));
#33417=CARTESIAN_POINT('Ctrl Pts',(9.70137854017372,-75.868984254242,-1.74689612655491E-11));
#33418=CARTESIAN_POINT('Ctrl Pts',(7.27603390512273,-75.693984254242,-4.20082013377291));
#33419=CARTESIAN_POINT('Ctrl Pts',(4.85068927007173,-75.518984254242,-8.40164026752836));
#33420=CARTESIAN_POINT('Ctrl Pts',(-1.51301075899711E-11,-75.343984254242,
-8.40164026751963));
#33421=CARTESIAN_POINT('Ctrl Pts',(-4.85068927010199,-75.1689842542419,
-8.4016402675109));
#33422=CARTESIAN_POINT('Ctrl Pts',(-7.27603390513785,-74.993984254242,-4.20082013374671));
#33423=CARTESIAN_POINT('Ctrl Pts',(-9.70137854017372,-74.818984254242,1.74701493417668E-11));
#33424=CARTESIAN_POINT('Ctrl Pts',(-7.27603390512272,-74.643984254242,4.20082013377292));
#33425=CARTESIAN_POINT('Ctrl Pts',(-4.85068927007173,-74.4689842542419,
8.40164026752836));
#33426=CARTESIAN_POINT('Ctrl Pts',(1.5129078685785E-11,-74.293984254242,
8.40164026751963));
#33427=CARTESIAN_POINT('Ctrl Pts',(4.85068927010198,-74.118984254242,8.4016402675109));
#33428=CARTESIAN_POINT('Ctrl Pts',(7.27603390513785,-73.943984254242,4.20082013374672));
#33429=CARTESIAN_POINT('Ctrl Pts',(9.70137854017372,-73.768984254242,-1.74689612655491E-11));
#33430=CARTESIAN_POINT('Ctrl Pts',(7.27603390512273,-73.593984254242,-4.20082013377291));
#33431=CARTESIAN_POINT('Ctrl Pts',(4.85068927007173,-73.4189842542419,-8.40164026752836));
#33432=CARTESIAN_POINT('Ctrl Pts',(-1.51301075899711E-11,-73.243984254242,
-8.40164026751963));
#33433=CARTESIAN_POINT('Ctrl Pts',(-4.85068927010199,-73.068984254242,-8.4016402675109));
#33434=CARTESIAN_POINT('Ctrl Pts',(-7.27603390513785,-72.893984254242,-4.20082013374671));
#33435=CARTESIAN_POINT('Ctrl Pts',(-9.70137854017372,-72.718984254242,1.74701493417668E-11));
#33436=CARTESIAN_POINT('Ctrl Pts',(-7.27603390512272,-72.543984254242,4.20082013377292));
#33437=CARTESIAN_POINT('Ctrl Pts',(-4.85068927007173,-72.368984254242,8.40164026752836));
#33438=CARTESIAN_POINT('Ctrl Pts',(1.5129078685785E-11,-72.193984254242,
8.40164026751963));
#33439=CARTESIAN_POINT('Ctrl Pts',(4.85068927010198,-72.018984254242,8.4016402675109));
#33440=CARTESIAN_POINT('Ctrl Pts',(7.27603390513785,-71.843984254242,4.20082013374672));
#33441=CARTESIAN_POINT('Ctrl Pts',(9.70137854017372,-71.6689842542419,-1.74689612655491E-11));
#33442=CARTESIAN_POINT('Ctrl Pts',(7.27603390512273,-71.493984254242,-4.20082013377291));
#33443=CARTESIAN_POINT('Ctrl Pts',(4.85068927007173,-71.318984254242,-8.40164026752836));
#33444=CARTESIAN_POINT('Ctrl Pts',(-1.51301075899711E-11,-71.143984254242,
-8.40164026751963));
#33445=CARTESIAN_POINT('Ctrl Pts',(-4.85068927010199,-70.968984254242,-8.4016402675109));
#33446=CARTESIAN_POINT('Ctrl Pts',(-7.27603390513785,-70.793984254242,-4.20082013374671));
#33447=CARTESIAN_POINT('Ctrl Pts',(-9.70137854017372,-70.618984254242,1.74701493417668E-11));
#33448=CARTESIAN_POINT('Ctrl Pts',(-7.27603390512272,-70.443984254242,4.20082013377292));
#33449=CARTESIAN_POINT('Ctrl Pts',(-4.85068927007173,-70.268984254242,8.40164026752836));
#33450=CARTESIAN_POINT('Ctrl Pts',(1.5129078685785E-11,-70.093984254242,
8.40164026751963));
#33451=CARTESIAN_POINT('Ctrl Pts',(4.85068927010198,-69.918984254242,8.4016402675109));
#33452=CARTESIAN_POINT('Ctrl Pts',(7.27603390513785,-69.743984254242,4.20082013374672));
#33453=CARTESIAN_POINT('Ctrl Pts',(9.70137854017372,-69.568984254242,-1.74689612655491E-11));
#33454=CARTESIAN_POINT('Ctrl Pts',(7.27603390512273,-69.393984254242,-4.20082013377291));
#33455=CARTESIAN_POINT('Ctrl Pts',(4.85068927007173,-69.218984254242,-8.40164026752836));
#33456=CARTESIAN_POINT('Ctrl Pts',(-1.51301075899711E-11,-69.043984254242,
-8.40164026751963));
#33457=CARTESIAN_POINT('Ctrl Pts',(-4.85068927010199,-68.868984254242,-8.4016402675109));
#33458=CARTESIAN_POINT('Ctrl Pts',(-7.27603390513785,-68.693984254242,-4.20082013374671));
#33459=CARTESIAN_POINT('Ctrl Pts',(-9.70137854017372,-68.518984254242,1.74701493417668E-11));
#33460=CARTESIAN_POINT('Ctrl Pts',(-7.27603390512272,-68.343984254242,4.20082013377292));
#33461=CARTESIAN_POINT('Ctrl Pts',(-4.85068927007173,-68.168984254242,8.40164026752836));
#33462=CARTESIAN_POINT('Ctrl Pts',(1.5129078685785E-11,-67.993984254242,
8.40164026751963));
#33463=CARTESIAN_POINT('Ctrl Pts',(4.85068927010198,-67.818984254242,8.4016402675109));
#33464=CARTESIAN_POINT('Ctrl Pts',(7.27603390513785,-67.643984254242,4.20082013374672));
#33465=CARTESIAN_POINT('Ctrl Pts',(9.70137854017372,-67.468984254242,-1.74689612655491E-11));
#33466=CARTESIAN_POINT('Ctrl Pts',(7.27603390512273,-67.293984254242,-4.20082013377291));
#33467=CARTESIAN_POINT('Ctrl Pts',(4.85068927007173,-67.118984254242,-8.40164026752836));
#33468=CARTESIAN_POINT('Ctrl Pts',(-1.51301075899711E-11,-66.943984254242,
-8.40164026751963));
#33469=CARTESIAN_POINT('Ctrl Pts',(-4.85068927010199,-66.768984254242,-8.4016402675109));
#33470=CARTESIAN_POINT('Ctrl Pts',(-7.27603390513785,-66.593984254242,-4.20082013374671));
#33471=CARTESIAN_POINT('Ctrl Pts',(-9.70137854017372,-66.418984254242,1.74701493417668E-11));
#33472=CARTESIAN_POINT('Ctrl Pts',(-7.27603390512272,-66.243984254242,4.20082013377292));
#33473=CARTESIAN_POINT('Ctrl Pts',(-4.85068927007173,-66.068984254242,8.40164026752836));
#33474=CARTESIAN_POINT('Ctrl Pts',(1.5129078685785E-11,-65.893984254242,
8.40164026751963));
#33475=CARTESIAN_POINT('Ctrl Pts',(4.85068927010198,-65.718984254242,8.4016402675109));
#33476=CARTESIAN_POINT('Ctrl Pts',(7.27603390513785,-65.543984254242,4.20082013374672));
#33477=CARTESIAN_POINT('Ctrl Pts',(9.70137854017372,-65.368984254242,-1.74689612655491E-11));
#33478=CARTESIAN_POINT('Ctrl Pts',(7.27603390512273,-65.193984254242,-4.20082013377291));
#33479=CARTESIAN_POINT('Ctrl Pts',(4.85068927007173,-65.018984254242,-8.40164026752836));
#33480=CARTESIAN_POINT('Ctrl Pts',(-1.51301075899711E-11,-64.843984254242,
-8.40164026751963));
#33481=CARTESIAN_POINT('Ctrl Pts',(-4.85068927010199,-64.668984254242,-8.4016402675109));
#33482=CARTESIAN_POINT('Ctrl Pts',(-7.27603390513785,-64.493984254242,-4.20082013374671));
#33483=CARTESIAN_POINT('Ctrl Pts',(-9.70137854017372,-64.318984254242,1.74701493417668E-11));
#33484=CARTESIAN_POINT('Ctrl Pts',(-7.27603390512272,-64.143984254242,4.20082013377292));
#33485=CARTESIAN_POINT('Ctrl Pts',(-4.85068927007173,-63.968984254242,8.40164026752836));
#33486=CARTESIAN_POINT('Ctrl Pts',(1.5129078685785E-11,-63.793984254242,
8.40164026751963));
#33487=CARTESIAN_POINT('Ctrl Pts',(4.85068927010198,-63.618984254242,8.4016402675109));
#33488=CARTESIAN_POINT('Ctrl Pts',(7.27603390513785,-63.443984254242,4.20082013374672));
#33489=CARTESIAN_POINT('Ctrl Pts',(9.70137854017372,-63.268984254242,-1.74689612655491E-11));
#33490=CARTESIAN_POINT('Ctrl Pts',(7.27603390512273,-63.093984254242,-4.20082013377291));
#33491=CARTESIAN_POINT('Ctrl Pts',(4.85068927007173,-62.918984254242,-8.40164026752836));
#33492=CARTESIAN_POINT('Ctrl Pts',(-1.51301075899711E-11,-62.743984254242,
-8.40164026751963));
#33493=CARTESIAN_POINT('Ctrl Pts',(-4.85068927010199,-62.568984254242,-8.4016402675109));
#33494=CARTESIAN_POINT('Ctrl Pts',(-7.27603390513785,-62.393984254242,-4.20082013374671));
#33495=CARTESIAN_POINT('Ctrl Pts',(-9.70137854017372,-62.218984254242,1.74701493417668E-11));
#33496=CARTESIAN_POINT('Ctrl Pts',(-7.27603390512272,-62.043984254242,4.20082013377292));
#33497=CARTESIAN_POINT('Ctrl Pts',(-4.85068927007173,-61.868984254242,8.40164026752836));
#33498=CARTESIAN_POINT('Ctrl Pts',(1.5129078685785E-11,-61.693984254242,
8.40164026751963));
#33499=CARTESIAN_POINT('Ctrl Pts',(4.85068927010198,-61.518984254242,8.4016402675109));
#33500=CARTESIAN_POINT('Ctrl Pts',(7.27603390513785,-61.343984254242,4.20082013374672));
#33501=CARTESIAN_POINT('Ctrl Pts',(9.70137854017372,-61.168984254242,-1.74689612655491E-11));
#33502=CARTESIAN_POINT('Ctrl Pts',(7.27603390512273,-60.993984254242,-4.20082013377291));
#33503=CARTESIAN_POINT('Ctrl Pts',(4.85068927007173,-60.818984254242,-8.40164026752836));
#33504=CARTESIAN_POINT('Ctrl Pts',(-1.51301075899711E-11,-60.643984254242,
-8.40164026751963));
#33505=CARTESIAN_POINT('Ctrl Pts',(-4.85068927010199,-60.468984254242,-8.4016402675109));
#33506=CARTESIAN_POINT('Ctrl Pts',(-7.27603390513785,-60.293984254242,-4.20082013374671));
#33507=CARTESIAN_POINT('Ctrl Pts',(-9.70137854017372,-60.118984254242,1.74701493417668E-11));
#33508=CARTESIAN_POINT('Ctrl Pts',(-7.27603390512272,-59.943984254242,4.20082013377292));
#33509=CARTESIAN_POINT('Ctrl Pts',(-4.85068927007173,-59.768984254242,8.40164026752836));
#33510=CARTESIAN_POINT('Ctrl Pts',(1.5129078685785E-11,-59.593984254242,
8.40164026751963));
#33511=CARTESIAN_POINT('Ctrl Pts',(4.85068927010198,-59.418984254242,8.4016402675109));
#33512=CARTESIAN_POINT('Ctrl Pts',(7.27603390513785,-59.243984254242,4.20082013374672));
#33513=CARTESIAN_POINT('Ctrl Pts',(9.70137854017372,-59.068984254242,-1.74689612655491E-11));
#33514=CARTESIAN_POINT('Ctrl Pts',(7.27603390512273,-58.893984254242,-4.20082013377291));
#33515=CARTESIAN_POINT('Ctrl Pts',(4.85068927007173,-58.718984254242,-8.40164026752836));
#33516=CARTESIAN_POINT('Ctrl Pts',(-1.51301075899711E-11,-58.543984254242,
-8.40164026751963));
#33517=CARTESIAN_POINT('Ctrl Pts',(-4.85068927010199,-58.368984254242,-8.4016402675109));
#33518=CARTESIAN_POINT('Ctrl Pts',(-7.27603390513785,-58.193984254242,-4.20082013374671));
#33519=CARTESIAN_POINT('Ctrl Pts',(-9.70137854017372,-58.018984254242,1.74701493417668E-11));
#33520=CARTESIAN_POINT('Ctrl Pts',(-7.27603390512272,-57.843984254242,4.20082013377292));
#33521=CARTESIAN_POINT('Ctrl Pts',(-4.85068927007173,-57.668984254242,8.40164026752836));
#33522=CARTESIAN_POINT('Ctrl Pts',(1.5129078685785E-11,-57.493984254242,
8.40164026751963));
#33523=CARTESIAN_POINT('Ctrl Pts',(4.85068927010198,-57.318984254242,8.4016402675109));
#33524=CARTESIAN_POINT('Ctrl Pts',(7.27603390513785,-57.143984254242,4.20082013374672));
#33525=CARTESIAN_POINT('Ctrl Pts',(9.70137854017372,-56.968984254242,-1.74689612655491E-11));
#33526=CARTESIAN_POINT('Ctrl Pts',(7.27603390512273,-56.793984254242,-4.20082013377291));
#33527=CARTESIAN_POINT('Ctrl Pts',(4.85068927007173,-56.618984254242,-8.40164026752836));
#33528=CARTESIAN_POINT('Ctrl Pts',(-1.51301075899711E-11,-56.443984254242,
-8.40164026751963));
#33529=CARTESIAN_POINT('Ctrl Pts',(-4.85068927010199,-56.268984254242,-8.4016402675109));
#33530=CARTESIAN_POINT('Ctrl Pts',(-7.27603390513785,-56.093984254242,-4.20082013374671));
#33531=CARTESIAN_POINT('Ctrl Pts',(-9.70137854017372,-55.918984254242,1.74701493417668E-11));
#33532=CARTESIAN_POINT('Ctrl Pts',(-7.27603390512272,-55.743984254242,4.20082013377292));
#33533=CARTESIAN_POINT('Ctrl Pts',(-4.85068927007173,-55.568984254242,8.40164026752836));
#33534=CARTESIAN_POINT('Ctrl Pts',(1.5129078685785E-11,-55.393984254242,
8.40164026751963));
#33535=CARTESIAN_POINT('Ctrl Pts',(4.85068927010198,-55.218984254242,8.4016402675109));
#33536=CARTESIAN_POINT('Ctrl Pts',(7.27603390513785,-55.043984254242,4.20082013374672));
#33537=CARTESIAN_POINT('Ctrl Pts',(9.70137854017372,-54.868984254242,-1.74689612655491E-11));
#33538=CARTESIAN_POINT('Ctrl Pts',(7.27603390512273,-54.693984254242,-4.20082013377291));
#33539=CARTESIAN_POINT('Ctrl Pts',(4.85068927007173,-54.518984254242,-8.40164026752836));
#33540=CARTESIAN_POINT('Ctrl Pts',(-1.51301075899711E-11,-54.343984254242,
-8.40164026751963));
#33541=CARTESIAN_POINT('Ctrl Pts',(-4.85068927010199,-54.168984254242,-8.4016402675109));
#33542=CARTESIAN_POINT('Ctrl Pts',(-7.27603390513785,-53.993984254242,-4.20082013374671));
#33543=CARTESIAN_POINT('Ctrl Pts',(-9.70137854017372,-53.818984254242,1.74701493417668E-11));
#33544=CARTESIAN_POINT('Ctrl Pts',(-7.27603390512272,-53.643984254242,4.20082013377292));
#33545=CARTESIAN_POINT('Ctrl Pts',(-4.85068927007173,-53.468984254242,8.40164026752836));
#33546=CARTESIAN_POINT('Ctrl Pts',(1.5129078685785E-11,-53.293984254242,
8.40164026751963));
#33547=CARTESIAN_POINT('Ctrl Pts',(4.85068927010198,-53.118984254242,8.4016402675109));
#33548=CARTESIAN_POINT('Ctrl Pts',(7.27603390513785,-52.943984254242,4.20082013374672));
#33549=CARTESIAN_POINT('Ctrl Pts',(9.70137854017372,-52.768984254242,-1.74689612655491E-11));
#33550=CARTESIAN_POINT('Ctrl Pts',(7.27603390512273,-52.593984254242,-4.20082013377291));
#33551=CARTESIAN_POINT('Ctrl Pts',(4.85068927007173,-52.418984254242,-8.40164026752836));
#33552=CARTESIAN_POINT('Ctrl Pts',(-1.51301075899711E-11,-52.243984254242,
-8.40164026751963));
#33553=CARTESIAN_POINT('Ctrl Pts',(-4.85068927010199,-52.068984254242,-8.4016402675109));
#33554=CARTESIAN_POINT('Ctrl Pts',(-7.27603390513785,-51.893984254242,-4.20082013374671));
#33555=CARTESIAN_POINT('Ctrl Pts',(-9.70137854017372,-51.718984254242,1.74701493417668E-11));
#33556=CARTESIAN_POINT('Ctrl Pts',(-7.27603390512272,-51.543984254242,4.20082013377292));
#33557=CARTESIAN_POINT('Ctrl Pts',(-4.85068927007173,-51.368984254242,8.40164026752836));
#33558=CARTESIAN_POINT('Ctrl Pts',(1.5129078685785E-11,-51.193984254242,
8.40164026751963));
#33559=CARTESIAN_POINT('Ctrl Pts',(4.85068927010198,-51.018984254242,8.4016402675109));
#33560=CARTESIAN_POINT('Ctrl Pts',(7.27603390513785,-50.843984254242,4.20082013374672));
#33561=CARTESIAN_POINT('Ctrl Pts',(9.70137854017372,-50.668984254242,-1.74689612655491E-11));
#33562=CARTESIAN_POINT('Ctrl Pts',(7.27603390512273,-50.493984254242,-4.20082013377291));
#33563=CARTESIAN_POINT('Ctrl Pts',(4.85068927007173,-50.318984254242,-8.40164026752836));
#33564=CARTESIAN_POINT('Ctrl Pts',(-1.51301075899711E-11,-50.143984254242,
-8.40164026751963));
#33565=CARTESIAN_POINT('Ctrl Pts',(-4.85068927010199,-49.968984254242,-8.4016402675109));
#33566=CARTESIAN_POINT('Ctrl Pts',(-7.27603390513785,-49.793984254242,-4.20082013374671));
#33567=CARTESIAN_POINT('Ctrl Pts',(-9.70137854017372,-49.618984254242,1.74701493417668E-11));
#33568=CARTESIAN_POINT('Ctrl Pts',(-7.27603390512272,-49.443984254242,4.20082013377292));
#33569=CARTESIAN_POINT('Ctrl Pts',(-4.85068927007173,-49.268984254242,8.40164026752836));
#33570=CARTESIAN_POINT('Ctrl Pts',(1.5129078685785E-11,-49.093984254242,
8.40164026751963));
#33571=CARTESIAN_POINT('Ctrl Pts',(4.85068927010198,-48.918984254242,8.4016402675109));
#33572=CARTESIAN_POINT('Ctrl Pts',(7.27603390513785,-48.743984254242,4.20082013374672));
#33573=CARTESIAN_POINT('Ctrl Pts',(9.70137854017372,-48.568984254242,-1.74689612655491E-11));
#33574=CARTESIAN_POINT('Ctrl Pts',(7.27603390512273,-48.393984254242,-4.20082013377291));
#33575=CARTESIAN_POINT('Ctrl Pts',(4.85068927007173,-48.218984254242,-8.40164026752836));
#33576=CARTESIAN_POINT('Ctrl Pts',(-1.51301075899711E-11,-48.043984254242,
-8.40164026751963));
#33577=CARTESIAN_POINT('Ctrl Pts',(-4.85068927010199,-47.868984254242,-8.4016402675109));
#33578=CARTESIAN_POINT('Ctrl Pts',(-7.27603390513785,-47.693984254242,-4.20082013374671));
#33579=CARTESIAN_POINT('Ctrl Pts',(-9.70137854017372,-47.518984254242,1.74701493417668E-11));
#33580=CARTESIAN_POINT('Ctrl Pts',(-7.27603390512272,-47.343984254242,4.20082013377292));
#33581=CARTESIAN_POINT('Ctrl Pts',(-4.85068927007173,-47.168984254242,8.40164026752836));
#33582=CARTESIAN_POINT('Ctrl Pts',(1.5129078685785E-11,-46.993984254242,
8.40164026751963));
#33583=CARTESIAN_POINT('Ctrl Pts',(4.85068927010198,-46.818984254242,8.4016402675109));
#33584=CARTESIAN_POINT('Ctrl Pts',(7.27603390513785,-46.643984254242,4.20082013374672));
#33585=CARTESIAN_POINT('Ctrl Pts',(9.70137854017372,-46.468984254242,-1.74689612655491E-11));
#33586=CARTESIAN_POINT('Ctrl Pts',(7.27603390512273,-46.293984254242,-4.20082013377291));
#33587=CARTESIAN_POINT('Ctrl Pts',(4.85068927007173,-46.118984254242,-8.40164026752836));
#33588=CARTESIAN_POINT('Ctrl Pts',(-1.51301075899711E-11,-45.943984254242,
-8.40164026751963));
#33589=CARTESIAN_POINT('Ctrl Pts',(-4.85068927010199,-45.768984254242,-8.4016402675109));
#33590=CARTESIAN_POINT('Ctrl Pts',(-7.27603390513785,-45.593984254242,-4.20082013374671));
#33591=CARTESIAN_POINT('Ctrl Pts',(-9.70137854017372,-45.418984254242,1.74701493417668E-11));
#33592=CARTESIAN_POINT('Ctrl Pts',(-7.27603390512272,-45.243984254242,4.20082013377292));
#33593=CARTESIAN_POINT('Ctrl Pts',(-4.85068927007173,-45.068984254242,8.40164026752836));
#33594=CARTESIAN_POINT('Ctrl Pts',(1.5129078685785E-11,-44.893984254242,
8.40164026751963));
#33595=CARTESIAN_POINT('Ctrl Pts',(4.85068927010198,-44.718984254242,8.4016402675109));
#33596=CARTESIAN_POINT('Ctrl Pts',(7.27603390513785,-44.543984254242,4.20082013374672));
#33597=CARTESIAN_POINT('Ctrl Pts',(9.70137854017372,-44.368984254242,-1.74689612655491E-11));
#33598=CARTESIAN_POINT('Ctrl Pts',(7.27603390512273,-44.193984254242,-4.20082013377291));
#33599=CARTESIAN_POINT('Ctrl Pts',(4.85068927007173,-44.018984254242,-8.40164026752836));
#33600=CARTESIAN_POINT('Ctrl Pts',(-1.51301075899711E-11,-43.843984254242,
-8.40164026751963));
#33601=CARTESIAN_POINT('Ctrl Pts',(-1.4702867290402E-11,-213.820483118095,
-8.16439679232146));
#33602=CARTESIAN_POINT('Ctrl Pts',(-4.71371668583241,-213.645483118095,
-8.16439679231297));
#33603=CARTESIAN_POINT('Ctrl Pts',(-7.07057502873392,-213.470483118095,
-4.082198396148));
#33604=CARTESIAN_POINT('Ctrl Pts',(-9.42743337163542,-213.295483118095,
1.69768315121407E-11));
#33605=CARTESIAN_POINT('Ctrl Pts',(-7.07057502871922,-213.120483118095,
4.08219839617346));
#33606=CARTESIAN_POINT('Ctrl Pts',(-4.71371668580301,-212.945483118095,
8.16439679232994));
#33607=CARTESIAN_POINT('Ctrl Pts',(1.47018674401621E-11,-212.770483118095,
8.16439679232146));
#33608=CARTESIAN_POINT('Ctrl Pts',(4.71371668583241,-212.595483118095,8.16439679231297));
#33609=CARTESIAN_POINT('Ctrl Pts',(7.07057502873392,-212.420483118095,4.082198396148));
#33610=CARTESIAN_POINT('Ctrl Pts',(9.42743337163542,-212.245483118095,-1.69756769845304E-11));
#33611=CARTESIAN_POINT('Ctrl Pts',(7.07057502871922,-212.070483118095,-4.08219839617346));
#33612=CARTESIAN_POINT('Ctrl Pts',(4.71371668580301,-211.895483118095,-8.16439679232994));
#33613=CARTESIAN_POINT('Ctrl Pts',(-1.4702867290402E-11,-211.720483118095,
-8.16439679232146));
#33614=CARTESIAN_POINT('Ctrl Pts',(-4.71371668583241,-211.545483118095,
-8.16439679231297));
#33615=CARTESIAN_POINT('Ctrl Pts',(-7.07057502873392,-211.370483118095,
-4.082198396148));
#33616=CARTESIAN_POINT('Ctrl Pts',(-9.42743337163542,-211.195483118095,
1.69768315121407E-11));
#33617=CARTESIAN_POINT('Ctrl Pts',(-7.07057502871922,-211.020483118095,
4.08219839617346));
#33618=CARTESIAN_POINT('Ctrl Pts',(-4.71371668580301,-210.845483118095,
8.16439679232994));
#33619=CARTESIAN_POINT('Ctrl Pts',(1.47018674401621E-11,-210.670483118095,
8.16439679232146));
#33620=CARTESIAN_POINT('Ctrl Pts',(4.71371668583241,-210.495483118095,8.16439679231297));
#33621=CARTESIAN_POINT('Ctrl Pts',(7.07057502873392,-210.320483118095,4.082198396148));
#33622=CARTESIAN_POINT('Ctrl Pts',(9.42743337163542,-210.145483118095,-1.69756769845304E-11));
#33623=CARTESIAN_POINT('Ctrl Pts',(7.07057502871922,-209.970483118095,-4.08219839617346));
#33624=CARTESIAN_POINT('Ctrl Pts',(4.71371668580301,-209.795483118095,-8.16439679232994));
#33625=CARTESIAN_POINT('Ctrl Pts',(-1.4702867290402E-11,-209.620483118095,
-8.16439679232146));
#33626=CARTESIAN_POINT('Ctrl Pts',(-4.71371668583241,-209.445483118095,
-8.16439679231297));
#33627=CARTESIAN_POINT('Ctrl Pts',(-7.07057502873392,-209.270483118095,
-4.082198396148));
#33628=CARTESIAN_POINT('Ctrl Pts',(-9.42743337163542,-209.095483118095,
1.69768315121407E-11));
#33629=CARTESIAN_POINT('Ctrl Pts',(-7.07057502871922,-208.920483118095,
4.08219839617346));
#33630=CARTESIAN_POINT('Ctrl Pts',(-4.71371668580301,-208.745483118095,
8.16439679232994));
#33631=CARTESIAN_POINT('Ctrl Pts',(1.47018674401621E-11,-208.570483118095,
8.16439679232146));
#33632=CARTESIAN_POINT('Ctrl Pts',(4.71371668583241,-208.395483118095,8.16439679231297));
#33633=CARTESIAN_POINT('Ctrl Pts',(7.07057502873392,-208.220483118095,4.082198396148));
#33634=CARTESIAN_POINT('Ctrl Pts',(9.42743337163542,-208.045483118095,-1.69756769845304E-11));
#33635=CARTESIAN_POINT('Ctrl Pts',(7.07057502871922,-207.870483118095,-4.08219839617346));
#33636=CARTESIAN_POINT('Ctrl Pts',(4.71371668580301,-207.695483118095,-8.16439679232994));
#33637=CARTESIAN_POINT('Ctrl Pts',(-1.4702867290402E-11,-207.520483118095,
-8.16439679232146));
#33638=CARTESIAN_POINT('Ctrl Pts',(-4.71371668583241,-207.345483118095,
-8.16439679231297));
#33639=CARTESIAN_POINT('Ctrl Pts',(-7.07057502873392,-207.170483118095,
-4.082198396148));
#33640=CARTESIAN_POINT('Ctrl Pts',(-9.42743337163542,-206.995483118095,
1.69768315121407E-11));
#33641=CARTESIAN_POINT('Ctrl Pts',(-7.07057502871922,-206.820483118095,
4.08219839617346));
#33642=CARTESIAN_POINT('Ctrl Pts',(-4.71371668580301,-206.645483118095,
8.16439679232994));
#33643=CARTESIAN_POINT('Ctrl Pts',(1.47018674401621E-11,-206.470483118095,
8.16439679232146));
#33644=CARTESIAN_POINT('Ctrl Pts',(4.71371668583241,-206.295483118095,8.16439679231297));
#33645=CARTESIAN_POINT('Ctrl Pts',(7.07057502873392,-206.120483118095,4.082198396148));
#33646=CARTESIAN_POINT('Ctrl Pts',(9.42743337163542,-205.945483118095,-1.69756769845304E-11));
#33647=CARTESIAN_POINT('Ctrl Pts',(7.07057502871922,-205.770483118095,-4.08219839617346));
#33648=CARTESIAN_POINT('Ctrl Pts',(4.71371668580301,-205.595483118095,-8.16439679232994));
#33649=CARTESIAN_POINT('Ctrl Pts',(-1.4702867290402E-11,-205.420483118095,
-8.16439679232146));
#33650=CARTESIAN_POINT('Ctrl Pts',(-4.71371668583241,-205.245483118095,
-8.16439679231297));
#33651=CARTESIAN_POINT('Ctrl Pts',(-7.07057502873392,-205.070483118095,
-4.082198396148));
#33652=CARTESIAN_POINT('Ctrl Pts',(-9.42743337163542,-204.895483118095,
1.69768315121407E-11));
#33653=CARTESIAN_POINT('Ctrl Pts',(-7.07057502871922,-204.720483118095,
4.08219839617346));
#33654=CARTESIAN_POINT('Ctrl Pts',(-4.71371668580301,-204.545483118095,
8.16439679232994));
#33655=CARTESIAN_POINT('Ctrl Pts',(1.47018674401621E-11,-204.370483118095,
8.16439679232146));
#33656=CARTESIAN_POINT('Ctrl Pts',(4.71371668583241,-204.195483118095,8.16439679231297));
#33657=CARTESIAN_POINT('Ctrl Pts',(7.07057502873392,-204.020483118095,4.082198396148));
#33658=CARTESIAN_POINT('Ctrl Pts',(9.42743337163542,-203.845483118095,-1.69756769845304E-11));
#33659=CARTESIAN_POINT('Ctrl Pts',(7.07057502871922,-203.670483118095,-4.08219839617346));
#33660=CARTESIAN_POINT('Ctrl Pts',(4.71371668580301,-203.495483118095,-8.16439679232994));
#33661=CARTESIAN_POINT('Ctrl Pts',(-1.4702867290402E-11,-203.320483118095,
-8.16439679232146));
#33662=CARTESIAN_POINT('Ctrl Pts',(-4.71371668583241,-203.145483118095,
-8.16439679231297));
#33663=CARTESIAN_POINT('Ctrl Pts',(-7.07057502873392,-202.970483118095,
-4.082198396148));
#33664=CARTESIAN_POINT('Ctrl Pts',(-9.42743337163542,-202.795483118095,
1.69768315121407E-11));
#33665=CARTESIAN_POINT('Ctrl Pts',(-7.07057502871922,-202.620483118095,
4.08219839617346));
#33666=CARTESIAN_POINT('Ctrl Pts',(-4.71371668580301,-202.445483118095,
8.16439679232994));
#33667=CARTESIAN_POINT('Ctrl Pts',(1.47018674401621E-11,-202.270483118095,
8.16439679232146));
#33668=CARTESIAN_POINT('Ctrl Pts',(4.71371668583241,-202.095483118095,8.16439679231297));
#33669=CARTESIAN_POINT('Ctrl Pts',(7.07057502873392,-201.920483118095,4.082198396148));
#33670=CARTESIAN_POINT('Ctrl Pts',(9.42743337163542,-201.745483118095,-1.69756769845304E-11));
#33671=CARTESIAN_POINT('Ctrl Pts',(7.07057502871922,-201.570483118095,-4.08219839617346));
#33672=CARTESIAN_POINT('Ctrl Pts',(4.71371668580301,-201.395483118095,-8.16439679232994));
#33673=CARTESIAN_POINT('Ctrl Pts',(-1.4702867290402E-11,-201.220483118095,
-8.16439679232146));
#33674=CARTESIAN_POINT('Ctrl Pts',(-4.71371668583241,-201.045483118095,
-8.16439679231297));
#33675=CARTESIAN_POINT('Ctrl Pts',(-7.07057502873392,-200.870483118095,
-4.082198396148));
#33676=CARTESIAN_POINT('Ctrl Pts',(-9.42743337163542,-200.695483118095,
1.69768315121407E-11));
#33677=CARTESIAN_POINT('Ctrl Pts',(-7.07057502871922,-200.520483118095,
4.08219839617346));
#33678=CARTESIAN_POINT('Ctrl Pts',(-4.71371668580301,-200.345483118095,
8.16439679232994));
#33679=CARTESIAN_POINT('Ctrl Pts',(1.47018674401621E-11,-200.170483118095,
8.16439679232146));
#33680=CARTESIAN_POINT('Ctrl Pts',(4.71371668583241,-199.995483118095,8.16439679231297));
#33681=CARTESIAN_POINT('Ctrl Pts',(7.07057502873392,-199.820483118095,4.082198396148));
#33682=CARTESIAN_POINT('Ctrl Pts',(9.42743337163542,-199.645483118095,-1.69756769845304E-11));
#33683=CARTESIAN_POINT('Ctrl Pts',(7.07057502871922,-199.470483118095,-4.08219839617346));
#33684=CARTESIAN_POINT('Ctrl Pts',(4.71371668580301,-199.295483118095,-8.16439679232994));
#33685=CARTESIAN_POINT('Ctrl Pts',(-1.4702867290402E-11,-199.120483118095,
-8.16439679232146));
#33686=CARTESIAN_POINT('Ctrl Pts',(-4.71371668583241,-198.945483118095,
-8.16439679231297));
#33687=CARTESIAN_POINT('Ctrl Pts',(-7.07057502873392,-198.770483118095,
-4.082198396148));
#33688=CARTESIAN_POINT('Ctrl Pts',(-9.42743337163542,-198.595483118095,
1.69768315121407E-11));
#33689=CARTESIAN_POINT('Ctrl Pts',(-7.07057502871922,-198.420483118095,
4.08219839617346));
#33690=CARTESIAN_POINT('Ctrl Pts',(-4.71371668580301,-198.245483118095,
8.16439679232994));
#33691=CARTESIAN_POINT('Ctrl Pts',(1.47018674401621E-11,-198.070483118095,
8.16439679232146));
#33692=CARTESIAN_POINT('Ctrl Pts',(4.71371668583241,-197.895483118095,8.16439679231297));
#33693=CARTESIAN_POINT('Ctrl Pts',(7.07057502873392,-197.720483118095,4.082198396148));
#33694=CARTESIAN_POINT('Ctrl Pts',(9.42743337163542,-197.545483118095,-1.69756769845304E-11));
#33695=CARTESIAN_POINT('Ctrl Pts',(7.07057502871922,-197.370483118095,-4.08219839617346));
#33696=CARTESIAN_POINT('Ctrl Pts',(4.71371668580301,-197.195483118095,-8.16439679232994));
#33697=CARTESIAN_POINT('Ctrl Pts',(-1.4702867290402E-11,-197.020483118095,
-8.16439679232146));
#33698=CARTESIAN_POINT('Ctrl Pts',(-4.71371668583241,-196.845483118095,
-8.16439679231297));
#33699=CARTESIAN_POINT('Ctrl Pts',(-7.07057502873392,-196.670483118095,
-4.082198396148));
#33700=CARTESIAN_POINT('Ctrl Pts',(-9.42743337163542,-196.495483118095,
1.69768315121407E-11));
#33701=CARTESIAN_POINT('Ctrl Pts',(-7.07057502871922,-196.320483118095,
4.08219839617346));
#33702=CARTESIAN_POINT('Ctrl Pts',(-4.71371668580301,-196.145483118095,
8.16439679232994));
#33703=CARTESIAN_POINT('Ctrl Pts',(1.47018674401621E-11,-195.970483118095,
8.16439679232146));
#33704=CARTESIAN_POINT('Ctrl Pts',(4.71371668583241,-195.795483118095,8.16439679231297));
#33705=CARTESIAN_POINT('Ctrl Pts',(7.07057502873392,-195.620483118095,4.082198396148));
#33706=CARTESIAN_POINT('Ctrl Pts',(9.42743337163542,-195.445483118095,-1.69756769845304E-11));
#33707=CARTESIAN_POINT('Ctrl Pts',(7.07057502871922,-195.270483118095,-4.08219839617346));
#33708=CARTESIAN_POINT('Ctrl Pts',(4.71371668580301,-195.095483118095,-8.16439679232994));
#33709=CARTESIAN_POINT('Ctrl Pts',(-1.4702867290402E-11,-194.920483118095,
-8.16439679232146));
#33710=CARTESIAN_POINT('Ctrl Pts',(-4.71371668583241,-194.745483118095,
-8.16439679231297));
#33711=CARTESIAN_POINT('Ctrl Pts',(-7.07057502873392,-194.570483118095,
-4.082198396148));
#33712=CARTESIAN_POINT('Ctrl Pts',(-9.42743337163542,-194.395483118095,
1.69768315121407E-11));
#33713=CARTESIAN_POINT('Ctrl Pts',(-7.07057502871922,-194.220483118095,
4.08219839617346));
#33714=CARTESIAN_POINT('Ctrl Pts',(-4.71371668580301,-194.045483118095,
8.16439679232994));
#33715=CARTESIAN_POINT('Ctrl Pts',(1.47018674401621E-11,-193.870483118095,
8.16439679232146));
#33716=CARTESIAN_POINT('Ctrl Pts',(4.71371668583241,-193.695483118095,8.16439679231297));
#33717=CARTESIAN_POINT('Ctrl Pts',(7.07057502873392,-193.520483118095,4.082198396148));
#33718=CARTESIAN_POINT('Ctrl Pts',(9.42743337163542,-193.345483118095,-1.69756769845304E-11));
#33719=CARTESIAN_POINT('Ctrl Pts',(7.07057502871922,-193.170483118095,-4.08219839617346));
#33720=CARTESIAN_POINT('Ctrl Pts',(4.71371668580301,-192.995483118095,-8.16439679232994));
#33721=CARTESIAN_POINT('Ctrl Pts',(-1.4702867290402E-11,-192.820483118095,
-8.16439679232146));
#33722=CARTESIAN_POINT('Ctrl Pts',(-4.71371668583241,-192.645483118095,
-8.16439679231297));
#33723=CARTESIAN_POINT('Ctrl Pts',(-7.07057502873392,-192.470483118095,
-4.082198396148));
#33724=CARTESIAN_POINT('Ctrl Pts',(-9.42743337163542,-192.295483118095,
1.69768315121407E-11));
#33725=CARTESIAN_POINT('Ctrl Pts',(-7.07057502871922,-192.120483118095,
4.08219839617346));
#33726=CARTESIAN_POINT('Ctrl Pts',(-4.71371668580301,-191.945483118095,
8.16439679232994));
#33727=CARTESIAN_POINT('Ctrl Pts',(1.47018674401621E-11,-191.770483118095,
8.16439679232146));
#33728=CARTESIAN_POINT('Ctrl Pts',(4.71371668583241,-191.595483118095,8.16439679231297));
#33729=CARTESIAN_POINT('Ctrl Pts',(7.07057502873392,-191.420483118095,4.082198396148));
#33730=CARTESIAN_POINT('Ctrl Pts',(9.42743337163542,-191.245483118095,-1.69756769845304E-11));
#33731=CARTESIAN_POINT('Ctrl Pts',(7.07057502871922,-191.070483118095,-4.08219839617346));
#33732=CARTESIAN_POINT('Ctrl Pts',(4.71371668580301,-190.895483118095,-8.16439679232994));
#33733=CARTESIAN_POINT('Ctrl Pts',(-1.4702867290402E-11,-190.720483118095,
-8.16439679232146));
#33734=CARTESIAN_POINT('Ctrl Pts',(-4.71371668583241,-190.545483118095,
-8.16439679231297));
#33735=CARTESIAN_POINT('Ctrl Pts',(-7.07057502873392,-190.370483118095,
-4.082198396148));
#33736=CARTESIAN_POINT('Ctrl Pts',(-9.42743337163542,-190.195483118095,
1.69768315121407E-11));
#33737=CARTESIAN_POINT('Ctrl Pts',(-7.07057502871922,-190.020483118095,
4.08219839617346));
#33738=CARTESIAN_POINT('Ctrl Pts',(-4.71371668580301,-189.845483118095,
8.16439679232994));
#33739=CARTESIAN_POINT('Ctrl Pts',(1.47018674401621E-11,-189.670483118095,
8.16439679232146));
#33740=CARTESIAN_POINT('Ctrl Pts',(4.71371668583241,-189.495483118095,8.16439679231297));
#33741=CARTESIAN_POINT('Ctrl Pts',(7.07057502873392,-189.320483118095,4.082198396148));
#33742=CARTESIAN_POINT('Ctrl Pts',(9.42743337163542,-189.145483118095,-1.69756769845304E-11));
#33743=CARTESIAN_POINT('Ctrl Pts',(7.07057502871922,-188.970483118095,-4.08219839617346));
#33744=CARTESIAN_POINT('Ctrl Pts',(4.71371668580301,-188.795483118095,-8.16439679232994));
#33745=CARTESIAN_POINT('Ctrl Pts',(-1.4702867290402E-11,-188.620483118095,
-8.16439679232146));
#33746=CARTESIAN_POINT('Ctrl Pts',(-4.71371668583241,-188.445483118095,
-8.16439679231297));
#33747=CARTESIAN_POINT('Ctrl Pts',(-7.07057502873392,-188.270483118095,
-4.082198396148));
#33748=CARTESIAN_POINT('Ctrl Pts',(-9.42743337163542,-188.095483118095,
1.69768315121407E-11));
#33749=CARTESIAN_POINT('Ctrl Pts',(-7.07057502871922,-187.920483118095,
4.08219839617346));
#33750=CARTESIAN_POINT('Ctrl Pts',(-4.71371668580301,-187.745483118095,
8.16439679232994));
#33751=CARTESIAN_POINT('Ctrl Pts',(1.47018674401621E-11,-187.570483118095,
8.16439679232146));
#33752=CARTESIAN_POINT('Ctrl Pts',(4.71371668583241,-187.395483118095,8.16439679231297));
#33753=CARTESIAN_POINT('Ctrl Pts',(7.07057502873392,-187.220483118095,4.082198396148));
#33754=CARTESIAN_POINT('Ctrl Pts',(9.42743337163542,-187.045483118095,-1.69756769845304E-11));
#33755=CARTESIAN_POINT('Ctrl Pts',(7.07057502871922,-186.870483118095,-4.08219839617346));
#33756=CARTESIAN_POINT('Ctrl Pts',(4.71371668580301,-186.695483118095,-8.16439679232994));
#33757=CARTESIAN_POINT('Ctrl Pts',(-1.4702867290402E-11,-186.520483118095,
-8.16439679232146));
#33758=CARTESIAN_POINT('Ctrl Pts',(-4.71371668583241,-186.345483118095,
-8.16439679231297));
#33759=CARTESIAN_POINT('Ctrl Pts',(-7.07057502873392,-186.170483118095,
-4.082198396148));
#33760=CARTESIAN_POINT('Ctrl Pts',(-9.42743337163542,-185.995483118095,
1.69768315121407E-11));
#33761=CARTESIAN_POINT('Ctrl Pts',(-7.07057502871922,-185.820483118095,
4.08219839617346));
#33762=CARTESIAN_POINT('Ctrl Pts',(-4.71371668580301,-185.645483118095,
8.16439679232994));
#33763=CARTESIAN_POINT('Ctrl Pts',(1.47018674401621E-11,-185.470483118095,
8.16439679232146));
#33764=CARTESIAN_POINT('Ctrl Pts',(4.71371668583241,-185.295483118095,8.16439679231297));
#33765=CARTESIAN_POINT('Ctrl Pts',(7.07057502873392,-185.120483118095,4.082198396148));
#33766=CARTESIAN_POINT('Ctrl Pts',(9.42743337163542,-184.945483118095,-1.69756769845304E-11));
#33767=CARTESIAN_POINT('Ctrl Pts',(7.07057502871922,-184.770483118095,-4.08219839617346));
#33768=CARTESIAN_POINT('Ctrl Pts',(4.71371668580301,-184.595483118095,-8.16439679232994));
#33769=CARTESIAN_POINT('Ctrl Pts',(-1.4702867290402E-11,-184.420483118095,
-8.16439679232146));
#33770=CARTESIAN_POINT('Ctrl Pts',(-4.71371668583241,-184.245483118095,
-8.16439679231297));
#33771=CARTESIAN_POINT('Ctrl Pts',(-7.07057502873392,-184.070483118095,
-4.082198396148));
#33772=CARTESIAN_POINT('Ctrl Pts',(-9.42743337163542,-183.895483118095,
1.69768315121407E-11));
#33773=CARTESIAN_POINT('Ctrl Pts',(-7.07057502871922,-183.720483118095,
4.08219839617346));
#33774=CARTESIAN_POINT('Ctrl Pts',(-4.71371668580301,-183.545483118095,
8.16439679232994));
#33775=CARTESIAN_POINT('Ctrl Pts',(1.47018674401621E-11,-183.370483118095,
8.16439679232146));
#33776=CARTESIAN_POINT('Ctrl Pts',(4.71371668583241,-183.195483118095,8.16439679231297));
#33777=CARTESIAN_POINT('Ctrl Pts',(7.07057502873392,-183.020483118095,4.082198396148));
#33778=CARTESIAN_POINT('Ctrl Pts',(9.42743337163542,-182.845483118095,-1.69756769845304E-11));
#33779=CARTESIAN_POINT('Ctrl Pts',(7.07057502871922,-182.670483118095,-4.08219839617346));
#33780=CARTESIAN_POINT('Ctrl Pts',(4.71371668580301,-182.495483118095,-8.16439679232994));
#33781=CARTESIAN_POINT('Ctrl Pts',(-1.4702867290402E-11,-182.320483118095,
-8.16439679232146));
#33782=CARTESIAN_POINT('Ctrl Pts',(-4.71371668583241,-182.145483118095,
-8.16439679231297));
#33783=CARTESIAN_POINT('Ctrl Pts',(-7.07057502873392,-181.970483118095,
-4.082198396148));
#33784=CARTESIAN_POINT('Ctrl Pts',(-9.42743337163542,-181.795483118095,
1.69768315121407E-11));
#33785=CARTESIAN_POINT('Ctrl Pts',(-7.07057502871922,-181.620483118095,
4.08219839617346));
#33786=CARTESIAN_POINT('Ctrl Pts',(-4.71371668580301,-181.445483118095,
8.16439679232994));
#33787=CARTESIAN_POINT('Ctrl Pts',(1.47018674401621E-11,-181.270483118095,
8.16439679232146));
#33788=CARTESIAN_POINT('Ctrl Pts',(4.71371668583241,-181.095483118095,8.16439679231297));
#33789=CARTESIAN_POINT('Ctrl Pts',(7.07057502873392,-180.920483118095,4.082198396148));
#33790=CARTESIAN_POINT('Ctrl Pts',(9.42743337163542,-180.745483118095,-1.69756769845304E-11));
#33791=CARTESIAN_POINT('Ctrl Pts',(7.07057502871922,-180.570483118095,-4.08219839617346));
#33792=CARTESIAN_POINT('Ctrl Pts',(4.71371668580301,-180.395483118095,-8.16439679232994));
#33793=CARTESIAN_POINT('Ctrl Pts',(-1.4702867290402E-11,-180.220483118095,
-8.16439679232146));
#33794=CARTESIAN_POINT('Ctrl Pts',(-4.71371668583241,-180.045483118095,
-8.16439679231297));
#33795=CARTESIAN_POINT('Ctrl Pts',(-7.07057502873392,-179.870483118095,
-4.082198396148));
#33796=CARTESIAN_POINT('Ctrl Pts',(-9.42743337163542,-179.695483118095,
1.69768315121407E-11));
#33797=CARTESIAN_POINT('Ctrl Pts',(-7.07057502871922,-179.520483118095,
4.08219839617346));
#33798=CARTESIAN_POINT('Ctrl Pts',(-4.71371668580301,-179.345483118095,
8.16439679232994));
#33799=CARTESIAN_POINT('Ctrl Pts',(1.47018674401621E-11,-179.170483118095,
8.16439679232146));
#33800=CARTESIAN_POINT('Ctrl Pts',(4.71371668583241,-178.995483118095,8.16439679231297));
#33801=CARTESIAN_POINT('Ctrl Pts',(7.07057502873392,-178.820483118095,4.082198396148));
#33802=CARTESIAN_POINT('Ctrl Pts',(9.42743337163542,-178.645483118095,-1.69756769845304E-11));
#33803=CARTESIAN_POINT('Ctrl Pts',(7.07057502871922,-178.470483118095,-4.08219839617346));
#33804=CARTESIAN_POINT('Ctrl Pts',(4.71371668580301,-178.295483118095,-8.16439679232994));
#33805=CARTESIAN_POINT('Ctrl Pts',(-1.4702867290402E-11,-178.120483118095,
-8.16439679232146));
#33806=CARTESIAN_POINT('Ctrl Pts',(-4.71371668583241,-177.945483118095,
-8.16439679231297));
#33807=CARTESIAN_POINT('Ctrl Pts',(-7.07057502873392,-177.770483118095,
-4.082198396148));
#33808=CARTESIAN_POINT('Ctrl Pts',(-9.42743337163542,-177.595483118095,
1.69768315121407E-11));
#33809=CARTESIAN_POINT('Ctrl Pts',(-7.07057502871922,-177.420483118095,
4.08219839617346));
#33810=CARTESIAN_POINT('Ctrl Pts',(-4.71371668580301,-177.245483118095,
8.16439679232994));
#33811=CARTESIAN_POINT('Ctrl Pts',(1.47018674401621E-11,-177.070483118095,
8.16439679232146));
#33812=CARTESIAN_POINT('Ctrl Pts',(4.71371668583241,-176.895483118095,8.16439679231297));
#33813=CARTESIAN_POINT('Ctrl Pts',(7.07057502873392,-176.720483118095,4.082198396148));
#33814=CARTESIAN_POINT('Ctrl Pts',(9.42743337163542,-176.545483118095,-1.69756769845304E-11));
#33815=CARTESIAN_POINT('Ctrl Pts',(7.07057502871922,-176.370483118095,-4.08219839617346));
#33816=CARTESIAN_POINT('Ctrl Pts',(4.71371668580301,-176.195483118095,-8.16439679232994));
#33817=CARTESIAN_POINT('Ctrl Pts',(-1.4702867290402E-11,-176.020483118095,
-8.16439679232146));
#33818=CARTESIAN_POINT('Ctrl Pts',(-4.71371668583241,-175.845483118095,
-8.16439679231297));
#33819=CARTESIAN_POINT('Ctrl Pts',(-7.07057502873392,-175.670483118095,
-4.082198396148));
#33820=CARTESIAN_POINT('Ctrl Pts',(-9.42743337163542,-175.495483118095,
1.69768315121407E-11));
#33821=CARTESIAN_POINT('Ctrl Pts',(-7.07057502871922,-175.320483118095,
4.08219839617346));
#33822=CARTESIAN_POINT('Ctrl Pts',(-4.71371668580301,-175.145483118095,
8.16439679232994));
#33823=CARTESIAN_POINT('Ctrl Pts',(1.47018674401621E-11,-174.970483118095,
8.16439679232146));
#33824=CARTESIAN_POINT('Ctrl Pts',(4.71371668583241,-174.795483118095,8.16439679231297));
#33825=CARTESIAN_POINT('Ctrl Pts',(7.07057502873392,-174.620483118095,4.082198396148));
#33826=CARTESIAN_POINT('Ctrl Pts',(9.42743337163542,-174.445483118095,-1.69756769845304E-11));
#33827=CARTESIAN_POINT('Ctrl Pts',(7.07057502871922,-174.270483118095,-4.08219839617346));
#33828=CARTESIAN_POINT('Ctrl Pts',(4.71371668580301,-174.095483118095,-8.16439679232994));
#33829=CARTESIAN_POINT('Ctrl Pts',(-1.4702867290402E-11,-173.920483118095,
-8.16439679232146));
#33830=CARTESIAN_POINT('Ctrl Pts',(-4.71371668583241,-173.745483118095,
-8.16439679231297));
#33831=CARTESIAN_POINT('Ctrl Pts',(-7.07057502873392,-173.570483118095,
-4.082198396148));
#33832=CARTESIAN_POINT('Ctrl Pts',(-9.42743337163542,-173.395483118095,
1.69768315121407E-11));
#33833=CARTESIAN_POINT('Ctrl Pts',(-7.07057502871922,-173.220483118095,
4.08219839617346));
#33834=CARTESIAN_POINT('Ctrl Pts',(-4.71371668580301,-173.045483118095,
8.16439679232994));
#33835=CARTESIAN_POINT('Ctrl Pts',(1.47018674401621E-11,-172.870483118095,
8.16439679232146));
#33836=CARTESIAN_POINT('Ctrl Pts',(4.71371668583241,-172.695483118095,8.16439679231297));
#33837=CARTESIAN_POINT('Ctrl Pts',(7.07057502873392,-172.520483118095,4.082198396148));
#33838=CARTESIAN_POINT('Ctrl Pts',(9.42743337163542,-172.345483118095,-1.69756769845304E-11));
#33839=CARTESIAN_POINT('Ctrl Pts',(7.07057502871922,-172.170483118095,-4.08219839617346));
#33840=CARTESIAN_POINT('Ctrl Pts',(4.71371668580301,-171.995483118095,-8.16439679232994));
#33841=CARTESIAN_POINT('Ctrl Pts',(-1.4702867290402E-11,-171.820483118095,
-8.16439679232146));
#33842=CARTESIAN_POINT('Ctrl Pts',(-4.71371668583241,-171.645483118095,
-8.16439679231297));
#33843=CARTESIAN_POINT('Ctrl Pts',(-7.07057502873392,-171.470483118095,
-4.082198396148));
#33844=CARTESIAN_POINT('Ctrl Pts',(-9.42743337163542,-171.295483118095,
1.69768315121407E-11));
#33845=CARTESIAN_POINT('Ctrl Pts',(-7.07057502871922,-171.120483118095,
4.08219839617346));
#33846=CARTESIAN_POINT('Ctrl Pts',(-4.71371668580301,-170.945483118095,
8.16439679232994));
#33847=CARTESIAN_POINT('Ctrl Pts',(1.47018674401621E-11,-170.770483118095,
8.16439679232146));
#33848=CARTESIAN_POINT('Ctrl Pts',(4.71371668583241,-170.595483118095,8.16439679231297));
#33849=CARTESIAN_POINT('Ctrl Pts',(7.07057502873392,-170.420483118095,4.082198396148));
#33850=CARTESIAN_POINT('Ctrl Pts',(9.42743337163542,-170.245483118095,-1.69756769845304E-11));
#33851=CARTESIAN_POINT('Ctrl Pts',(7.07057502871922,-170.070483118095,-4.08219839617346));
#33852=CARTESIAN_POINT('Ctrl Pts',(4.71371668580301,-169.895483118095,-8.16439679232994));
#33853=CARTESIAN_POINT('Ctrl Pts',(-1.4702867290402E-11,-169.720483118095,
-8.16439679232146));
#33854=CARTESIAN_POINT('Ctrl Pts',(-4.71371668583241,-169.545483118095,
-8.16439679231297));
#33855=CARTESIAN_POINT('Ctrl Pts',(-7.07057502873392,-169.370483118095,
-4.082198396148));
#33856=CARTESIAN_POINT('Ctrl Pts',(-9.42743337163542,-169.195483118095,
1.69768315121407E-11));
#33857=CARTESIAN_POINT('Ctrl Pts',(-7.07057502871922,-169.020483118095,
4.08219839617346));
#33858=CARTESIAN_POINT('Ctrl Pts',(-4.71371668580301,-168.845483118095,
8.16439679232994));
#33859=CARTESIAN_POINT('Ctrl Pts',(1.47018674401621E-11,-168.670483118095,
8.16439679232146));
#33860=CARTESIAN_POINT('Ctrl Pts',(4.71371668583241,-168.495483118095,8.16439679231297));
#33861=CARTESIAN_POINT('Ctrl Pts',(7.07057502873392,-168.320483118095,4.082198396148));
#33862=CARTESIAN_POINT('Ctrl Pts',(9.42743337163542,-168.145483118095,-1.69756769845304E-11));
#33863=CARTESIAN_POINT('Ctrl Pts',(7.07057502871922,-167.970483118095,-4.08219839617346));
#33864=CARTESIAN_POINT('Ctrl Pts',(4.71371668580301,-167.795483118095,-8.16439679232994));
#33865=CARTESIAN_POINT('Ctrl Pts',(-1.4702867290402E-11,-167.620483118095,
-8.16439679232146));
#33866=CARTESIAN_POINT('Ctrl Pts',(-4.71371668583241,-167.445483118095,
-8.16439679231297));
#33867=CARTESIAN_POINT('Ctrl Pts',(-7.07057502873392,-167.270483118095,
-4.082198396148));
#33868=CARTESIAN_POINT('Ctrl Pts',(-9.42743337163542,-167.095483118095,
1.69768315121407E-11));
#33869=CARTESIAN_POINT('Ctrl Pts',(-7.07057502871922,-166.920483118095,
4.08219839617346));
#33870=CARTESIAN_POINT('Ctrl Pts',(-4.71371668580301,-166.745483118095,
8.16439679232994));
#33871=CARTESIAN_POINT('Ctrl Pts',(1.47018674401621E-11,-166.570483118095,
8.16439679232146));
#33872=CARTESIAN_POINT('Ctrl Pts',(4.71371668583241,-166.395483118095,8.16439679231297));
#33873=CARTESIAN_POINT('Ctrl Pts',(7.07057502873392,-166.220483118095,4.082198396148));
#33874=CARTESIAN_POINT('Ctrl Pts',(9.42743337163542,-166.045483118095,-1.69756769845304E-11));
#33875=CARTESIAN_POINT('Ctrl Pts',(7.07057502871922,-165.870483118095,-4.08219839617346));
#33876=CARTESIAN_POINT('Ctrl Pts',(4.71371668580301,-165.695483118095,-8.16439679232994));
#33877=CARTESIAN_POINT('Ctrl Pts',(-1.4702867290402E-11,-165.520483118095,
-8.16439679232146));
#33878=CARTESIAN_POINT('Ctrl Pts',(-4.71371668583241,-165.345483118095,
-8.16439679231297));
#33879=CARTESIAN_POINT('Ctrl Pts',(-7.07057502873392,-165.170483118095,
-4.082198396148));
#33880=CARTESIAN_POINT('Ctrl Pts',(-9.42743337163542,-164.995483118095,
1.69768315121407E-11));
#33881=CARTESIAN_POINT('Ctrl Pts',(-7.07057502871922,-164.820483118095,
4.08219839617346));
#33882=CARTESIAN_POINT('Ctrl Pts',(-4.71371668580301,-164.645483118095,
8.16439679232994));
#33883=CARTESIAN_POINT('Ctrl Pts',(1.47018674401621E-11,-164.470483118095,
8.16439679232146));
#33884=CARTESIAN_POINT('Ctrl Pts',(4.71371668583241,-164.295483118095,8.16439679231297));
#33885=CARTESIAN_POINT('Ctrl Pts',(7.07057502873392,-164.120483118095,4.082198396148));
#33886=CARTESIAN_POINT('Ctrl Pts',(9.42743337163542,-163.945483118095,-1.69756769845304E-11));
#33887=CARTESIAN_POINT('Ctrl Pts',(7.07057502871922,-163.770483118095,-4.08219839617346));
#33888=CARTESIAN_POINT('Ctrl Pts',(4.71371668580301,-163.595483118095,-8.16439679232994));
#33889=CARTESIAN_POINT('Ctrl Pts',(-1.4702867290402E-11,-163.420483118095,
-8.16439679232146));
#33890=CARTESIAN_POINT('Ctrl Pts',(-4.71371668583241,-163.245483118095,
-8.16439679231297));
#33891=CARTESIAN_POINT('Ctrl Pts',(-7.07057502873392,-163.070483118095,
-4.082198396148));
#33892=CARTESIAN_POINT('Ctrl Pts',(-9.42743337163542,-162.895483118095,
1.69768315121407E-11));
#33893=CARTESIAN_POINT('Ctrl Pts',(-7.07057502871922,-162.720483118095,
4.08219839617346));
#33894=CARTESIAN_POINT('Ctrl Pts',(-4.71371668580301,-162.545483118095,
8.16439679232994));
#33895=CARTESIAN_POINT('Ctrl Pts',(1.47018674401621E-11,-162.370483118095,
8.16439679232146));
#33896=CARTESIAN_POINT('Ctrl Pts',(4.71371668583241,-162.195483118095,8.16439679231297));
#33897=CARTESIAN_POINT('Ctrl Pts',(7.07057502873392,-162.020483118095,4.082198396148));
#33898=CARTESIAN_POINT('Ctrl Pts',(9.42743337163542,-161.845483118095,-1.69756769845304E-11));
#33899=CARTESIAN_POINT('Ctrl Pts',(7.07057502871922,-161.670483118095,-4.08219839617346));
#33900=CARTESIAN_POINT('Ctrl Pts',(4.71371668580301,-161.495483118095,-8.16439679232994));
#33901=CARTESIAN_POINT('Ctrl Pts',(-1.4702867290402E-11,-161.320483118095,
-8.16439679232146));
#33902=CARTESIAN_POINT('Ctrl Pts',(-4.71371668583241,-161.145483118095,
-8.16439679231297));
#33903=CARTESIAN_POINT('Ctrl Pts',(-7.07057502873392,-160.970483118095,
-4.082198396148));
#33904=CARTESIAN_POINT('Ctrl Pts',(-9.42743337163542,-160.795483118095,
1.69768315121407E-11));
#33905=CARTESIAN_POINT('Ctrl Pts',(-7.07057502871922,-160.620483118095,
4.08219839617346));
#33906=CARTESIAN_POINT('Ctrl Pts',(-4.71371668580301,-160.445483118095,
8.16439679232994));
#33907=CARTESIAN_POINT('Ctrl Pts',(1.47018674401621E-11,-160.270483118095,
8.16439679232146));
#33908=CARTESIAN_POINT('Ctrl Pts',(4.71371668583241,-160.095483118095,8.16439679231297));
#33909=CARTESIAN_POINT('Ctrl Pts',(7.07057502873392,-159.920483118095,4.082198396148));
#33910=CARTESIAN_POINT('Ctrl Pts',(9.42743337163542,-159.745483118095,-1.69756769845304E-11));
#33911=CARTESIAN_POINT('Ctrl Pts',(7.07057502871922,-159.570483118095,-4.08219839617346));
#33912=CARTESIAN_POINT('Ctrl Pts',(4.71371668580301,-159.395483118095,-8.16439679232994));
#33913=CARTESIAN_POINT('Ctrl Pts',(-1.4702867290402E-11,-159.220483118095,
-8.16439679232146));
#33914=CARTESIAN_POINT('Ctrl Pts',(-4.71371668583241,-159.045483118095,
-8.16439679231297));
#33915=CARTESIAN_POINT('Ctrl Pts',(-7.07057502873392,-158.870483118095,
-4.082198396148));
#33916=CARTESIAN_POINT('Ctrl Pts',(-9.42743337163542,-158.695483118095,
1.69768315121407E-11));
#33917=CARTESIAN_POINT('Ctrl Pts',(-7.07057502871922,-158.520483118095,
4.08219839617346));
#33918=CARTESIAN_POINT('Ctrl Pts',(-4.71371668580301,-158.345483118095,
8.16439679232994));
#33919=CARTESIAN_POINT('Ctrl Pts',(1.47018674401621E-11,-158.170483118095,
8.16439679232146));
#33920=CARTESIAN_POINT('Ctrl Pts',(4.71371668583241,-157.995483118095,8.16439679231297));
#33921=CARTESIAN_POINT('Ctrl Pts',(7.07057502873392,-157.820483118095,4.082198396148));
#33922=CARTESIAN_POINT('Ctrl Pts',(9.42743337163542,-157.645483118095,-1.69756769845304E-11));
#33923=CARTESIAN_POINT('Ctrl Pts',(7.07057502871922,-157.470483118095,-4.08219839617346));
#33924=CARTESIAN_POINT('Ctrl Pts',(4.71371668580301,-157.295483118095,-8.16439679232994));
#33925=CARTESIAN_POINT('Ctrl Pts',(-1.4702867290402E-11,-157.120483118095,
-8.16439679232146));
#33926=CARTESIAN_POINT('Ctrl Pts',(-4.71371668583241,-156.945483118095,
-8.16439679231297));
#33927=CARTESIAN_POINT('Ctrl Pts',(-7.07057502873392,-156.770483118095,
-4.082198396148));
#33928=CARTESIAN_POINT('Ctrl Pts',(-9.42743337163542,-156.595483118095,
1.69768315121407E-11));
#33929=CARTESIAN_POINT('Ctrl Pts',(-7.07057502871922,-156.420483118095,
4.08219839617346));
#33930=CARTESIAN_POINT('Ctrl Pts',(-4.71371668580301,-156.245483118095,
8.16439679232994));
#33931=CARTESIAN_POINT('Ctrl Pts',(1.47018674401621E-11,-156.070483118095,
8.16439679232146));
#33932=CARTESIAN_POINT('Ctrl Pts',(4.71371668583241,-155.895483118095,8.16439679231297));
#33933=CARTESIAN_POINT('Ctrl Pts',(7.07057502873392,-155.720483118095,4.082198396148));
#33934=CARTESIAN_POINT('Ctrl Pts',(9.42743337163542,-155.545483118095,-1.69756769845304E-11));
#33935=CARTESIAN_POINT('Ctrl Pts',(7.07057502871922,-155.370483118095,-4.08219839617346));
#33936=CARTESIAN_POINT('Ctrl Pts',(4.71371668580301,-155.195483118095,-8.16439679232994));
#33937=CARTESIAN_POINT('Ctrl Pts',(-1.4702867290402E-11,-155.020483118095,
-8.16439679232146));
#33938=CARTESIAN_POINT('Ctrl Pts',(-4.71371668583241,-154.845483118095,
-8.16439679231297));
#33939=CARTESIAN_POINT('Ctrl Pts',(-7.07057502873392,-154.670483118095,
-4.082198396148));
#33940=CARTESIAN_POINT('Ctrl Pts',(-9.42743337163542,-154.495483118095,
1.69768315121407E-11));
#33941=CARTESIAN_POINT('Ctrl Pts',(-7.07057502871922,-154.320483118095,
4.08219839617346));
#33942=CARTESIAN_POINT('Ctrl Pts',(-4.71371668580301,-154.145483118095,
8.16439679232994));
#33943=CARTESIAN_POINT('Ctrl Pts',(1.47018674401621E-11,-153.970483118095,
8.16439679232146));
#33944=CARTESIAN_POINT('Ctrl Pts',(4.71371668583241,-153.795483118095,8.16439679231297));
#33945=CARTESIAN_POINT('Ctrl Pts',(7.07057502873392,-153.620483118095,4.082198396148));
#33946=CARTESIAN_POINT('Ctrl Pts',(9.42743337163542,-153.445483118095,-1.69756769845304E-11));
#33947=CARTESIAN_POINT('Ctrl Pts',(7.07057502871922,-153.270483118095,-4.08219839617346));
#33948=CARTESIAN_POINT('Ctrl Pts',(4.71371668580301,-153.095483118095,-8.16439679232994));
#33949=CARTESIAN_POINT('Ctrl Pts',(-1.4702867290402E-11,-152.920483118095,
-8.16439679232146));
#33950=CARTESIAN_POINT('Ctrl Pts',(-4.71371668583241,-152.745483118095,
-8.16439679231297));
#33951=CARTESIAN_POINT('Ctrl Pts',(-7.07057502873392,-152.570483118095,
-4.082198396148));
#33952=CARTESIAN_POINT('Ctrl Pts',(-9.42743337163542,-152.395483118095,
1.69768315121407E-11));
#33953=CARTESIAN_POINT('Ctrl Pts',(-7.07057502871922,-152.220483118095,
4.08219839617346));
#33954=CARTESIAN_POINT('Ctrl Pts',(-4.71371668580301,-152.045483118095,
8.16439679232994));
#33955=CARTESIAN_POINT('Ctrl Pts',(1.47018674401621E-11,-151.870483118095,
8.16439679232146));
#33956=CARTESIAN_POINT('Ctrl Pts',(4.71371668583241,-151.695483118095,8.16439679231297));
#33957=CARTESIAN_POINT('Ctrl Pts',(7.07057502873392,-151.520483118095,4.082198396148));
#33958=CARTESIAN_POINT('Ctrl Pts',(9.42743337163542,-151.345483118095,-1.69756769845304E-11));
#33959=CARTESIAN_POINT('Ctrl Pts',(7.07057502871922,-151.170483118095,-4.08219839617346));
#33960=CARTESIAN_POINT('Ctrl Pts',(4.71371668580301,-150.995483118095,-8.16439679232994));
#33961=CARTESIAN_POINT('Ctrl Pts',(-1.4702867290402E-11,-150.820483118095,
-8.16439679232146));
#33962=CARTESIAN_POINT('Ctrl Pts',(-4.71371668583241,-150.645483118095,
-8.16439679231297));
#33963=CARTESIAN_POINT('Ctrl Pts',(-7.07057502873392,-150.470483118095,
-4.082198396148));
#33964=CARTESIAN_POINT('Ctrl Pts',(-9.42743337163542,-150.295483118095,
1.69768315121407E-11));
#33965=CARTESIAN_POINT('Ctrl Pts',(-7.07057502871922,-150.120483118095,
4.08219839617346));
#33966=CARTESIAN_POINT('Ctrl Pts',(-4.71371668580301,-149.945483118095,
8.16439679232994));
#33967=CARTESIAN_POINT('Ctrl Pts',(1.47018674401621E-11,-149.770483118095,
8.16439679232146));
#33968=CARTESIAN_POINT('Ctrl Pts',(4.71371668583241,-149.595483118095,8.16439679231297));
#33969=CARTESIAN_POINT('Ctrl Pts',(7.07057502873392,-149.420483118095,4.082198396148));
#33970=CARTESIAN_POINT('Ctrl Pts',(9.42743337163542,-149.245483118095,-1.69756769845304E-11));
#33971=CARTESIAN_POINT('Ctrl Pts',(7.07057502871922,-149.070483118095,-4.08219839617346));
#33972=CARTESIAN_POINT('Ctrl Pts',(4.71371668580301,-148.895483118095,-8.16439679232994));
#33973=CARTESIAN_POINT('Ctrl Pts',(-1.4702867290402E-11,-148.720483118095,
-8.16439679232146));
#33974=CARTESIAN_POINT('Ctrl Pts',(-4.71371668583241,-148.545483118095,
-8.16439679231297));
#33975=CARTESIAN_POINT('Ctrl Pts',(-7.07057502873392,-148.370483118095,
-4.082198396148));
#33976=CARTESIAN_POINT('Ctrl Pts',(-9.42743337163542,-148.195483118095,
1.69768315121407E-11));
#33977=CARTESIAN_POINT('Ctrl Pts',(-7.07057502871922,-148.020483118095,
4.08219839617346));
#33978=CARTESIAN_POINT('Ctrl Pts',(-4.71371668580301,-147.845483118095,
8.16439679232994));
#33979=CARTESIAN_POINT('Ctrl Pts',(1.47018674401621E-11,-147.670483118095,
8.16439679232146));
#33980=CARTESIAN_POINT('Ctrl Pts',(4.71371668583241,-147.495483118095,8.16439679231297));
#33981=CARTESIAN_POINT('Ctrl Pts',(7.07057502873392,-147.320483118095,4.082198396148));
#33982=CARTESIAN_POINT('Ctrl Pts',(9.42743337163542,-147.145483118095,-1.69756769845304E-11));
#33983=CARTESIAN_POINT('Ctrl Pts',(7.07057502871922,-146.970483118095,-4.08219839617346));
#33984=CARTESIAN_POINT('Ctrl Pts',(4.71371668580301,-146.795483118095,-8.16439679232994));
#33985=CARTESIAN_POINT('Ctrl Pts',(-1.4702867290402E-11,-146.620483118095,
-8.16439679232146));
#33986=CARTESIAN_POINT('Ctrl Pts',(-4.71371668583241,-146.445483118095,
-8.16439679231297));
#33987=CARTESIAN_POINT('Ctrl Pts',(-7.07057502873392,-146.270483118095,
-4.082198396148));
#33988=CARTESIAN_POINT('Ctrl Pts',(-9.42743337163542,-146.095483118095,
1.69768315121407E-11));
#33989=CARTESIAN_POINT('Ctrl Pts',(-7.07057502871922,-145.920483118095,
4.08219839617346));
#33990=CARTESIAN_POINT('Ctrl Pts',(-4.71371668580301,-145.745483118095,
8.16439679232994));
#33991=CARTESIAN_POINT('Ctrl Pts',(1.47018674401621E-11,-145.570483118095,
8.16439679232146));
#33992=CARTESIAN_POINT('Ctrl Pts',(4.71371668583241,-145.395483118095,8.16439679231297));
#33993=CARTESIAN_POINT('Ctrl Pts',(7.07057502873392,-145.220483118095,4.082198396148));
#33994=CARTESIAN_POINT('Ctrl Pts',(9.42743337163542,-145.045483118095,-1.69756769845304E-11));
#33995=CARTESIAN_POINT('Ctrl Pts',(7.07057502871922,-144.870483118095,-4.08219839617346));
#33996=CARTESIAN_POINT('Ctrl Pts',(4.71371668580301,-144.695483118095,-8.16439679232994));
#33997=CARTESIAN_POINT('Ctrl Pts',(-1.4702867290402E-11,-144.520483118095,
-8.16439679232146));
#33998=CARTESIAN_POINT('Ctrl Pts',(-4.71371668583241,-144.345483118095,
-8.16439679231297));
#33999=CARTESIAN_POINT('Ctrl Pts',(-7.07057502873392,-144.170483118095,
-4.082198396148));
#34000=CARTESIAN_POINT('Ctrl Pts',(-9.42743337163542,-143.995483118095,
1.69768315121407E-11));
#34001=CARTESIAN_POINT('Ctrl Pts',(-7.07057502871922,-143.820483118095,
4.08219839617346));
#34002=CARTESIAN_POINT('Ctrl Pts',(-4.71371668580301,-143.645483118095,
8.16439679232994));
#34003=CARTESIAN_POINT('Ctrl Pts',(1.47018674401621E-11,-143.470483118095,
8.16439679232146));
#34004=CARTESIAN_POINT('Ctrl Pts',(4.71371668583241,-143.295483118095,8.16439679231297));
#34005=CARTESIAN_POINT('Ctrl Pts',(7.07057502873392,-143.120483118095,4.082198396148));
#34006=CARTESIAN_POINT('Ctrl Pts',(9.42743337163542,-142.945483118095,-1.69756769845304E-11));
#34007=CARTESIAN_POINT('Ctrl Pts',(7.07057502871922,-142.770483118095,-4.08219839617346));
#34008=CARTESIAN_POINT('Ctrl Pts',(4.71371668580301,-142.595483118095,-8.16439679232994));
#34009=CARTESIAN_POINT('Ctrl Pts',(-1.4702867290402E-11,-142.420483118095,
-8.16439679232146));
#34010=CARTESIAN_POINT('Ctrl Pts',(-4.71371668583241,-142.245483118095,
-8.16439679231297));
#34011=CARTESIAN_POINT('Ctrl Pts',(-7.07057502873392,-142.070483118095,
-4.082198396148));
#34012=CARTESIAN_POINT('Ctrl Pts',(-9.42743337163542,-141.895483118095,
1.69768315121407E-11));
#34013=CARTESIAN_POINT('Ctrl Pts',(-7.07057502871922,-141.720483118095,
4.08219839617346));
#34014=CARTESIAN_POINT('Ctrl Pts',(-4.71371668580301,-141.545483118095,
8.16439679232994));
#34015=CARTESIAN_POINT('Ctrl Pts',(1.47018674401621E-11,-141.370483118095,
8.16439679232146));
#34016=CARTESIAN_POINT('Ctrl Pts',(4.71371668583241,-141.195483118095,8.16439679231297));
#34017=CARTESIAN_POINT('Ctrl Pts',(7.07057502873392,-141.020483118095,4.082198396148));
#34018=CARTESIAN_POINT('Ctrl Pts',(9.42743337163542,-140.845483118095,-1.69756769845304E-11));
#34019=CARTESIAN_POINT('Ctrl Pts',(7.07057502871922,-140.670483118095,-4.08219839617346));
#34020=CARTESIAN_POINT('Ctrl Pts',(4.71371668580301,-140.495483118095,-8.16439679232994));
#34021=CARTESIAN_POINT('Ctrl Pts',(-1.4702867290402E-11,-140.320483118095,
-8.16439679232146));
#34022=CARTESIAN_POINT('Ctrl Pts',(-4.71371668583241,-140.145483118095,
-8.16439679231297));
#34023=CARTESIAN_POINT('Ctrl Pts',(-7.07057502873392,-139.970483118095,
-4.082198396148));
#34024=CARTESIAN_POINT('Ctrl Pts',(-9.42743337163542,-139.795483118095,
1.69768315121407E-11));
#34025=CARTESIAN_POINT('Ctrl Pts',(-7.07057502871922,-139.620483118095,
4.08219839617346));
#34026=CARTESIAN_POINT('Ctrl Pts',(-4.71371668580301,-139.445483118095,
8.16439679232994));
#34027=CARTESIAN_POINT('Ctrl Pts',(1.47018674401621E-11,-139.270483118095,
8.16439679232146));
#34028=CARTESIAN_POINT('Ctrl Pts',(4.71371668583241,-139.095483118095,8.16439679231297));
#34029=CARTESIAN_POINT('Ctrl Pts',(7.07057502873392,-138.920483118095,4.082198396148));
#34030=CARTESIAN_POINT('Ctrl Pts',(9.42743337163542,-138.745483118095,-1.69756769845304E-11));
#34031=CARTESIAN_POINT('Ctrl Pts',(7.07057502871922,-138.570483118095,-4.08219839617346));
#34032=CARTESIAN_POINT('Ctrl Pts',(4.71371668580301,-138.395483118095,-8.16439679232994));
#34033=CARTESIAN_POINT('Ctrl Pts',(-1.4702867290402E-11,-138.220483118095,
-8.16439679232146));
#34034=CARTESIAN_POINT('Ctrl Pts',(-4.71371668583241,-138.045483118095,
-8.16439679231297));
#34035=CARTESIAN_POINT('Ctrl Pts',(-7.07057502873392,-137.870483118095,
-4.082198396148));
#34036=CARTESIAN_POINT('Ctrl Pts',(-9.42743337163542,-137.695483118095,
1.69768315121407E-11));
#34037=CARTESIAN_POINT('Ctrl Pts',(-7.07057502871922,-137.520483118095,
4.08219839617346));
#34038=CARTESIAN_POINT('Ctrl Pts',(-4.71371668580301,-137.345483118095,
8.16439679232994));
#34039=CARTESIAN_POINT('Ctrl Pts',(1.47018674401621E-11,-137.170483118095,
8.16439679232146));
#34040=CARTESIAN_POINT('Ctrl Pts',(4.71371668583241,-136.995483118095,8.16439679231297));
#34041=CARTESIAN_POINT('Ctrl Pts',(7.07057502873392,-136.820483118095,4.082198396148));
#34042=CARTESIAN_POINT('Ctrl Pts',(9.42743337163542,-136.645483118095,-1.69756769845304E-11));
#34043=CARTESIAN_POINT('Ctrl Pts',(7.07057502871922,-136.470483118095,-4.08219839617346));
#34044=CARTESIAN_POINT('Ctrl Pts',(4.71371668580301,-136.295483118095,-8.16439679232994));
#34045=CARTESIAN_POINT('Ctrl Pts',(-1.4702867290402E-11,-136.120483118095,
-8.16439679232146));
#34046=CARTESIAN_POINT('Ctrl Pts',(-4.71371668583241,-135.945483118095,
-8.16439679231297));
#34047=CARTESIAN_POINT('Ctrl Pts',(-7.07057502873392,-135.770483118095,
-4.082198396148));
#34048=CARTESIAN_POINT('Ctrl Pts',(-9.42743337163542,-135.595483118095,
1.69768315121407E-11));
#34049=CARTESIAN_POINT('Ctrl Pts',(-7.07057502871922,-135.420483118095,
4.08219839617346));
#34050=CARTESIAN_POINT('Ctrl Pts',(-4.71371668580301,-135.245483118095,
8.16439679232994));
#34051=CARTESIAN_POINT('Ctrl Pts',(1.47018674401621E-11,-135.070483118095,
8.16439679232146));
#34052=CARTESIAN_POINT('Ctrl Pts',(4.71371668583241,-134.895483118095,8.16439679231297));
#34053=CARTESIAN_POINT('Ctrl Pts',(7.07057502873392,-134.720483118095,4.082198396148));
#34054=CARTESIAN_POINT('Ctrl Pts',(9.42743337163542,-134.545483118095,-1.69756769845304E-11));
#34055=CARTESIAN_POINT('Ctrl Pts',(7.07057502871922,-134.370483118095,-4.08219839617346));
#34056=CARTESIAN_POINT('Ctrl Pts',(4.71371668580301,-134.195483118095,-8.16439679232994));
#34057=CARTESIAN_POINT('Ctrl Pts',(-1.4702867290402E-11,-134.020483118095,
-8.16439679232146));
#34058=CARTESIAN_POINT('Ctrl Pts',(-4.71371668583241,-133.845483118095,
-8.16439679231297));
#34059=CARTESIAN_POINT('Ctrl Pts',(-7.07057502873392,-133.670483118095,
-4.082198396148));
#34060=CARTESIAN_POINT('Ctrl Pts',(-9.42743337163542,-133.495483118095,
1.69768315121407E-11));
#34061=CARTESIAN_POINT('Ctrl Pts',(-7.07057502871922,-133.320483118095,
4.08219839617346));
#34062=CARTESIAN_POINT('Ctrl Pts',(-4.71371668580301,-133.145483118095,
8.16439679232994));
#34063=CARTESIAN_POINT('Ctrl Pts',(1.47018674401621E-11,-132.970483118095,
8.16439679232146));
#34064=CARTESIAN_POINT('Ctrl Pts',(4.71371668583241,-132.795483118095,8.16439679231297));
#34065=CARTESIAN_POINT('Ctrl Pts',(7.07057502873392,-132.620483118095,4.082198396148));
#34066=CARTESIAN_POINT('Ctrl Pts',(9.42743337163542,-132.445483118095,-1.69756769845304E-11));
#34067=CARTESIAN_POINT('Ctrl Pts',(7.07057502871922,-132.270483118095,-4.08219839617346));
#34068=CARTESIAN_POINT('Ctrl Pts',(4.71371668580301,-132.095483118095,-8.16439679232994));
#34069=CARTESIAN_POINT('Ctrl Pts',(-1.4702867290402E-11,-131.920483118095,
-8.16439679232146));
#34070=CARTESIAN_POINT('Ctrl Pts',(-4.71371668583241,-131.745483118095,
-8.16439679231297));
#34071=CARTESIAN_POINT('Ctrl Pts',(-7.07057502873392,-131.570483118095,
-4.082198396148));
#34072=CARTESIAN_POINT('Ctrl Pts',(-9.42743337163542,-131.395483118095,
1.69768315121407E-11));
#34073=CARTESIAN_POINT('Ctrl Pts',(-7.07057502871922,-131.220483118095,
4.08219839617346));
#34074=CARTESIAN_POINT('Ctrl Pts',(-4.71371668580301,-131.045483118095,
8.16439679232994));
#34075=CARTESIAN_POINT('Ctrl Pts',(1.47018674401621E-11,-130.870483118095,
8.16439679232146));
#34076=CARTESIAN_POINT('Ctrl Pts',(4.71371668583241,-130.695483118095,8.16439679231297));
#34077=CARTESIAN_POINT('Ctrl Pts',(7.07057502873392,-130.520483118095,4.082198396148));
#34078=CARTESIAN_POINT('Ctrl Pts',(9.42743337163542,-130.345483118095,-1.69756769845304E-11));
#34079=CARTESIAN_POINT('Ctrl Pts',(7.07057502871922,-130.170483118095,-4.08219839617346));
#34080=CARTESIAN_POINT('Ctrl Pts',(4.71371668580301,-129.995483118095,-8.16439679232994));
#34081=CARTESIAN_POINT('Ctrl Pts',(-1.4702867290402E-11,-129.820483118095,
-8.16439679232146));
#34082=CARTESIAN_POINT('Ctrl Pts',(-4.71371668583241,-129.645483118095,
-8.16439679231297));
#34083=CARTESIAN_POINT('Ctrl Pts',(-7.07057502873392,-129.470483118095,
-4.082198396148));
#34084=CARTESIAN_POINT('Ctrl Pts',(-9.42743337163542,-129.295483118095,
1.69768315121407E-11));
#34085=CARTESIAN_POINT('Ctrl Pts',(-7.07057502871922,-129.120483118095,
4.08219839617346));
#34086=CARTESIAN_POINT('Ctrl Pts',(-4.71371668580301,-128.945483118095,
8.16439679232994));
#34087=CARTESIAN_POINT('Ctrl Pts',(1.47018674401621E-11,-128.770483118095,
8.16439679232146));
#34088=CARTESIAN_POINT('Ctrl Pts',(4.71371668583241,-128.595483118095,8.16439679231297));
#34089=CARTESIAN_POINT('Ctrl Pts',(7.07057502873392,-128.420483118095,4.082198396148));
#34090=CARTESIAN_POINT('Ctrl Pts',(9.42743337163542,-128.245483118095,-1.69756769845304E-11));
#34091=CARTESIAN_POINT('Ctrl Pts',(7.07057502871922,-128.070483118095,-4.08219839617346));
#34092=CARTESIAN_POINT('Ctrl Pts',(4.71371668580301,-127.895483118095,-8.16439679232994));
#34093=CARTESIAN_POINT('Ctrl Pts',(-1.4702867290402E-11,-127.720483118095,
-8.16439679232146));
#34094=CARTESIAN_POINT('Ctrl Pts',(-4.71371668583241,-127.545483118095,
-8.16439679231297));
#34095=CARTESIAN_POINT('Ctrl Pts',(-7.07057502873392,-127.370483118095,
-4.082198396148));
#34096=CARTESIAN_POINT('Ctrl Pts',(-9.42743337163542,-127.195483118095,
1.69768315121407E-11));
#34097=CARTESIAN_POINT('Ctrl Pts',(-7.07057502871922,-127.020483118095,
4.08219839617346));
#34098=CARTESIAN_POINT('Ctrl Pts',(-4.71371668580301,-126.845483118095,
8.16439679232994));
#34099=CARTESIAN_POINT('Ctrl Pts',(1.47018674401621E-11,-126.670483118095,
8.16439679232146));
#34100=CARTESIAN_POINT('Ctrl Pts',(4.71371668583241,-126.495483118095,8.16439679231297));
#34101=CARTESIAN_POINT('Ctrl Pts',(7.07057502873392,-126.320483118095,4.082198396148));
#34102=CARTESIAN_POINT('Ctrl Pts',(9.42743337163542,-126.145483118095,-1.69756769845304E-11));
#34103=CARTESIAN_POINT('Ctrl Pts',(7.07057502871922,-125.970483118095,-4.08219839617346));
#34104=CARTESIAN_POINT('Ctrl Pts',(4.71371668580301,-125.795483118095,-8.16439679232994));
#34105=CARTESIAN_POINT('Ctrl Pts',(-1.4702867290402E-11,-125.620483118095,
-8.16439679232146));
#34106=CARTESIAN_POINT('Ctrl Pts',(-4.71371668583241,-125.445483118095,
-8.16439679231297));
#34107=CARTESIAN_POINT('Ctrl Pts',(-7.07057502873392,-125.270483118095,
-4.082198396148));
#34108=CARTESIAN_POINT('Ctrl Pts',(-9.42743337163542,-125.095483118095,
1.69768315121407E-11));
#34109=CARTESIAN_POINT('Ctrl Pts',(-7.07057502871922,-124.920483118095,
4.08219839617346));
#34110=CARTESIAN_POINT('Ctrl Pts',(-4.71371668580301,-124.745483118095,
8.16439679232994));
#34111=CARTESIAN_POINT('Ctrl Pts',(1.47018674401621E-11,-124.570483118095,
8.16439679232146));
#34112=CARTESIAN_POINT('Ctrl Pts',(4.71371668583241,-124.395483118095,8.16439679231297));
#34113=CARTESIAN_POINT('Ctrl Pts',(7.07057502873392,-124.220483118095,4.082198396148));
#34114=CARTESIAN_POINT('Ctrl Pts',(9.42743337163542,-124.045483118095,-1.69756769845304E-11));
#34115=CARTESIAN_POINT('Ctrl Pts',(7.07057502871922,-123.870483118095,-4.08219839617346));
#34116=CARTESIAN_POINT('Ctrl Pts',(4.71371668580301,-123.695483118095,-8.16439679232994));
#34117=CARTESIAN_POINT('Ctrl Pts',(-1.4702867290402E-11,-123.520483118095,
-8.16439679232146));
#34118=CARTESIAN_POINT('Ctrl Pts',(-4.71371668583241,-123.345483118095,
-8.16439679231297));
#34119=CARTESIAN_POINT('Ctrl Pts',(-7.07057502873392,-123.170483118095,
-4.082198396148));
#34120=CARTESIAN_POINT('Ctrl Pts',(-9.42743337163542,-122.995483118095,
1.69768315121407E-11));
#34121=CARTESIAN_POINT('Ctrl Pts',(-7.07057502871922,-122.820483118095,
4.08219839617346));
#34122=CARTESIAN_POINT('Ctrl Pts',(-4.71371668580301,-122.645483118095,
8.16439679232994));
#34123=CARTESIAN_POINT('Ctrl Pts',(1.47018674401621E-11,-122.470483118095,
8.16439679232146));
#34124=CARTESIAN_POINT('Ctrl Pts',(4.71371668583241,-122.295483118095,8.16439679231297));
#34125=CARTESIAN_POINT('Ctrl Pts',(7.07057502873392,-122.120483118095,4.082198396148));
#34126=CARTESIAN_POINT('Ctrl Pts',(9.42743337163542,-121.945483118095,-1.69756769845304E-11));
#34127=CARTESIAN_POINT('Ctrl Pts',(7.07057502871922,-121.770483118095,-4.08219839617346));
#34128=CARTESIAN_POINT('Ctrl Pts',(4.71371668580301,-121.595483118095,-8.16439679232994));
#34129=CARTESIAN_POINT('Ctrl Pts',(-1.4702867290402E-11,-121.420483118095,
-8.16439679232146));
#34130=CARTESIAN_POINT('Ctrl Pts',(-4.71371668583241,-121.245483118095,
-8.16439679231297));
#34131=CARTESIAN_POINT('Ctrl Pts',(-7.07057502873392,-121.070483118095,
-4.082198396148));
#34132=CARTESIAN_POINT('Ctrl Pts',(-9.42743337163542,-120.895483118095,
1.69768315121407E-11));
#34133=CARTESIAN_POINT('Ctrl Pts',(-7.07057502871922,-120.720483118095,
4.08219839617346));
#34134=CARTESIAN_POINT('Ctrl Pts',(-4.71371668580301,-120.545483118095,
8.16439679232994));
#34135=CARTESIAN_POINT('Ctrl Pts',(1.47018674401621E-11,-120.370483118095,
8.16439679232146));
#34136=CARTESIAN_POINT('Ctrl Pts',(4.71371668583241,-120.195483118095,8.16439679231297));
#34137=CARTESIAN_POINT('Ctrl Pts',(7.07057502873392,-120.020483118095,4.082198396148));
#34138=CARTESIAN_POINT('Ctrl Pts',(9.42743337163542,-119.845483118095,-1.69756769845304E-11));
#34139=CARTESIAN_POINT('Ctrl Pts',(7.07057502871922,-119.670483118095,-4.08219839617346));
#34140=CARTESIAN_POINT('Ctrl Pts',(4.71371668580301,-119.495483118095,-8.16439679232994));
#34141=CARTESIAN_POINT('Ctrl Pts',(-1.4702867290402E-11,-119.320483118095,
-8.16439679232146));
#34142=CARTESIAN_POINT('Ctrl Pts',(-4.71371668583241,-119.145483118095,
-8.16439679231297));
#34143=CARTESIAN_POINT('Ctrl Pts',(-7.07057502873392,-118.970483118095,
-4.082198396148));
#34144=CARTESIAN_POINT('Ctrl Pts',(-9.42743337163542,-118.795483118095,
1.69768315121407E-11));
#34145=CARTESIAN_POINT('Ctrl Pts',(-7.07057502871922,-118.620483118095,
4.08219839617346));
#34146=CARTESIAN_POINT('Ctrl Pts',(-4.71371668580301,-118.445483118095,
8.16439679232994));
#34147=CARTESIAN_POINT('Ctrl Pts',(1.47018674401621E-11,-118.270483118095,
8.16439679232146));
#34148=CARTESIAN_POINT('Ctrl Pts',(4.71371668583241,-118.095483118095,8.16439679231297));
#34149=CARTESIAN_POINT('Ctrl Pts',(7.07057502873392,-117.920483118095,4.082198396148));
#34150=CARTESIAN_POINT('Ctrl Pts',(9.42743337163542,-117.745483118095,-1.69756769845304E-11));
#34151=CARTESIAN_POINT('Ctrl Pts',(7.07057502871922,-117.570483118095,-4.08219839617346));
#34152=CARTESIAN_POINT('Ctrl Pts',(4.71371668580301,-117.395483118095,-8.16439679232994));
#34153=CARTESIAN_POINT('Ctrl Pts',(-1.4702867290402E-11,-117.220483118095,
-8.16439679232146));
#34154=CARTESIAN_POINT('Ctrl Pts',(-4.71371668583241,-117.045483118095,
-8.16439679231297));
#34155=CARTESIAN_POINT('Ctrl Pts',(-7.07057502873392,-116.870483118095,
-4.082198396148));
#34156=CARTESIAN_POINT('Ctrl Pts',(-9.42743337163542,-116.695483118095,
1.69768315121407E-11));
#34157=CARTESIAN_POINT('Ctrl Pts',(-7.07057502871922,-116.520483118095,
4.08219839617346));
#34158=CARTESIAN_POINT('Ctrl Pts',(-4.71371668580301,-116.345483118095,
8.16439679232994));
#34159=CARTESIAN_POINT('Ctrl Pts',(1.47018674401621E-11,-116.170483118095,
8.16439679232146));
#34160=CARTESIAN_POINT('Ctrl Pts',(4.71371668583241,-115.995483118095,8.16439679231297));
#34161=CARTESIAN_POINT('Ctrl Pts',(7.07057502873392,-115.820483118095,4.082198396148));
#34162=CARTESIAN_POINT('Ctrl Pts',(9.42743337163542,-115.645483118095,-1.69756769845304E-11));
#34163=CARTESIAN_POINT('Ctrl Pts',(7.07057502871922,-115.470483118095,-4.08219839617346));
#34164=CARTESIAN_POINT('Ctrl Pts',(4.71371668580301,-115.295483118095,-8.16439679232994));
#34165=CARTESIAN_POINT('Ctrl Pts',(-1.4702867290402E-11,-115.120483118095,
-8.16439679232146));
#34166=CARTESIAN_POINT('Ctrl Pts',(-4.71371668583241,-114.945483118095,
-8.16439679231297));
#34167=CARTESIAN_POINT('Ctrl Pts',(-7.07057502873392,-114.770483118095,
-4.082198396148));
#34168=CARTESIAN_POINT('Ctrl Pts',(-9.42743337163542,-114.595483118095,
1.69768315121407E-11));
#34169=CARTESIAN_POINT('Ctrl Pts',(-7.07057502871922,-114.420483118095,
4.08219839617346));
#34170=CARTESIAN_POINT('Ctrl Pts',(-4.71371668580301,-114.245483118095,
8.16439679232994));
#34171=CARTESIAN_POINT('Ctrl Pts',(1.47018674401621E-11,-114.070483118095,
8.16439679232146));
#34172=CARTESIAN_POINT('Ctrl Pts',(4.71371668583241,-113.895483118095,8.16439679231297));
#34173=CARTESIAN_POINT('Ctrl Pts',(7.07057502873392,-113.720483118095,4.082198396148));
#34174=CARTESIAN_POINT('Ctrl Pts',(9.42743337163542,-113.545483118095,-1.69756769845304E-11));
#34175=CARTESIAN_POINT('Ctrl Pts',(7.07057502871922,-113.370483118095,-4.08219839617346));
#34176=CARTESIAN_POINT('Ctrl Pts',(4.71371668580301,-113.195483118095,-8.16439679232994));
#34177=CARTESIAN_POINT('Ctrl Pts',(-1.4702867290402E-11,-113.020483118095,
-8.16439679232146));
#34178=CARTESIAN_POINT('Ctrl Pts',(-4.71371668583241,-112.845483118095,
-8.16439679231297));
#34179=CARTESIAN_POINT('Ctrl Pts',(-7.07057502873392,-112.670483118095,
-4.082198396148));
#34180=CARTESIAN_POINT('Ctrl Pts',(-9.42743337163542,-112.495483118095,
1.69768315121407E-11));
#34181=CARTESIAN_POINT('Ctrl Pts',(-7.07057502871922,-112.320483118095,
4.08219839617346));
#34182=CARTESIAN_POINT('Ctrl Pts',(-4.71371668580301,-112.145483118095,
8.16439679232994));
#34183=CARTESIAN_POINT('Ctrl Pts',(1.47018674401621E-11,-111.970483118095,
8.16439679232146));
#34184=CARTESIAN_POINT('Ctrl Pts',(4.71371668583241,-111.795483118095,8.16439679231297));
#34185=CARTESIAN_POINT('Ctrl Pts',(7.07057502873392,-111.620483118095,4.082198396148));
#34186=CARTESIAN_POINT('Ctrl Pts',(9.42743337163542,-111.445483118095,-1.69756769845304E-11));
#34187=CARTESIAN_POINT('Ctrl Pts',(7.07057502871922,-111.270483118095,-4.08219839617346));
#34188=CARTESIAN_POINT('Ctrl Pts',(4.71371668580301,-111.095483118095,-8.16439679232994));
#34189=CARTESIAN_POINT('Ctrl Pts',(-1.4702867290402E-11,-110.920483118095,
-8.16439679232146));
#34190=CARTESIAN_POINT('Ctrl Pts',(-4.71371668583241,-110.745483118095,
-8.16439679231297));
#34191=CARTESIAN_POINT('Ctrl Pts',(-7.07057502873392,-110.570483118095,
-4.082198396148));
#34192=CARTESIAN_POINT('Ctrl Pts',(-9.42743337163542,-110.395483118095,
1.69768315121407E-11));
#34193=CARTESIAN_POINT('Ctrl Pts',(-7.07057502871922,-110.220483118095,
4.08219839617346));
#34194=CARTESIAN_POINT('Ctrl Pts',(-4.71371668580301,-110.045483118095,
8.16439679232994));
#34195=CARTESIAN_POINT('Ctrl Pts',(1.47018674401621E-11,-109.870483118095,
8.16439679232146));
#34196=CARTESIAN_POINT('Ctrl Pts',(4.71371668583241,-109.695483118095,8.16439679231297));
#34197=CARTESIAN_POINT('Ctrl Pts',(7.07057502873392,-109.520483118095,4.082198396148));
#34198=CARTESIAN_POINT('Ctrl Pts',(9.42743337163542,-109.345483118095,-1.69756769845304E-11));
#34199=CARTESIAN_POINT('Ctrl Pts',(7.07057502871922,-109.170483118095,-4.08219839617346));
#34200=CARTESIAN_POINT('Ctrl Pts',(4.71371668580301,-108.995483118095,-8.16439679232994));
#34201=CARTESIAN_POINT('Ctrl Pts',(-1.4702867290402E-11,-108.820483118095,
-8.16439679232146));
#34202=CARTESIAN_POINT('Ctrl Pts',(-4.71371668583241,-108.645483118095,
-8.16439679231297));
#34203=CARTESIAN_POINT('Ctrl Pts',(-7.07057502873392,-108.470483118095,
-4.082198396148));
#34204=CARTESIAN_POINT('Ctrl Pts',(-9.42743337163542,-108.295483118095,
1.69768315121407E-11));
#34205=CARTESIAN_POINT('Ctrl Pts',(-7.07057502871922,-108.120483118095,
4.08219839617346));
#34206=CARTESIAN_POINT('Ctrl Pts',(-4.71371668580301,-107.945483118095,
8.16439679232994));
#34207=CARTESIAN_POINT('Ctrl Pts',(1.47018674401621E-11,-107.770483118095,
8.16439679232146));
#34208=CARTESIAN_POINT('Ctrl Pts',(4.71371668583241,-107.595483118095,8.16439679231297));
#34209=CARTESIAN_POINT('Ctrl Pts',(7.07057502873392,-107.420483118095,4.082198396148));
#34210=CARTESIAN_POINT('Ctrl Pts',(9.42743337163542,-107.245483118095,-1.69756769845304E-11));
#34211=CARTESIAN_POINT('Ctrl Pts',(7.07057502871922,-107.070483118095,-4.08219839617346));
#34212=CARTESIAN_POINT('Ctrl Pts',(4.71371668580301,-106.895483118095,-8.16439679232994));
#34213=CARTESIAN_POINT('Ctrl Pts',(-1.4702867290402E-11,-106.720483118095,
-8.16439679232146));
#34214=CARTESIAN_POINT('Ctrl Pts',(-4.71371668583241,-106.545483118095,
-8.16439679231297));
#34215=CARTESIAN_POINT('Ctrl Pts',(-7.07057502873392,-106.370483118095,
-4.082198396148));
#34216=CARTESIAN_POINT('Ctrl Pts',(-9.42743337163542,-106.195483118095,
1.69768315121407E-11));
#34217=CARTESIAN_POINT('Ctrl Pts',(-7.07057502871922,-106.020483118095,
4.08219839617346));
#34218=CARTESIAN_POINT('Ctrl Pts',(-4.71371668580301,-105.845483118095,
8.16439679232994));
#34219=CARTESIAN_POINT('Ctrl Pts',(1.47018674401621E-11,-105.670483118095,
8.16439679232146));
#34220=CARTESIAN_POINT('Ctrl Pts',(4.71371668583241,-105.495483118095,8.16439679231297));
#34221=CARTESIAN_POINT('Ctrl Pts',(7.07057502873392,-105.320483118095,4.082198396148));
#34222=CARTESIAN_POINT('Ctrl Pts',(9.42743337163542,-105.145483118095,-1.69756769845304E-11));
#34223=CARTESIAN_POINT('Ctrl Pts',(7.07057502871922,-104.970483118095,-4.08219839617346));
#34224=CARTESIAN_POINT('Ctrl Pts',(4.71371668580301,-104.795483118095,-8.16439679232994));
#34225=CARTESIAN_POINT('Ctrl Pts',(-1.4702867290402E-11,-104.620483118095,
-8.16439679232146));
#34226=CARTESIAN_POINT('Ctrl Pts',(-4.71371668583241,-104.445483118095,
-8.16439679231297));
#34227=CARTESIAN_POINT('Ctrl Pts',(-7.07057502873392,-104.270483118095,
-4.082198396148));
#34228=CARTESIAN_POINT('Ctrl Pts',(-9.42743337163542,-104.095483118095,
1.69768315121407E-11));
#34229=CARTESIAN_POINT('Ctrl Pts',(-7.07057502871922,-103.920483118095,
4.08219839617346));
#34230=CARTESIAN_POINT('Ctrl Pts',(-4.71371668580301,-103.745483118095,
8.16439679232994));
#34231=CARTESIAN_POINT('Ctrl Pts',(1.47018674401621E-11,-103.570483118095,
8.16439679232146));
#34232=CARTESIAN_POINT('Ctrl Pts',(4.71371668583241,-103.395483118095,8.16439679231297));
#34233=CARTESIAN_POINT('Ctrl Pts',(7.07057502873392,-103.220483118095,4.082198396148));
#34234=CARTESIAN_POINT('Ctrl Pts',(9.42743337163542,-103.045483118095,-1.69756769845304E-11));
#34235=CARTESIAN_POINT('Ctrl Pts',(7.07057502871922,-102.870483118095,-4.08219839617346));
#34236=CARTESIAN_POINT('Ctrl Pts',(4.71371668580301,-102.695483118095,-8.16439679232994));
#34237=CARTESIAN_POINT('Ctrl Pts',(-1.4702867290402E-11,-102.520483118095,
-8.16439679232146));
#34238=CARTESIAN_POINT('Ctrl Pts',(-4.71371668583241,-102.345483118095,
-8.16439679231297));
#34239=CARTESIAN_POINT('Ctrl Pts',(-7.07057502873392,-102.170483118095,
-4.082198396148));
#34240=CARTESIAN_POINT('Ctrl Pts',(-9.42743337163542,-101.995483118095,
1.69768315121407E-11));
#34241=CARTESIAN_POINT('Ctrl Pts',(-7.07057502871922,-101.820483118095,
4.08219839617346));
#34242=CARTESIAN_POINT('Ctrl Pts',(-4.71371668580301,-101.645483118095,
8.16439679232994));
#34243=CARTESIAN_POINT('Ctrl Pts',(1.47018674401621E-11,-101.470483118095,
8.16439679232146));
#34244=CARTESIAN_POINT('Ctrl Pts',(4.71371668583241,-101.295483118095,8.16439679231297));
#34245=CARTESIAN_POINT('Ctrl Pts',(7.07057502873392,-101.120483118095,4.082198396148));
#34246=CARTESIAN_POINT('Ctrl Pts',(9.42743337163542,-100.945483118095,-1.69756769845304E-11));
#34247=CARTESIAN_POINT('Ctrl Pts',(7.07057502871922,-100.770483118095,-4.08219839617346));
#34248=CARTESIAN_POINT('Ctrl Pts',(4.71371668580301,-100.595483118095,-8.16439679232994));
#34249=CARTESIAN_POINT('Ctrl Pts',(-1.4702867290402E-11,-100.420483118095,
-8.16439679232146));
#34250=CARTESIAN_POINT('Ctrl Pts',(-4.71371668583241,-100.245483118095,
-8.16439679231297));
#34251=CARTESIAN_POINT('Ctrl Pts',(-7.07057502873392,-100.070483118095,
-4.082198396148));
#34252=CARTESIAN_POINT('Ctrl Pts',(-9.42743337163542,-99.8954831180954,
1.69768315121407E-11));
#34253=CARTESIAN_POINT('Ctrl Pts',(-7.07057502871922,-99.7204831180953,
4.08219839617346));
#34254=CARTESIAN_POINT('Ctrl Pts',(-4.71371668580301,-99.5454831180953,
8.16439679232994));
#34255=CARTESIAN_POINT('Ctrl Pts',(1.47018674401621E-11,-99.3704831180953,
8.16439679232146));
#34256=CARTESIAN_POINT('Ctrl Pts',(4.71371668583241,-99.1954831180954,8.16439679231297));
#34257=CARTESIAN_POINT('Ctrl Pts',(7.07057502873392,-99.0204831180954,4.082198396148));
#34258=CARTESIAN_POINT('Ctrl Pts',(9.42743337163542,-98.8454831180953,-1.69756769845304E-11));
#34259=CARTESIAN_POINT('Ctrl Pts',(7.07057502871922,-98.6704831180953,-4.08219839617346));
#34260=CARTESIAN_POINT('Ctrl Pts',(4.71371668580301,-98.4954831180954,-8.16439679232994));
#34261=CARTESIAN_POINT('Ctrl Pts',(-1.4702867290402E-11,-98.3204831180954,
-8.16439679232146));
#34262=CARTESIAN_POINT('Ctrl Pts',(-4.71371668583241,-98.1454831180953,
-8.16439679231297));
#34263=CARTESIAN_POINT('Ctrl Pts',(-7.07057502873392,-97.9704831180953,
-4.082198396148));
#34264=CARTESIAN_POINT('Ctrl Pts',(-9.42743337163542,-97.7954831180953,
1.69768315121407E-11));
#34265=CARTESIAN_POINT('Ctrl Pts',(-7.07057502871922,-97.6204831180954,
4.08219839617346));
#34266=CARTESIAN_POINT('Ctrl Pts',(-4.71371668580301,-97.4454831180954,
8.16439679232994));
#34267=CARTESIAN_POINT('Ctrl Pts',(1.47018674401621E-11,-97.2704831180953,
8.16439679232146));
#34268=CARTESIAN_POINT('Ctrl Pts',(4.71371668583241,-97.0954831180953,8.16439679231297));
#34269=CARTESIAN_POINT('Ctrl Pts',(7.07057502873392,-96.9204831180953,4.082198396148));
#34270=CARTESIAN_POINT('Ctrl Pts',(9.42743337163542,-96.7454831180954,-1.69756769845304E-11));
#34271=CARTESIAN_POINT('Ctrl Pts',(7.07057502871922,-96.5704831180954,-4.08219839617346));
#34272=CARTESIAN_POINT('Ctrl Pts',(4.71371668580301,-96.3954831180953,-8.16439679232994));
#34273=CARTESIAN_POINT('Ctrl Pts',(-1.4702867290402E-11,-96.2204831180954,
-8.16439679232146));
#34274=CARTESIAN_POINT('Ctrl Pts',(-4.71371668583241,-96.0454831180953,
-8.16439679231297));
#34275=CARTESIAN_POINT('Ctrl Pts',(-7.07057502873392,-95.8704831180954,
-4.082198396148));
#34276=CARTESIAN_POINT('Ctrl Pts',(-9.42743337163542,-95.6954831180953,
1.69768315121407E-11));
#34277=CARTESIAN_POINT('Ctrl Pts',(-7.07057502871922,-95.5204831180954,
4.08219839617346));
#34278=CARTESIAN_POINT('Ctrl Pts',(-4.71371668580301,-95.3454831180954,
8.16439679232994));
#34279=CARTESIAN_POINT('Ctrl Pts',(1.47018674401621E-11,-95.1704831180953,
8.16439679232146));
#34280=CARTESIAN_POINT('Ctrl Pts',(4.71371668583241,-94.9954831180954,8.16439679231297));
#34281=CARTESIAN_POINT('Ctrl Pts',(7.07057502873392,-94.8204831180954,4.082198396148));
#34282=CARTESIAN_POINT('Ctrl Pts',(9.42743337163542,-94.6454831180954,-1.69756769845304E-11));
#34283=CARTESIAN_POINT('Ctrl Pts',(7.07057502871922,-94.4704831180954,-4.08219839617346));
#34284=CARTESIAN_POINT('Ctrl Pts',(4.71371668580301,-94.2954831180953,-8.16439679232994));
#34285=CARTESIAN_POINT('Ctrl Pts',(-1.4702867290402E-11,-94.1204831180953,
-8.16439679232146));
#34286=CARTESIAN_POINT('Ctrl Pts',(-4.71371668583241,-93.9454831180954,
-8.16439679231297));
#34287=CARTESIAN_POINT('Ctrl Pts',(-7.07057502873392,-93.7704831180953,
-4.082198396148));
#34288=CARTESIAN_POINT('Ctrl Pts',(-9.42743337163542,-93.5954831180953,
1.69768315121407E-11));
#34289=CARTESIAN_POINT('Ctrl Pts',(-7.07057502871922,-93.4204831180954,
4.08219839617346));
#34290=CARTESIAN_POINT('Ctrl Pts',(-4.71371668580301,-93.2454831180954,
8.16439679232994));
#34291=CARTESIAN_POINT('Ctrl Pts',(1.47018674401621E-11,-93.0704831180954,
8.16439679232146));
#34292=CARTESIAN_POINT('Ctrl Pts',(4.71371668583241,-92.8954831180954,8.16439679231297));
#34293=CARTESIAN_POINT('Ctrl Pts',(7.07057502873392,-92.7204831180954,4.082198396148));
#34294=CARTESIAN_POINT('Ctrl Pts',(9.42743337163542,-92.5454831180953,-1.69756769845304E-11));
#34295=CARTESIAN_POINT('Ctrl Pts',(7.07057502871922,-92.3704831180954,-4.08219839617346));
#34296=CARTESIAN_POINT('Ctrl Pts',(4.71371668580301,-92.1954831180954,-8.16439679232994));
#34297=CARTESIAN_POINT('Ctrl Pts',(-1.4702867290402E-11,-92.0204831180953,
-8.16439679232146));
#34298=CARTESIAN_POINT('Ctrl Pts',(-4.71371668583241,-91.8454831180954,
-8.16439679231297));
#34299=CARTESIAN_POINT('Ctrl Pts',(-7.07057502873392,-91.6704831180954,
-4.082198396148));
#34300=CARTESIAN_POINT('Ctrl Pts',(-9.42743337163542,-91.4954831180954,
1.69768315121407E-11));
#34301=CARTESIAN_POINT('Ctrl Pts',(-7.07057502871922,-91.3204831180953,
4.08219839617346));
#34302=CARTESIAN_POINT('Ctrl Pts',(-4.71371668580301,-91.1454831180954,
8.16439679232994));
#34303=CARTESIAN_POINT('Ctrl Pts',(1.47018674401621E-11,-90.9704831180954,
8.16439679232146));
#34304=CARTESIAN_POINT('Ctrl Pts',(4.71371668583241,-90.7954831180953,8.16439679231297));
#34305=CARTESIAN_POINT('Ctrl Pts',(7.07057502873392,-90.6204831180954,4.082198396148));
#34306=CARTESIAN_POINT('Ctrl Pts',(9.42743337163542,-90.4454831180954,-1.69756769845304E-11));
#34307=CARTESIAN_POINT('Ctrl Pts',(7.07057502871922,-90.2704831180954,-4.08219839617346));
#34308=CARTESIAN_POINT('Ctrl Pts',(4.71371668580301,-90.0954831180954,-8.16439679232994));
#34309=CARTESIAN_POINT('Ctrl Pts',(-1.4702867290402E-11,-89.9204831180954,
-8.16439679232146));
#34310=CARTESIAN_POINT('Ctrl Pts',(-4.71371668583241,-89.7454831180954,
-8.16439679231297));
#34311=CARTESIAN_POINT('Ctrl Pts',(-7.07057502873392,-89.5704831180954,
-4.082198396148));
#34312=CARTESIAN_POINT('Ctrl Pts',(-9.42743337163542,-89.3954831180954,
1.69768315121407E-11));
#34313=CARTESIAN_POINT('Ctrl Pts',(-7.07057502871922,-89.2204831180953,
4.08219839617346));
#34314=CARTESIAN_POINT('Ctrl Pts',(-4.71371668580301,-89.0454831180954,
8.16439679232994));
#34315=CARTESIAN_POINT('Ctrl Pts',(1.47018674401621E-11,-88.8704831180954,
8.16439679232146));
#34316=CARTESIAN_POINT('Ctrl Pts',(4.71371668583241,-88.6954831180954,8.16439679231297));
#34317=CARTESIAN_POINT('Ctrl Pts',(7.07057502873392,-88.5204831180954,4.082198396148));
#34318=CARTESIAN_POINT('Ctrl Pts',(9.42743337163542,-88.3454831180954,-1.69756769845304E-11));
#34319=CARTESIAN_POINT('Ctrl Pts',(7.07057502871922,-88.1704831180954,-4.08219839617346));
#34320=CARTESIAN_POINT('Ctrl Pts',(4.71371668580301,-87.9954831180954,-8.16439679232994));
#34321=CARTESIAN_POINT('Ctrl Pts',(-1.4702867290402E-11,-87.8204831180954,
-8.16439679232146));
#34322=CARTESIAN_POINT('Ctrl Pts',(-4.71371668583241,-87.6454831180954,
-8.16439679231297));
#34323=CARTESIAN_POINT('Ctrl Pts',(-7.07057502873392,-87.4704831180954,
-4.082198396148));
#34324=CARTESIAN_POINT('Ctrl Pts',(-9.42743337163542,-87.2954831180954,
1.69768315121407E-11));
#34325=CARTESIAN_POINT('Ctrl Pts',(-7.07057502871922,-87.1204831180954,
4.08219839617346));
#34326=CARTESIAN_POINT('Ctrl Pts',(-4.71371668580301,-86.9454831180954,
8.16439679232994));
#34327=CARTESIAN_POINT('Ctrl Pts',(1.47018674401621E-11,-86.7704831180954,
8.16439679232146));
#34328=CARTESIAN_POINT('Ctrl Pts',(4.71371668583241,-86.5954831180954,8.16439679231297));
#34329=CARTESIAN_POINT('Ctrl Pts',(7.07057502873392,-86.4204831180953,4.082198396148));
#34330=CARTESIAN_POINT('Ctrl Pts',(9.42743337163542,-86.2454831180954,-1.69756769845304E-11));
#34331=CARTESIAN_POINT('Ctrl Pts',(7.07057502871922,-86.0704831180954,-4.08219839617346));
#34332=CARTESIAN_POINT('Ctrl Pts',(4.71371668580301,-85.8954831180954,-8.16439679232994));
#34333=CARTESIAN_POINT('Ctrl Pts',(-1.4702867290402E-11,-85.7204831180954,
-8.16439679232146));
#34334=CARTESIAN_POINT('Ctrl Pts',(-4.71371668583241,-85.5454831180954,
-8.16439679231297));
#34335=CARTESIAN_POINT('Ctrl Pts',(-7.07057502873392,-85.3704831180954,
-4.082198396148));
#34336=CARTESIAN_POINT('Ctrl Pts',(-9.42743337163542,-85.1954831180954,
1.69768315121407E-11));
#34337=CARTESIAN_POINT('Ctrl Pts',(-7.07057502871922,-85.0204831180954,
4.08219839617346));
#34338=CARTESIAN_POINT('Ctrl Pts',(-4.71371668580301,-84.8454831180954,
8.16439679232994));
#34339=CARTESIAN_POINT('Ctrl Pts',(1.47018674401621E-11,-84.6704831180954,
8.16439679232146));
#34340=CARTESIAN_POINT('Ctrl Pts',(4.71371668583241,-84.4954831180954,8.16439679231297));
#34341=CARTESIAN_POINT('Ctrl Pts',(7.07057502873392,-84.3204831180954,4.082198396148));
#34342=CARTESIAN_POINT('Ctrl Pts',(9.42743337163542,-84.1454831180954,-1.69756769845304E-11));
#34343=CARTESIAN_POINT('Ctrl Pts',(7.07057502871922,-83.9704831180954,-4.08219839617346));
#34344=CARTESIAN_POINT('Ctrl Pts',(4.71371668580301,-83.7954831180954,-8.16439679232994));
#34345=CARTESIAN_POINT('Ctrl Pts',(-1.4702867290402E-11,-83.6204831180954,
-8.16439679232146));
#34346=CARTESIAN_POINT('Ctrl Pts',(-4.71371668583241,-83.4454831180954,
-8.16439679231297));
#34347=CARTESIAN_POINT('Ctrl Pts',(-7.07057502873392,-83.2704831180954,
-4.082198396148));
#34348=CARTESIAN_POINT('Ctrl Pts',(-9.42743337163542,-83.0954831180954,
1.69768315121407E-11));
#34349=CARTESIAN_POINT('Ctrl Pts',(-7.07057502871922,-82.9204831180954,
4.08219839617346));
#34350=CARTESIAN_POINT('Ctrl Pts',(-4.71371668580301,-82.7454831180954,
8.16439679232994));
#34351=CARTESIAN_POINT('Ctrl Pts',(1.47018674401621E-11,-82.5704831180954,
8.16439679232146));
#34352=CARTESIAN_POINT('Ctrl Pts',(4.71371668583241,-82.3954831180954,8.16439679231297));
#34353=CARTESIAN_POINT('Ctrl Pts',(7.07057502873392,-82.2204831180954,4.082198396148));
#34354=CARTESIAN_POINT('Ctrl Pts',(9.42743337163542,-82.0454831180954,-1.69756769845304E-11));
#34355=CARTESIAN_POINT('Ctrl Pts',(7.07057502871922,-81.8704831180954,-4.08219839617346));
#34356=CARTESIAN_POINT('Ctrl Pts',(4.71371668580301,-81.6954831180954,-8.16439679232994));
#34357=CARTESIAN_POINT('Ctrl Pts',(-1.4702867290402E-11,-81.5204831180954,
-8.16439679232146));
#34358=CARTESIAN_POINT('Ctrl Pts',(-4.71371668583241,-81.3454831180954,
-8.16439679231297));
#34359=CARTESIAN_POINT('Ctrl Pts',(-7.07057502873392,-81.1704831180954,
-4.082198396148));
#34360=CARTESIAN_POINT('Ctrl Pts',(-9.42743337163542,-80.9954831180954,
1.69768315121407E-11));
#34361=CARTESIAN_POINT('Ctrl Pts',(-7.07057502871922,-80.8204831180954,
4.08219839617346));
#34362=CARTESIAN_POINT('Ctrl Pts',(-4.71371668580301,-80.6454831180954,
8.16439679232994));
#34363=CARTESIAN_POINT('Ctrl Pts',(1.47018674401621E-11,-80.4704831180954,
8.16439679232146));
#34364=CARTESIAN_POINT('Ctrl Pts',(4.71371668583241,-80.2954831180954,8.16439679231297));
#34365=CARTESIAN_POINT('Ctrl Pts',(7.07057502873392,-80.1204831180954,4.082198396148));
#34366=CARTESIAN_POINT('Ctrl Pts',(9.42743337163542,-79.9454831180954,-1.69756769845304E-11));
#34367=CARTESIAN_POINT('Ctrl Pts',(7.07057502871922,-79.7704831180954,-4.08219839617346));
#34368=CARTESIAN_POINT('Ctrl Pts',(4.71371668580301,-79.5954831180954,-8.16439679232994));
#34369=CARTESIAN_POINT('Ctrl Pts',(-1.4702867290402E-11,-79.4204831180954,
-8.16439679232146));
#34370=CARTESIAN_POINT('Ctrl Pts',(-4.71371668583241,-79.2454831180954,
-8.16439679231297));
#34371=CARTESIAN_POINT('Ctrl Pts',(-7.07057502873392,-79.0704831180954,
-4.082198396148));
#34372=CARTESIAN_POINT('Ctrl Pts',(-9.42743337163542,-78.8954831180954,
1.69768315121407E-11));
#34373=CARTESIAN_POINT('Ctrl Pts',(-7.07057502871922,-78.7204831180954,
4.08219839617346));
#34374=CARTESIAN_POINT('Ctrl Pts',(-4.71371668580301,-78.5454831180954,
8.16439679232994));
#34375=CARTESIAN_POINT('Ctrl Pts',(1.47018674401621E-11,-78.3704831180954,
8.16439679232146));
#34376=CARTESIAN_POINT('Ctrl Pts',(4.71371668583241,-78.1954831180954,8.16439679231297));
#34377=CARTESIAN_POINT('Ctrl Pts',(7.07057502873392,-78.0204831180954,4.082198396148));
#34378=CARTESIAN_POINT('Ctrl Pts',(9.42743337163542,-77.8454831180954,-1.69756769845304E-11));
#34379=CARTESIAN_POINT('Ctrl Pts',(7.07057502871922,-77.6704831180954,-4.08219839617346));
#34380=CARTESIAN_POINT('Ctrl Pts',(4.71371668580301,-77.4954831180954,-8.16439679232994));
#34381=CARTESIAN_POINT('Ctrl Pts',(-1.4702867290402E-11,-77.3204831180954,
-8.16439679232146));
#34382=CARTESIAN_POINT('Ctrl Pts',(-4.71371668583241,-77.1454831180954,
-8.16439679231297));
#34383=CARTESIAN_POINT('Ctrl Pts',(-7.07057502873392,-76.9704831180954,
-4.082198396148));
#34384=CARTESIAN_POINT('Ctrl Pts',(-9.42743337163542,-76.7954831180954,
1.69768315121407E-11));
#34385=CARTESIAN_POINT('Ctrl Pts',(-7.07057502871922,-76.6204831180954,
4.08219839617346));
#34386=CARTESIAN_POINT('Ctrl Pts',(-4.71371668580301,-76.4454831180954,
8.16439679232994));
#34387=CARTESIAN_POINT('Ctrl Pts',(1.47018674401621E-11,-76.2704831180954,
8.16439679232146));
#34388=CARTESIAN_POINT('Ctrl Pts',(4.71371668583241,-76.0954831180954,8.16439679231297));
#34389=CARTESIAN_POINT('Ctrl Pts',(7.07057502873392,-75.9204831180954,4.082198396148));
#34390=CARTESIAN_POINT('Ctrl Pts',(9.42743337163542,-75.7454831180954,-1.69756769845304E-11));
#34391=CARTESIAN_POINT('Ctrl Pts',(7.07057502871922,-75.5704831180954,-4.08219839617346));
#34392=CARTESIAN_POINT('Ctrl Pts',(4.71371668580301,-75.3954831180954,-8.16439679232994));
#34393=CARTESIAN_POINT('Ctrl Pts',(-1.4702867290402E-11,-75.2204831180954,
-8.16439679232146));
#34394=CARTESIAN_POINT('Ctrl Pts',(-4.71371668583241,-75.0454831180954,
-8.16439679231297));
#34395=CARTESIAN_POINT('Ctrl Pts',(-7.07057502873392,-74.8704831180954,
-4.082198396148));
#34396=CARTESIAN_POINT('Ctrl Pts',(-9.42743337163542,-74.6954831180954,
1.69768315121407E-11));
#34397=CARTESIAN_POINT('Ctrl Pts',(-7.07057502871922,-74.5204831180954,
4.08219839617346));
#34398=CARTESIAN_POINT('Ctrl Pts',(-4.71371668580301,-74.3454831180954,
8.16439679232994));
#34399=CARTESIAN_POINT('Ctrl Pts',(1.47018674401621E-11,-74.1704831180954,
8.16439679232146));
#34400=CARTESIAN_POINT('Ctrl Pts',(4.71371668583241,-73.9954831180954,8.16439679231297));
#34401=CARTESIAN_POINT('Ctrl Pts',(7.07057502873392,-73.8204831180954,4.082198396148));
#34402=CARTESIAN_POINT('Ctrl Pts',(9.42743337163542,-73.6454831180954,-1.69756769845304E-11));
#34403=CARTESIAN_POINT('Ctrl Pts',(7.07057502871922,-73.4704831180954,-4.08219839617346));
#34404=CARTESIAN_POINT('Ctrl Pts',(4.71371668580301,-73.2954831180954,-8.16439679232994));
#34405=CARTESIAN_POINT('Ctrl Pts',(-1.4702867290402E-11,-73.1204831180954,
-8.16439679232146));
#34406=CARTESIAN_POINT('Ctrl Pts',(-4.71371668583241,-72.9454831180954,
-8.16439679231297));
#34407=CARTESIAN_POINT('Ctrl Pts',(-7.07057502873392,-72.7704831180954,
-4.082198396148));
#34408=CARTESIAN_POINT('Ctrl Pts',(-9.42743337163542,-72.5954831180954,
1.69768315121407E-11));
#34409=CARTESIAN_POINT('Ctrl Pts',(-7.07057502871922,-72.4204831180954,
4.08219839617346));
#34410=CARTESIAN_POINT('Ctrl Pts',(-4.71371668580301,-72.2454831180954,
8.16439679232994));
#34411=CARTESIAN_POINT('Ctrl Pts',(1.47018674401621E-11,-72.0704831180954,
8.16439679232146));
#34412=CARTESIAN_POINT('Ctrl Pts',(4.71371668583241,-71.8954831180954,8.16439679231297));
#34413=CARTESIAN_POINT('Ctrl Pts',(7.07057502873392,-71.7204831180954,4.082198396148));
#34414=CARTESIAN_POINT('Ctrl Pts',(9.42743337163542,-71.5454831180954,-1.69756769845304E-11));
#34415=CARTESIAN_POINT('Ctrl Pts',(7.07057502871922,-71.3704831180954,-4.08219839617346));
#34416=CARTESIAN_POINT('Ctrl Pts',(4.71371668580301,-71.1954831180954,-8.16439679232994));
#34417=CARTESIAN_POINT('Ctrl Pts',(-1.4702867290402E-11,-71.0204831180954,
-8.16439679232146));
#34418=CARTESIAN_POINT('Ctrl Pts',(-4.71371668583241,-70.8454831180954,
-8.16439679231297));
#34419=CARTESIAN_POINT('Ctrl Pts',(-7.07057502873392,-70.6704831180954,
-4.082198396148));
#34420=CARTESIAN_POINT('Ctrl Pts',(-9.42743337163542,-70.4954831180954,
1.69768315121407E-11));
#34421=CARTESIAN_POINT('Ctrl Pts',(-7.07057502871922,-70.3204831180954,
4.08219839617346));
#34422=CARTESIAN_POINT('Ctrl Pts',(-4.71371668580301,-70.1454831180954,
8.16439679232994));
#34423=CARTESIAN_POINT('Ctrl Pts',(1.47018674401621E-11,-69.9704831180954,
8.16439679232146));
#34424=CARTESIAN_POINT('Ctrl Pts',(4.71371668583241,-69.7954831180954,8.16439679231297));
#34425=CARTESIAN_POINT('Ctrl Pts',(7.07057502873392,-69.6204831180954,4.082198396148));
#34426=CARTESIAN_POINT('Ctrl Pts',(9.42743337163542,-69.4454831180954,-1.69756769845304E-11));
#34427=CARTESIAN_POINT('Ctrl Pts',(7.07057502871922,-69.2704831180954,-4.08219839617346));
#34428=CARTESIAN_POINT('Ctrl Pts',(4.71371668580301,-69.0954831180954,-8.16439679232994));
#34429=CARTESIAN_POINT('Ctrl Pts',(-1.4702867290402E-11,-68.9204831180954,
-8.16439679232146));
#34430=CARTESIAN_POINT('Ctrl Pts',(-4.71371668583241,-68.7454831180954,
-8.16439679231297));
#34431=CARTESIAN_POINT('Ctrl Pts',(-7.07057502873392,-68.5704831180954,
-4.082198396148));
#34432=CARTESIAN_POINT('Ctrl Pts',(-9.42743337163542,-68.3954831180954,
1.69768315121407E-11));
#34433=CARTESIAN_POINT('Ctrl Pts',(-7.07057502871922,-68.2204831180954,
4.08219839617346));
#34434=CARTESIAN_POINT('Ctrl Pts',(-4.71371668580301,-68.0454831180954,
8.16439679232994));
#34435=CARTESIAN_POINT('Ctrl Pts',(1.47018674401621E-11,-67.8704831180954,
8.16439679232146));
#34436=CARTESIAN_POINT('Ctrl Pts',(4.71371668583241,-67.6954831180954,8.16439679231297));
#34437=CARTESIAN_POINT('Ctrl Pts',(7.07057502873392,-67.5204831180954,4.082198396148));
#34438=CARTESIAN_POINT('Ctrl Pts',(9.42743337163542,-67.3454831180954,-1.69756769845304E-11));
#34439=CARTESIAN_POINT('Ctrl Pts',(7.07057502871922,-67.1704831180954,-4.08219839617346));
#34440=CARTESIAN_POINT('Ctrl Pts',(4.71371668580301,-66.9954831180954,-8.16439679232994));
#34441=CARTESIAN_POINT('Ctrl Pts',(-1.4702867290402E-11,-66.8204831180954,
-8.16439679232146));
#34442=CARTESIAN_POINT('Ctrl Pts',(-4.71371668583241,-66.6454831180954,
-8.16439679231297));
#34443=CARTESIAN_POINT('Ctrl Pts',(-7.07057502873392,-66.4704831180954,
-4.082198396148));
#34444=CARTESIAN_POINT('Ctrl Pts',(-9.42743337163542,-66.2954831180954,
1.69768315121407E-11));
#34445=CARTESIAN_POINT('Ctrl Pts',(-7.07057502871922,-66.1204831180954,
4.08219839617346));
#34446=CARTESIAN_POINT('Ctrl Pts',(-4.71371668580301,-65.9454831180954,
8.16439679232994));
#34447=CARTESIAN_POINT('Ctrl Pts',(1.47018674401621E-11,-65.7704831180954,
8.16439679232146));
#34448=CARTESIAN_POINT('Ctrl Pts',(4.71371668583241,-65.5954831180954,8.16439679231297));
#34449=CARTESIAN_POINT('Ctrl Pts',(7.07057502873392,-65.4204831180954,4.082198396148));
#34450=CARTESIAN_POINT('Ctrl Pts',(9.42743337163542,-65.2454831180954,-1.69756769845304E-11));
#34451=CARTESIAN_POINT('Ctrl Pts',(7.07057502871922,-65.0704831180954,-4.08219839617346));
#34452=CARTESIAN_POINT('Ctrl Pts',(4.71371668580301,-64.8954831180954,-8.16439679232994));
#34453=CARTESIAN_POINT('Ctrl Pts',(-1.4702867290402E-11,-64.7204831180954,
-8.16439679232146));
#34454=CARTESIAN_POINT('Ctrl Pts',(-4.71371668583241,-64.5454831180954,
-8.16439679231297));
#34455=CARTESIAN_POINT('Ctrl Pts',(-7.07057502873392,-64.3704831180954,
-4.082198396148));
#34456=CARTESIAN_POINT('Ctrl Pts',(-9.42743337163542,-64.1954831180954,
1.69768315121407E-11));
#34457=CARTESIAN_POINT('Ctrl Pts',(-7.07057502871922,-64.0204831180954,
4.08219839617346));
#34458=CARTESIAN_POINT('Ctrl Pts',(-4.71371668580301,-63.8454831180954,
8.16439679232994));
#34459=CARTESIAN_POINT('Ctrl Pts',(1.47018674401621E-11,-63.6704831180954,
8.16439679232146));
#34460=CARTESIAN_POINT('Ctrl Pts',(4.71371668583241,-63.4954831180954,8.16439679231297));
#34461=CARTESIAN_POINT('Ctrl Pts',(7.07057502873392,-63.3204831180954,4.082198396148));
#34462=CARTESIAN_POINT('Ctrl Pts',(9.42743337163542,-63.1454831180954,-1.69756769845304E-11));
#34463=CARTESIAN_POINT('Ctrl Pts',(7.07057502871922,-62.9704831180954,-4.08219839617346));
#34464=CARTESIAN_POINT('Ctrl Pts',(4.71371668580301,-62.7954831180954,-8.16439679232994));
#34465=CARTESIAN_POINT('Ctrl Pts',(-1.4702867290402E-11,-62.6204831180954,
-8.16439679232146));
#34466=CARTESIAN_POINT('Ctrl Pts',(-4.71371668583241,-62.4454831180954,
-8.16439679231297));
#34467=CARTESIAN_POINT('Ctrl Pts',(-7.07057502873392,-62.2704831180954,
-4.082198396148));
#34468=CARTESIAN_POINT('Ctrl Pts',(-9.42743337163542,-62.0954831180954,
1.69768315121407E-11));
#34469=CARTESIAN_POINT('Ctrl Pts',(-7.07057502871922,-61.9204831180954,
4.08219839617346));
#34470=CARTESIAN_POINT('Ctrl Pts',(-4.71371668580301,-61.7454831180954,
8.16439679232994));
#34471=CARTESIAN_POINT('Ctrl Pts',(1.47018674401621E-11,-61.5704831180954,
8.16439679232146));
#34472=CARTESIAN_POINT('Ctrl Pts',(4.71371668583241,-61.3954831180954,8.16439679231297));
#34473=CARTESIAN_POINT('Ctrl Pts',(7.07057502873392,-61.2204831180954,4.082198396148));
#34474=CARTESIAN_POINT('Ctrl Pts',(9.42743337163542,-61.0454831180954,-1.69756769845304E-11));
#34475=CARTESIAN_POINT('Ctrl Pts',(7.07057502871922,-60.8704831180954,-4.08219839617346));
#34476=CARTESIAN_POINT('Ctrl Pts',(4.71371668580301,-60.6954831180954,-8.16439679232994));
#34477=CARTESIAN_POINT('Ctrl Pts',(-1.4702867290402E-11,-60.5204831180954,
-8.16439679232146));
#34478=CARTESIAN_POINT('Ctrl Pts',(-4.71371668583241,-60.3454831180954,
-8.16439679231297));
#34479=CARTESIAN_POINT('Ctrl Pts',(-7.07057502873392,-60.1704831180954,
-4.082198396148));
#34480=CARTESIAN_POINT('Ctrl Pts',(-9.42743337163542,-59.9954831180954,
1.69768315121407E-11));
#34481=CARTESIAN_POINT('Ctrl Pts',(-7.07057502871922,-59.8204831180954,
4.08219839617346));
#34482=CARTESIAN_POINT('Ctrl Pts',(-4.71371668580301,-59.6454831180954,
8.16439679232994));
#34483=CARTESIAN_POINT('Ctrl Pts',(1.47018674401621E-11,-59.4704831180955,
8.16439679232146));
#34484=CARTESIAN_POINT('Ctrl Pts',(4.71371668583241,-59.2954831180954,8.16439679231297));
#34485=CARTESIAN_POINT('Ctrl Pts',(7.07057502873392,-59.1204831180954,4.082198396148));
#34486=CARTESIAN_POINT('Ctrl Pts',(9.42743337163542,-58.9454831180954,-1.69756769845304E-11));
#34487=CARTESIAN_POINT('Ctrl Pts',(7.07057502871922,-58.7704831180954,-4.08219839617346));
#34488=CARTESIAN_POINT('Ctrl Pts',(4.71371668580301,-58.5954831180954,-8.16439679232994));
#34489=CARTESIAN_POINT('Ctrl Pts',(-1.4702867290402E-11,-58.4204831180954,
-8.16439679232146));
#34490=CARTESIAN_POINT('Ctrl Pts',(-4.71371668583241,-58.2454831180954,
-8.16439679231297));
#34491=CARTESIAN_POINT('Ctrl Pts',(-7.07057502873392,-58.0704831180954,
-4.082198396148));
#34492=CARTESIAN_POINT('Ctrl Pts',(-9.42743337163542,-57.8954831180954,
1.69768315121407E-11));
#34493=CARTESIAN_POINT('Ctrl Pts',(-7.07057502871922,-57.7204831180954,
4.08219839617346));
#34494=CARTESIAN_POINT('Ctrl Pts',(-4.71371668580301,-57.5454831180954,
8.16439679232994));
#34495=CARTESIAN_POINT('Ctrl Pts',(1.47018674401621E-11,-57.3704831180954,
8.16439679232146));
#34496=CARTESIAN_POINT('Ctrl Pts',(4.71371668583241,-57.1954831180954,8.16439679231297));
#34497=CARTESIAN_POINT('Ctrl Pts',(7.07057502873392,-57.0204831180954,4.082198396148));
#34498=CARTESIAN_POINT('Ctrl Pts',(9.42743337163542,-56.8454831180954,-1.69756769845304E-11));
#34499=CARTESIAN_POINT('Ctrl Pts',(7.07057502871922,-56.6704831180954,-4.08219839617346));
#34500=CARTESIAN_POINT('Ctrl Pts',(4.71371668580301,-56.4954831180954,-8.16439679232994));
#34501=CARTESIAN_POINT('Ctrl Pts',(-1.4702867290402E-11,-56.3204831180954,
-8.16439679232146));
#34502=CARTESIAN_POINT('Ctrl Pts',(-4.71371668583241,-56.1454831180954,
-8.16439679231297));
#34503=CARTESIAN_POINT('Ctrl Pts',(-7.07057502873392,-55.9704831180955,
-4.082198396148));
#34504=CARTESIAN_POINT('Ctrl Pts',(-9.42743337163542,-55.7954831180954,
1.69768315121407E-11));
#34505=CARTESIAN_POINT('Ctrl Pts',(-7.07057502871922,-55.6204831180954,
4.08219839617346));
#34506=CARTESIAN_POINT('Ctrl Pts',(-4.71371668580301,-55.4454831180954,
8.16439679232994));
#34507=CARTESIAN_POINT('Ctrl Pts',(1.47018674401621E-11,-55.2704831180954,
8.16439679232146));
#34508=CARTESIAN_POINT('Ctrl Pts',(4.71371668583241,-55.0954831180955,8.16439679231297));
#34509=CARTESIAN_POINT('Ctrl Pts',(7.07057502873392,-54.9204831180954,4.082198396148));
#34510=CARTESIAN_POINT('Ctrl Pts',(9.42743337163542,-54.7454831180954,-1.69756769845304E-11));
#34511=CARTESIAN_POINT('Ctrl Pts',(7.07057502871922,-54.5704831180954,-4.08219839617346));
#34512=CARTESIAN_POINT('Ctrl Pts',(4.71371668580301,-54.3954831180955,-8.16439679232994));
#34513=CARTESIAN_POINT('Ctrl Pts',(-1.4702867290402E-11,-54.2204831180954,
-8.16439679232146));
#34514=CARTESIAN_POINT('Ctrl Pts',(-4.71371668583241,-54.0454831180954,
-8.16439679231297));
#34515=CARTESIAN_POINT('Ctrl Pts',(-7.07057502873392,-53.8704831180954,
-4.082198396148));
#34516=CARTESIAN_POINT('Ctrl Pts',(-9.42743337163542,-53.6954831180954,
1.69768315121407E-11));
#34517=CARTESIAN_POINT('Ctrl Pts',(-7.07057502871922,-53.5204831180954,
4.08219839617346));
#34518=CARTESIAN_POINT('Ctrl Pts',(-4.71371668580301,-53.3454831180955,
8.16439679232994));
#34519=CARTESIAN_POINT('Ctrl Pts',(1.47018674401621E-11,-53.1704831180954,
8.16439679232146));
#34520=CARTESIAN_POINT('Ctrl Pts',(4.71371668583241,-52.9954831180954,8.16439679231297));
#34521=CARTESIAN_POINT('Ctrl Pts',(7.07057502873392,-52.8204831180955,4.082198396148));
#34522=CARTESIAN_POINT('Ctrl Pts',(9.42743337163542,-52.6454831180954,-1.69756769845304E-11));
#34523=CARTESIAN_POINT('Ctrl Pts',(7.07057502871922,-52.4704831180954,-4.08219839617346));
#34524=CARTESIAN_POINT('Ctrl Pts',(4.71371668580301,-52.2954831180954,-8.16439679232994));
#34525=CARTESIAN_POINT('Ctrl Pts',(-1.4702867290402E-11,-52.1204831180955,
-8.16439679232146));
#34526=CARTESIAN_POINT('Ctrl Pts',(-4.71371668583241,-51.9454831180954,
-8.16439679231297));
#34527=CARTESIAN_POINT('Ctrl Pts',(-7.07057502873392,-51.7704831180955,
-4.082198396148));
#34528=CARTESIAN_POINT('Ctrl Pts',(-9.42743337163542,-51.5954831180955,
1.69768315121407E-11));
#34529=CARTESIAN_POINT('Ctrl Pts',(-7.07057502871922,-51.4204831180954,
4.08219839617346));
#34530=CARTESIAN_POINT('Ctrl Pts',(-4.71371668580301,-51.2454831180955,
8.16439679232994));
#34531=CARTESIAN_POINT('Ctrl Pts',(1.47018674401621E-11,-51.0704831180955,
8.16439679232146));
#34532=CARTESIAN_POINT('Ctrl Pts',(4.71371668583241,-50.8954831180954,8.16439679231297));
#34533=CARTESIAN_POINT('Ctrl Pts',(7.07057502873392,-50.7204831180955,4.082198396148));
#34534=CARTESIAN_POINT('Ctrl Pts',(9.42743337163542,-50.5454831180955,-1.69756769845304E-11));
#34535=CARTESIAN_POINT('Ctrl Pts',(7.07057502871922,-50.3704831180955,-4.08219839617346));
#34536=CARTESIAN_POINT('Ctrl Pts',(4.71371668580301,-50.1954831180954,-8.16439679232994));
#34537=CARTESIAN_POINT('Ctrl Pts',(-1.4702867290402E-11,-50.0204831180955,
-8.16439679232146));
#34538=CARTESIAN_POINT('Ctrl Pts',(-4.71371668583241,-49.8454831180955,
-8.16439679231297));
#34539=CARTESIAN_POINT('Ctrl Pts',(-7.07057502873392,-49.6704831180954,
-4.082198396148));
#34540=CARTESIAN_POINT('Ctrl Pts',(-9.42743337163542,-49.4954831180955,
1.69768315121407E-11));
#34541=CARTESIAN_POINT('Ctrl Pts',(-7.07057502871922,-49.3204831180955,
4.08219839617346));
#34542=CARTESIAN_POINT('Ctrl Pts',(-4.71371668580301,-49.1454831180954,
8.16439679232994));
#34543=CARTESIAN_POINT('Ctrl Pts',(1.47018674401621E-11,-48.9704831180955,
8.16439679232146));
#34544=CARTESIAN_POINT('Ctrl Pts',(4.71371668583241,-48.7954831180955,8.16439679231297));
#34545=CARTESIAN_POINT('Ctrl Pts',(7.07057502873392,-48.6204831180954,4.082198396148));
#34546=CARTESIAN_POINT('Ctrl Pts',(9.42743337163542,-48.4454831180955,-1.69756769845304E-11));
#34547=CARTESIAN_POINT('Ctrl Pts',(7.07057502871922,-48.2704831180955,-4.08219839617346));
#34548=CARTESIAN_POINT('Ctrl Pts',(4.71371668580301,-48.0954831180954,-8.16439679232994));
#34549=CARTESIAN_POINT('Ctrl Pts',(-1.4702867290402E-11,-47.9204831180955,
-8.16439679232146));
#34550=CARTESIAN_POINT('Ctrl Pts',(-4.71371668583241,-47.7454831180955,
-8.16439679231297));
#34551=CARTESIAN_POINT('Ctrl Pts',(-7.07057502873392,-47.5704831180955,
-4.082198396148));
#34552=CARTESIAN_POINT('Ctrl Pts',(-9.42743337163542,-47.3954831180955,
1.69768315121407E-11));
#34553=CARTESIAN_POINT('Ctrl Pts',(-7.07057502871922,-47.2204831180955,
4.08219839617346));
#34554=CARTESIAN_POINT('Ctrl Pts',(-4.71371668580301,-47.0454831180955,
8.16439679232994));
#34555=CARTESIAN_POINT('Ctrl Pts',(1.47018674401621E-11,-46.8704831180955,
8.16439679232146));
#34556=CARTESIAN_POINT('Ctrl Pts',(4.71371668583241,-46.6954831180955,8.16439679231297));
#34557=CARTESIAN_POINT('Ctrl Pts',(7.07057502873392,-46.5204831180954,4.082198396148));
#34558=CARTESIAN_POINT('Ctrl Pts',(9.42743337163542,-46.3454831180955,-1.69756769845304E-11));
#34559=CARTESIAN_POINT('Ctrl Pts',(7.07057502871922,-46.1704831180955,-4.08219839617346));
#34560=CARTESIAN_POINT('Ctrl Pts',(4.71371668580301,-45.9954831180954,-8.16439679232994));
#34561=CARTESIAN_POINT('Ctrl Pts',(-1.4702867290402E-11,-45.8204831180955,
-8.16439679232146));
#34562=CARTESIAN_POINT('Ctrl Pts',(-4.71371668583241,-45.6454831180955,
-8.16439679231297));
#34563=CARTESIAN_POINT('Ctrl Pts',(-7.07057502873392,-45.4704831180955,
-4.082198396148));
#34564=CARTESIAN_POINT('Ctrl Pts',(-9.42743337163542,-45.2954831180954,
1.69768315121407E-11));
#34565=CARTESIAN_POINT('Ctrl Pts',(-7.07057502871922,-45.1204831180955,
4.08219839617346));
#34566=CARTESIAN_POINT('Ctrl Pts',(-4.71371668580301,-44.9454831180955,
8.16439679232994));
#34567=CARTESIAN_POINT('Ctrl Pts',(1.47018674401621E-11,-44.7704831180955,
8.16439679232146));
#34568=CARTESIAN_POINT('Ctrl Pts',(4.71371668583241,-44.5954831180955,8.16439679231297));
#34569=CARTESIAN_POINT('Ctrl Pts',(7.07057502873392,-44.4204831180955,4.082198396148));
#34570=CARTESIAN_POINT('Ctrl Pts',(9.42743337163542,-44.2454831180955,-1.69756769845304E-11));
#34571=CARTESIAN_POINT('Ctrl Pts',(7.07057502871922,-44.0704831180955,-4.08219839617346));
#34572=CARTESIAN_POINT('Ctrl Pts',(4.71371668580301,-43.8954831180955,-8.16439679232994));
#34573=CARTESIAN_POINT('Ctrl Pts',(-1.4702867290402E-11,-43.7204831180955,
-8.16439679232146));
#34574=CARTESIAN_POINT('Ctrl Pts',(-1.4702867290402E-11,-213.553019107145,
-8.16439679232146));
#34575=CARTESIAN_POINT('Ctrl Pts',(-4.71371668583241,-213.378019107145,
-8.16439679231297));
#34576=CARTESIAN_POINT('Ctrl Pts',(-7.07057502873392,-213.203019107145,
-4.082198396148));
#34577=CARTESIAN_POINT('Ctrl Pts',(-9.42743337163542,-213.028019107145,
1.69768315121407E-11));
#34578=CARTESIAN_POINT('Ctrl Pts',(-7.07057502871922,-212.853019107145,
4.08219839617346));
#34579=CARTESIAN_POINT('Ctrl Pts',(-4.71371668580301,-212.678019107145,
8.16439679232994));
#34580=CARTESIAN_POINT('Ctrl Pts',(1.47018674401621E-11,-212.503019107145,
8.16439679232146));
#34581=CARTESIAN_POINT('Ctrl Pts',(4.71371668583241,-212.328019107145,8.16439679231297));
#34582=CARTESIAN_POINT('Ctrl Pts',(7.07057502873392,-212.153019107145,4.082198396148));
#34583=CARTESIAN_POINT('Ctrl Pts',(9.42743337163542,-211.978019107145,-1.69756769845304E-11));
#34584=CARTESIAN_POINT('Ctrl Pts',(7.07057502871922,-211.803019107145,-4.08219839617346));
#34585=CARTESIAN_POINT('Ctrl Pts',(4.71371668580301,-211.628019107145,-8.16439679232994));
#34586=CARTESIAN_POINT('Ctrl Pts',(-1.4702867290402E-11,-211.453019107145,
-8.16439679232146));
#34587=CARTESIAN_POINT('Ctrl Pts',(-4.71371668583241,-211.278019107145,
-8.16439679231297));
#34588=CARTESIAN_POINT('Ctrl Pts',(-7.07057502873392,-211.103019107145,
-4.082198396148));
#34589=CARTESIAN_POINT('Ctrl Pts',(-9.42743337163542,-210.928019107145,
1.69768315121407E-11));
#34590=CARTESIAN_POINT('Ctrl Pts',(-7.07057502871922,-210.753019107145,
4.08219839617346));
#34591=CARTESIAN_POINT('Ctrl Pts',(-4.71371668580301,-210.578019107145,
8.16439679232994));
#34592=CARTESIAN_POINT('Ctrl Pts',(1.47018674401621E-11,-210.403019107145,
8.16439679232146));
#34593=CARTESIAN_POINT('Ctrl Pts',(4.71371668583241,-210.228019107145,8.16439679231297));
#34594=CARTESIAN_POINT('Ctrl Pts',(7.07057502873392,-210.053019107145,4.082198396148));
#34595=CARTESIAN_POINT('Ctrl Pts',(9.42743337163542,-209.878019107145,-1.69756769845304E-11));
#34596=CARTESIAN_POINT('Ctrl Pts',(7.07057502871922,-209.703019107145,-4.08219839617346));
#34597=CARTESIAN_POINT('Ctrl Pts',(4.71371668580301,-209.528019107145,-8.16439679232994));
#34598=CARTESIAN_POINT('Ctrl Pts',(-1.4702867290402E-11,-209.353019107145,
-8.16439679232146));
#34599=CARTESIAN_POINT('Ctrl Pts',(-4.71371668583241,-209.178019107145,
-8.16439679231297));
#34600=CARTESIAN_POINT('Ctrl Pts',(-7.07057502873392,-209.003019107145,
-4.082198396148));
#34601=CARTESIAN_POINT('Ctrl Pts',(-9.42743337163542,-208.828019107145,
1.69768315121407E-11));
#34602=CARTESIAN_POINT('Ctrl Pts',(-7.07057502871922,-208.653019107145,
4.08219839617346));
#34603=CARTESIAN_POINT('Ctrl Pts',(-4.71371668580301,-208.478019107145,
8.16439679232994));
#34604=CARTESIAN_POINT('Ctrl Pts',(1.47018674401621E-11,-208.303019107145,
8.16439679232146));
#34605=CARTESIAN_POINT('Ctrl Pts',(4.71371668583241,-208.128019107145,8.16439679231297));
#34606=CARTESIAN_POINT('Ctrl Pts',(7.07057502873392,-207.953019107145,4.082198396148));
#34607=CARTESIAN_POINT('Ctrl Pts',(9.42743337163542,-207.778019107145,-1.69756769845304E-11));
#34608=CARTESIAN_POINT('Ctrl Pts',(7.07057502871922,-207.603019107145,-4.08219839617346));
#34609=CARTESIAN_POINT('Ctrl Pts',(4.71371668580301,-207.428019107145,-8.16439679232994));
#34610=CARTESIAN_POINT('Ctrl Pts',(-1.4702867290402E-11,-207.253019107145,
-8.16439679232146));
#34611=CARTESIAN_POINT('Ctrl Pts',(-4.71371668583241,-207.078019107145,
-8.16439679231297));
#34612=CARTESIAN_POINT('Ctrl Pts',(-7.07057502873392,-206.903019107145,
-4.082198396148));
#34613=CARTESIAN_POINT('Ctrl Pts',(-9.42743337163542,-206.728019107145,
1.69768315121407E-11));
#34614=CARTESIAN_POINT('Ctrl Pts',(-7.07057502871922,-206.553019107145,
4.08219839617346));
#34615=CARTESIAN_POINT('Ctrl Pts',(-4.71371668580301,-206.378019107145,
8.16439679232994));
#34616=CARTESIAN_POINT('Ctrl Pts',(1.47018674401621E-11,-206.203019107145,
8.16439679232146));
#34617=CARTESIAN_POINT('Ctrl Pts',(4.71371668583241,-206.028019107145,8.16439679231297));
#34618=CARTESIAN_POINT('Ctrl Pts',(7.07057502873392,-205.853019107145,4.082198396148));
#34619=CARTESIAN_POINT('Ctrl Pts',(9.42743337163542,-205.678019107145,-1.69756769845304E-11));
#34620=CARTESIAN_POINT('Ctrl Pts',(7.07057502871922,-205.503019107145,-4.08219839617346));
#34621=CARTESIAN_POINT('Ctrl Pts',(4.71371668580301,-205.328019107145,-8.16439679232994));
#34622=CARTESIAN_POINT('Ctrl Pts',(-1.4702867290402E-11,-205.153019107145,
-8.16439679232146));
#34623=CARTESIAN_POINT('Ctrl Pts',(-4.71371668583241,-204.978019107145,
-8.16439679231297));
#34624=CARTESIAN_POINT('Ctrl Pts',(-7.07057502873392,-204.803019107145,
-4.082198396148));
#34625=CARTESIAN_POINT('Ctrl Pts',(-9.42743337163542,-204.628019107145,
1.69768315121407E-11));
#34626=CARTESIAN_POINT('Ctrl Pts',(-7.07057502871922,-204.453019107145,
4.08219839617346));
#34627=CARTESIAN_POINT('Ctrl Pts',(-4.71371668580301,-204.278019107145,
8.16439679232994));
#34628=CARTESIAN_POINT('Ctrl Pts',(1.47018674401621E-11,-204.103019107145,
8.16439679232146));
#34629=CARTESIAN_POINT('Ctrl Pts',(4.71371668583241,-203.928019107145,8.16439679231297));
#34630=CARTESIAN_POINT('Ctrl Pts',(7.07057502873392,-203.753019107145,4.082198396148));
#34631=CARTESIAN_POINT('Ctrl Pts',(9.42743337163542,-203.578019107145,-1.69756769845304E-11));
#34632=CARTESIAN_POINT('Ctrl Pts',(7.07057502871922,-203.403019107145,-4.08219839617346));
#34633=CARTESIAN_POINT('Ctrl Pts',(4.71371668580301,-203.228019107145,-8.16439679232994));
#34634=CARTESIAN_POINT('Ctrl Pts',(-1.4702867290402E-11,-203.053019107145,
-8.16439679232146));
#34635=CARTESIAN_POINT('Ctrl Pts',(-4.71371668583241,-202.878019107145,
-8.16439679231297));
#34636=CARTESIAN_POINT('Ctrl Pts',(-7.07057502873392,-202.703019107145,
-4.082198396148));
#34637=CARTESIAN_POINT('Ctrl Pts',(-9.42743337163542,-202.528019107145,
1.69768315121407E-11));
#34638=CARTESIAN_POINT('Ctrl Pts',(-7.07057502871922,-202.353019107145,
4.08219839617346));
#34639=CARTESIAN_POINT('Ctrl Pts',(-4.71371668580301,-202.178019107145,
8.16439679232994));
#34640=CARTESIAN_POINT('Ctrl Pts',(1.47018674401621E-11,-202.003019107145,
8.16439679232146));
#34641=CARTESIAN_POINT('Ctrl Pts',(4.71371668583241,-201.828019107145,8.16439679231297));
#34642=CARTESIAN_POINT('Ctrl Pts',(7.07057502873392,-201.653019107145,4.082198396148));
#34643=CARTESIAN_POINT('Ctrl Pts',(9.42743337163542,-201.478019107145,-1.69756769845304E-11));
#34644=CARTESIAN_POINT('Ctrl Pts',(7.07057502871922,-201.303019107145,-4.08219839617346));
#34645=CARTESIAN_POINT('Ctrl Pts',(4.71371668580301,-201.128019107145,-8.16439679232994));
#34646=CARTESIAN_POINT('Ctrl Pts',(-1.4702867290402E-11,-200.953019107145,
-8.16439679232146));
#34647=CARTESIAN_POINT('Ctrl Pts',(-4.71371668583241,-200.778019107145,
-8.16439679231297));
#34648=CARTESIAN_POINT('Ctrl Pts',(-7.07057502873392,-200.603019107145,
-4.082198396148));
#34649=CARTESIAN_POINT('Ctrl Pts',(-9.42743337163542,-200.428019107145,
1.69768315121407E-11));
#34650=CARTESIAN_POINT('Ctrl Pts',(-7.07057502871922,-200.253019107145,
4.08219839617346));
#34651=CARTESIAN_POINT('Ctrl Pts',(-4.71371668580301,-200.078019107145,
8.16439679232994));
#34652=CARTESIAN_POINT('Ctrl Pts',(1.47018674401621E-11,-199.903019107145,
8.16439679232146));
#34653=CARTESIAN_POINT('Ctrl Pts',(4.71371668583241,-199.728019107145,8.16439679231297));
#34654=CARTESIAN_POINT('Ctrl Pts',(7.07057502873392,-199.553019107145,4.082198396148));
#34655=CARTESIAN_POINT('Ctrl Pts',(9.42743337163542,-199.378019107145,-1.69756769845304E-11));
#34656=CARTESIAN_POINT('Ctrl Pts',(7.07057502871922,-199.203019107145,-4.08219839617346));
#34657=CARTESIAN_POINT('Ctrl Pts',(4.71371668580301,-199.028019107145,-8.16439679232994));
#34658=CARTESIAN_POINT('Ctrl Pts',(-1.4702867290402E-11,-198.853019107145,
-8.16439679232146));
#34659=CARTESIAN_POINT('Ctrl Pts',(-4.71371668583241,-198.678019107145,
-8.16439679231297));
#34660=CARTESIAN_POINT('Ctrl Pts',(-7.07057502873392,-198.503019107145,
-4.082198396148));
#34661=CARTESIAN_POINT('Ctrl Pts',(-9.42743337163542,-198.328019107145,
1.69768315121407E-11));
#34662=CARTESIAN_POINT('Ctrl Pts',(-7.07057502871922,-198.153019107145,
4.08219839617346));
#34663=CARTESIAN_POINT('Ctrl Pts',(-4.71371668580301,-197.978019107145,
8.16439679232994));
#34664=CARTESIAN_POINT('Ctrl Pts',(1.47018674401621E-11,-197.803019107145,
8.16439679232146));
#34665=CARTESIAN_POINT('Ctrl Pts',(4.71371668583241,-197.628019107145,8.16439679231297));
#34666=CARTESIAN_POINT('Ctrl Pts',(7.07057502873392,-197.453019107145,4.082198396148));
#34667=CARTESIAN_POINT('Ctrl Pts',(9.42743337163542,-197.278019107145,-1.69756769845304E-11));
#34668=CARTESIAN_POINT('Ctrl Pts',(7.07057502871922,-197.103019107145,-4.08219839617346));
#34669=CARTESIAN_POINT('Ctrl Pts',(4.71371668580301,-196.928019107145,-8.16439679232994));
#34670=CARTESIAN_POINT('Ctrl Pts',(-1.4702867290402E-11,-196.753019107145,
-8.16439679232146));
#34671=CARTESIAN_POINT('Ctrl Pts',(-4.71371668583241,-196.578019107145,
-8.16439679231297));
#34672=CARTESIAN_POINT('Ctrl Pts',(-7.07057502873392,-196.403019107145,
-4.082198396148));
#34673=CARTESIAN_POINT('Ctrl Pts',(-9.42743337163542,-196.228019107145,
1.69768315121407E-11));
#34674=CARTESIAN_POINT('Ctrl Pts',(-7.07057502871922,-196.053019107145,
4.08219839617346));
#34675=CARTESIAN_POINT('Ctrl Pts',(-4.71371668580301,-195.878019107145,
8.16439679232994));
#34676=CARTESIAN_POINT('Ctrl Pts',(1.47018674401621E-11,-195.703019107145,
8.16439679232146));
#34677=CARTESIAN_POINT('Ctrl Pts',(4.71371668583241,-195.528019107145,8.16439679231297));
#34678=CARTESIAN_POINT('Ctrl Pts',(7.07057502873392,-195.353019107145,4.082198396148));
#34679=CARTESIAN_POINT('Ctrl Pts',(9.42743337163542,-195.178019107145,-1.69756769845304E-11));
#34680=CARTESIAN_POINT('Ctrl Pts',(7.07057502871922,-195.003019107145,-4.08219839617346));
#34681=CARTESIAN_POINT('Ctrl Pts',(4.71371668580301,-194.828019107145,-8.16439679232994));
#34682=CARTESIAN_POINT('Ctrl Pts',(-1.4702867290402E-11,-194.653019107145,
-8.16439679232146));
#34683=CARTESIAN_POINT('Ctrl Pts',(-4.71371668583241,-194.478019107145,
-8.16439679231297));
#34684=CARTESIAN_POINT('Ctrl Pts',(-7.07057502873392,-194.303019107145,
-4.082198396148));
#34685=CARTESIAN_POINT('Ctrl Pts',(-9.42743337163542,-194.128019107145,
1.69768315121407E-11));
#34686=CARTESIAN_POINT('Ctrl Pts',(-7.07057502871922,-193.953019107145,
4.08219839617346));
#34687=CARTESIAN_POINT('Ctrl Pts',(-4.71371668580301,-193.778019107145,
8.16439679232994));
#34688=CARTESIAN_POINT('Ctrl Pts',(1.47018674401621E-11,-193.603019107145,
8.16439679232146));
#34689=CARTESIAN_POINT('Ctrl Pts',(4.71371668583241,-193.428019107145,8.16439679231297));
#34690=CARTESIAN_POINT('Ctrl Pts',(7.07057502873392,-193.253019107145,4.082198396148));
#34691=CARTESIAN_POINT('Ctrl Pts',(9.42743337163542,-193.078019107145,-1.69756769845304E-11));
#34692=CARTESIAN_POINT('Ctrl Pts',(7.07057502871922,-192.903019107145,-4.08219839617346));
#34693=CARTESIAN_POINT('Ctrl Pts',(4.71371668580301,-192.728019107145,-8.16439679232994));
#34694=CARTESIAN_POINT('Ctrl Pts',(-1.4702867290402E-11,-192.553019107145,
-8.16439679232146));
#34695=CARTESIAN_POINT('Ctrl Pts',(-4.71371668583241,-192.378019107145,
-8.16439679231297));
#34696=CARTESIAN_POINT('Ctrl Pts',(-7.07057502873392,-192.203019107145,
-4.082198396148));
#34697=CARTESIAN_POINT('Ctrl Pts',(-9.42743337163542,-192.028019107145,
1.69768315121407E-11));
#34698=CARTESIAN_POINT('Ctrl Pts',(-7.07057502871922,-191.853019107145,
4.08219839617346));
#34699=CARTESIAN_POINT('Ctrl Pts',(-4.71371668580301,-191.678019107145,
8.16439679232994));
#34700=CARTESIAN_POINT('Ctrl Pts',(1.47018674401621E-11,-191.503019107145,
8.16439679232146));
#34701=CARTESIAN_POINT('Ctrl Pts',(4.71371668583241,-191.328019107145,8.16439679231297));
#34702=CARTESIAN_POINT('Ctrl Pts',(7.07057502873392,-191.153019107145,4.082198396148));
#34703=CARTESIAN_POINT('Ctrl Pts',(9.42743337163542,-190.978019107145,-1.69756769845304E-11));
#34704=CARTESIAN_POINT('Ctrl Pts',(7.07057502871922,-190.803019107145,-4.08219839617346));
#34705=CARTESIAN_POINT('Ctrl Pts',(4.71371668580301,-190.628019107145,-8.16439679232994));
#34706=CARTESIAN_POINT('Ctrl Pts',(-1.4702867290402E-11,-190.453019107145,
-8.16439679232146));
#34707=CARTESIAN_POINT('Ctrl Pts',(-4.71371668583241,-190.278019107145,
-8.16439679231297));
#34708=CARTESIAN_POINT('Ctrl Pts',(-7.07057502873392,-190.103019107145,
-4.082198396148));
#34709=CARTESIAN_POINT('Ctrl Pts',(-9.42743337163542,-189.928019107145,
1.69768315121407E-11));
#34710=CARTESIAN_POINT('Ctrl Pts',(-7.07057502871922,-189.753019107145,
4.08219839617346));
#34711=CARTESIAN_POINT('Ctrl Pts',(-4.71371668580301,-189.578019107145,
8.16439679232994));
#34712=CARTESIAN_POINT('Ctrl Pts',(1.47018674401621E-11,-189.403019107145,
8.16439679232146));
#34713=CARTESIAN_POINT('Ctrl Pts',(4.71371668583241,-189.228019107145,8.16439679231297));
#34714=CARTESIAN_POINT('Ctrl Pts',(7.07057502873392,-189.053019107145,4.082198396148));
#34715=CARTESIAN_POINT('Ctrl Pts',(9.42743337163542,-188.878019107145,-1.69756769845304E-11));
#34716=CARTESIAN_POINT('Ctrl Pts',(7.07057502871922,-188.703019107145,-4.08219839617346));
#34717=CARTESIAN_POINT('Ctrl Pts',(4.71371668580301,-188.528019107145,-8.16439679232994));
#34718=CARTESIAN_POINT('Ctrl Pts',(-1.4702867290402E-11,-188.353019107145,
-8.16439679232146));
#34719=CARTESIAN_POINT('Ctrl Pts',(-4.71371668583241,-188.178019107145,
-8.16439679231297));
#34720=CARTESIAN_POINT('Ctrl Pts',(-7.07057502873392,-188.003019107145,
-4.082198396148));
#34721=CARTESIAN_POINT('Ctrl Pts',(-9.42743337163542,-187.828019107145,
1.69768315121407E-11));
#34722=CARTESIAN_POINT('Ctrl Pts',(-7.07057502871922,-187.653019107145,
4.08219839617346));
#34723=CARTESIAN_POINT('Ctrl Pts',(-4.71371668580301,-187.478019107145,
8.16439679232994));
#34724=CARTESIAN_POINT('Ctrl Pts',(1.47018674401621E-11,-187.303019107145,
8.16439679232146));
#34725=CARTESIAN_POINT('Ctrl Pts',(4.71371668583241,-187.128019107145,8.16439679231297));
#34726=CARTESIAN_POINT('Ctrl Pts',(7.07057502873392,-186.953019107145,4.082198396148));
#34727=CARTESIAN_POINT('Ctrl Pts',(9.42743337163542,-186.778019107145,-1.69756769845304E-11));
#34728=CARTESIAN_POINT('Ctrl Pts',(7.07057502871922,-186.603019107145,-4.08219839617346));
#34729=CARTESIAN_POINT('Ctrl Pts',(4.71371668580301,-186.428019107145,-8.16439679232994));
#34730=CARTESIAN_POINT('Ctrl Pts',(-1.4702867290402E-11,-186.253019107145,
-8.16439679232146));
#34731=CARTESIAN_POINT('Ctrl Pts',(-4.71371668583241,-186.078019107145,
-8.16439679231297));
#34732=CARTESIAN_POINT('Ctrl Pts',(-7.07057502873392,-185.903019107145,
-4.082198396148));
#34733=CARTESIAN_POINT('Ctrl Pts',(-9.42743337163542,-185.728019107145,
1.69768315121407E-11));
#34734=CARTESIAN_POINT('Ctrl Pts',(-7.07057502871922,-185.553019107145,
4.08219839617346));
#34735=CARTESIAN_POINT('Ctrl Pts',(-4.71371668580301,-185.378019107145,
8.16439679232994));
#34736=CARTESIAN_POINT('Ctrl Pts',(1.47018674401621E-11,-185.203019107145,
8.16439679232146));
#34737=CARTESIAN_POINT('Ctrl Pts',(4.71371668583241,-185.028019107145,8.16439679231297));
#34738=CARTESIAN_POINT('Ctrl Pts',(7.07057502873392,-184.853019107145,4.082198396148));
#34739=CARTESIAN_POINT('Ctrl Pts',(9.42743337163542,-184.678019107145,-1.69756769845304E-11));
#34740=CARTESIAN_POINT('Ctrl Pts',(7.07057502871922,-184.503019107145,-4.08219839617346));
#34741=CARTESIAN_POINT('Ctrl Pts',(4.71371668580301,-184.328019107145,-8.16439679232994));
#34742=CARTESIAN_POINT('Ctrl Pts',(-1.4702867290402E-11,-184.153019107145,
-8.16439679232146));
#34743=CARTESIAN_POINT('Ctrl Pts',(-4.71371668583241,-183.978019107145,
-8.16439679231297));
#34744=CARTESIAN_POINT('Ctrl Pts',(-7.07057502873392,-183.803019107145,
-4.082198396148));
#34745=CARTESIAN_POINT('Ctrl Pts',(-9.42743337163542,-183.628019107145,
1.69768315121407E-11));
#34746=CARTESIAN_POINT('Ctrl Pts',(-7.07057502871922,-183.453019107145,
4.08219839617346));
#34747=CARTESIAN_POINT('Ctrl Pts',(-4.71371668580301,-183.278019107145,
8.16439679232994));
#34748=CARTESIAN_POINT('Ctrl Pts',(1.47018674401621E-11,-183.103019107145,
8.16439679232146));
#34749=CARTESIAN_POINT('Ctrl Pts',(4.71371668583241,-182.928019107145,8.16439679231297));
#34750=CARTESIAN_POINT('Ctrl Pts',(7.07057502873392,-182.753019107145,4.082198396148));
#34751=CARTESIAN_POINT('Ctrl Pts',(9.42743337163542,-182.578019107145,-1.69756769845304E-11));
#34752=CARTESIAN_POINT('Ctrl Pts',(7.07057502871922,-182.403019107145,-4.08219839617346));
#34753=CARTESIAN_POINT('Ctrl Pts',(4.71371668580301,-182.228019107145,-8.16439679232994));
#34754=CARTESIAN_POINT('Ctrl Pts',(-1.4702867290402E-11,-182.053019107145,
-8.16439679232146));
#34755=CARTESIAN_POINT('Ctrl Pts',(-4.71371668583241,-181.878019107145,
-8.16439679231297));
#34756=CARTESIAN_POINT('Ctrl Pts',(-7.07057502873392,-181.703019107145,
-4.082198396148));
#34757=CARTESIAN_POINT('Ctrl Pts',(-9.42743337163542,-181.528019107145,
1.69768315121407E-11));
#34758=CARTESIAN_POINT('Ctrl Pts',(-7.07057502871922,-181.353019107145,
4.08219839617346));
#34759=CARTESIAN_POINT('Ctrl Pts',(-4.71371668580301,-181.178019107145,
8.16439679232994));
#34760=CARTESIAN_POINT('Ctrl Pts',(1.47018674401621E-11,-181.003019107145,
8.16439679232146));
#34761=CARTESIAN_POINT('Ctrl Pts',(4.71371668583241,-180.828019107145,8.16439679231297));
#34762=CARTESIAN_POINT('Ctrl Pts',(7.07057502873392,-180.653019107145,4.082198396148));
#34763=CARTESIAN_POINT('Ctrl Pts',(9.42743337163542,-180.478019107145,-1.69756769845304E-11));
#34764=CARTESIAN_POINT('Ctrl Pts',(7.07057502871922,-180.303019107145,-4.08219839617346));
#34765=CARTESIAN_POINT('Ctrl Pts',(4.71371668580301,-180.128019107145,-8.16439679232994));
#34766=CARTESIAN_POINT('Ctrl Pts',(-1.4702867290402E-11,-179.953019107145,
-8.16439679232146));
#34767=CARTESIAN_POINT('Ctrl Pts',(-4.71371668583241,-179.778019107145,
-8.16439679231297));
#34768=CARTESIAN_POINT('Ctrl Pts',(-7.07057502873392,-179.603019107145,
-4.082198396148));
#34769=CARTESIAN_POINT('Ctrl Pts',(-9.42743337163542,-179.428019107145,
1.69768315121407E-11));
#34770=CARTESIAN_POINT('Ctrl Pts',(-7.07057502871922,-179.253019107145,
4.08219839617346));
#34771=CARTESIAN_POINT('Ctrl Pts',(-4.71371668580301,-179.078019107145,
8.16439679232994));
#34772=CARTESIAN_POINT('Ctrl Pts',(1.47018674401621E-11,-178.903019107145,
8.16439679232146));
#34773=CARTESIAN_POINT('Ctrl Pts',(4.71371668583241,-178.728019107145,8.16439679231297));
#34774=CARTESIAN_POINT('Ctrl Pts',(7.07057502873392,-178.553019107145,4.082198396148));
#34775=CARTESIAN_POINT('Ctrl Pts',(9.42743337163542,-178.378019107145,-1.69756769845304E-11));
#34776=CARTESIAN_POINT('Ctrl Pts',(7.07057502871922,-178.203019107145,-4.08219839617346));
#34777=CARTESIAN_POINT('Ctrl Pts',(4.71371668580301,-178.028019107145,-8.16439679232994));
#34778=CARTESIAN_POINT('Ctrl Pts',(-1.4702867290402E-11,-177.853019107145,
-8.16439679232146));
#34779=CARTESIAN_POINT('Ctrl Pts',(-4.71371668583241,-177.678019107145,
-8.16439679231297));
#34780=CARTESIAN_POINT('Ctrl Pts',(-7.07057502873392,-177.503019107145,
-4.082198396148));
#34781=CARTESIAN_POINT('Ctrl Pts',(-9.42743337163542,-177.328019107145,
1.69768315121407E-11));
#34782=CARTESIAN_POINT('Ctrl Pts',(-7.07057502871922,-177.153019107145,
4.08219839617346));
#34783=CARTESIAN_POINT('Ctrl Pts',(-4.71371668580301,-176.978019107145,
8.16439679232994));
#34784=CARTESIAN_POINT('Ctrl Pts',(1.47018674401621E-11,-176.803019107145,
8.16439679232146));
#34785=CARTESIAN_POINT('Ctrl Pts',(4.71371668583241,-176.628019107145,8.16439679231297));
#34786=CARTESIAN_POINT('Ctrl Pts',(7.07057502873392,-176.453019107145,4.082198396148));
#34787=CARTESIAN_POINT('Ctrl Pts',(9.42743337163542,-176.278019107145,-1.69756769845304E-11));
#34788=CARTESIAN_POINT('Ctrl Pts',(7.07057502871922,-176.103019107145,-4.08219839617346));
#34789=CARTESIAN_POINT('Ctrl Pts',(4.71371668580301,-175.928019107145,-8.16439679232994));
#34790=CARTESIAN_POINT('Ctrl Pts',(-1.4702867290402E-11,-175.753019107145,
-8.16439679232146));
#34791=CARTESIAN_POINT('Ctrl Pts',(-4.71371668583241,-175.578019107145,
-8.16439679231297));
#34792=CARTESIAN_POINT('Ctrl Pts',(-7.07057502873392,-175.403019107145,
-4.082198396148));
#34793=CARTESIAN_POINT('Ctrl Pts',(-9.42743337163542,-175.228019107145,
1.69768315121407E-11));
#34794=CARTESIAN_POINT('Ctrl Pts',(-7.07057502871922,-175.053019107145,
4.08219839617346));
#34795=CARTESIAN_POINT('Ctrl Pts',(-4.71371668580301,-174.878019107145,
8.16439679232994));
#34796=CARTESIAN_POINT('Ctrl Pts',(1.47018674401621E-11,-174.703019107145,
8.16439679232146));
#34797=CARTESIAN_POINT('Ctrl Pts',(4.71371668583241,-174.528019107145,8.16439679231297));
#34798=CARTESIAN_POINT('Ctrl Pts',(7.07057502873392,-174.353019107145,4.082198396148));
#34799=CARTESIAN_POINT('Ctrl Pts',(9.42743337163542,-174.178019107145,-1.69756769845304E-11));
#34800=CARTESIAN_POINT('Ctrl Pts',(7.07057502871922,-174.003019107145,-4.08219839617346));
#34801=CARTESIAN_POINT('Ctrl Pts',(4.71371668580301,-173.828019107145,-8.16439679232994));
#34802=CARTESIAN_POINT('Ctrl Pts',(-1.4702867290402E-11,-173.653019107145,
-8.16439679232146));
#34803=CARTESIAN_POINT('Ctrl Pts',(-4.71371668583241,-173.478019107145,
-8.16439679231297));
#34804=CARTESIAN_POINT('Ctrl Pts',(-7.07057502873392,-173.303019107145,
-4.082198396148));
#34805=CARTESIAN_POINT('Ctrl Pts',(-9.42743337163542,-173.128019107145,
1.69768315121407E-11));
#34806=CARTESIAN_POINT('Ctrl Pts',(-7.07057502871922,-172.953019107145,
4.08219839617346));
#34807=CARTESIAN_POINT('Ctrl Pts',(-4.71371668580301,-172.778019107145,
8.16439679232994));
#34808=CARTESIAN_POINT('Ctrl Pts',(1.47018674401621E-11,-172.603019107145,
8.16439679232146));
#34809=CARTESIAN_POINT('Ctrl Pts',(4.71371668583241,-172.428019107145,8.16439679231297));
#34810=CARTESIAN_POINT('Ctrl Pts',(7.07057502873392,-172.253019107145,4.082198396148));
#34811=CARTESIAN_POINT('Ctrl Pts',(9.42743337163542,-172.078019107145,-1.69756769845304E-11));
#34812=CARTESIAN_POINT('Ctrl Pts',(7.07057502871922,-171.903019107145,-4.08219839617346));
#34813=CARTESIAN_POINT('Ctrl Pts',(4.71371668580301,-171.728019107145,-8.16439679232994));
#34814=CARTESIAN_POINT('Ctrl Pts',(-1.4702867290402E-11,-171.553019107145,
-8.16439679232146));
#34815=CARTESIAN_POINT('Ctrl Pts',(-4.71371668583241,-171.378019107145,
-8.16439679231297));
#34816=CARTESIAN_POINT('Ctrl Pts',(-7.07057502873392,-171.203019107145,
-4.082198396148));
#34817=CARTESIAN_POINT('Ctrl Pts',(-9.42743337163542,-171.028019107145,
1.69768315121407E-11));
#34818=CARTESIAN_POINT('Ctrl Pts',(-7.07057502871922,-170.853019107145,
4.08219839617346));
#34819=CARTESIAN_POINT('Ctrl Pts',(-4.71371668580301,-170.678019107145,
8.16439679232994));
#34820=CARTESIAN_POINT('Ctrl Pts',(1.47018674401621E-11,-170.503019107145,
8.16439679232146));
#34821=CARTESIAN_POINT('Ctrl Pts',(4.71371668583241,-170.328019107145,8.16439679231297));
#34822=CARTESIAN_POINT('Ctrl Pts',(7.07057502873392,-170.153019107145,4.082198396148));
#34823=CARTESIAN_POINT('Ctrl Pts',(9.42743337163542,-169.978019107145,-1.69756769845304E-11));
#34824=CARTESIAN_POINT('Ctrl Pts',(7.07057502871922,-169.803019107145,-4.08219839617346));
#34825=CARTESIAN_POINT('Ctrl Pts',(4.71371668580301,-169.628019107145,-8.16439679232994));
#34826=CARTESIAN_POINT('Ctrl Pts',(-1.4702867290402E-11,-169.453019107145,
-8.16439679232146));
#34827=CARTESIAN_POINT('Ctrl Pts',(-4.71371668583241,-169.278019107145,
-8.16439679231297));
#34828=CARTESIAN_POINT('Ctrl Pts',(-7.07057502873392,-169.103019107145,
-4.082198396148));
#34829=CARTESIAN_POINT('Ctrl Pts',(-9.42743337163542,-168.928019107145,
1.69768315121407E-11));
#34830=CARTESIAN_POINT('Ctrl Pts',(-7.07057502871922,-168.753019107145,
4.08219839617346));
#34831=CARTESIAN_POINT('Ctrl Pts',(-4.71371668580301,-168.578019107145,
8.16439679232994));
#34832=CARTESIAN_POINT('Ctrl Pts',(1.47018674401621E-11,-168.403019107145,
8.16439679232146));
#34833=CARTESIAN_POINT('Ctrl Pts',(4.71371668583241,-168.228019107145,8.16439679231297));
#34834=CARTESIAN_POINT('Ctrl Pts',(7.07057502873392,-168.053019107145,4.082198396148));
#34835=CARTESIAN_POINT('Ctrl Pts',(9.42743337163542,-167.878019107145,-1.69756769845304E-11));
#34836=CARTESIAN_POINT('Ctrl Pts',(7.07057502871922,-167.703019107145,-4.08219839617346));
#34837=CARTESIAN_POINT('Ctrl Pts',(4.71371668580301,-167.528019107145,-8.16439679232994));
#34838=CARTESIAN_POINT('Ctrl Pts',(-1.4702867290402E-11,-167.353019107145,
-8.16439679232146));
#34839=CARTESIAN_POINT('Ctrl Pts',(-4.71371668583241,-167.178019107145,
-8.16439679231297));
#34840=CARTESIAN_POINT('Ctrl Pts',(-7.07057502873392,-167.003019107145,
-4.082198396148));
#34841=CARTESIAN_POINT('Ctrl Pts',(-9.42743337163542,-166.828019107145,
1.69768315121407E-11));
#34842=CARTESIAN_POINT('Ctrl Pts',(-7.07057502871922,-166.653019107145,
4.08219839617346));
#34843=CARTESIAN_POINT('Ctrl Pts',(-4.71371668580301,-166.478019107145,
8.16439679232994));
#34844=CARTESIAN_POINT('Ctrl Pts',(1.47018674401621E-11,-166.303019107145,
8.16439679232146));
#34845=CARTESIAN_POINT('Ctrl Pts',(4.71371668583241,-166.128019107145,8.16439679231297));
#34846=CARTESIAN_POINT('Ctrl Pts',(7.07057502873392,-165.953019107145,4.082198396148));
#34847=CARTESIAN_POINT('Ctrl Pts',(9.42743337163542,-165.778019107145,-1.69756769845304E-11));
#34848=CARTESIAN_POINT('Ctrl Pts',(7.07057502871922,-165.603019107145,-4.08219839617346));
#34849=CARTESIAN_POINT('Ctrl Pts',(4.71371668580301,-165.428019107145,-8.16439679232994));
#34850=CARTESIAN_POINT('Ctrl Pts',(-1.4702867290402E-11,-165.253019107145,
-8.16439679232146));
#34851=CARTESIAN_POINT('Ctrl Pts',(-4.71371668583241,-165.078019107145,
-8.16439679231297));
#34852=CARTESIAN_POINT('Ctrl Pts',(-7.07057502873392,-164.903019107145,
-4.082198396148));
#34853=CARTESIAN_POINT('Ctrl Pts',(-9.42743337163542,-164.728019107145,
1.69768315121407E-11));
#34854=CARTESIAN_POINT('Ctrl Pts',(-7.07057502871922,-164.553019107145,
4.08219839617346));
#34855=CARTESIAN_POINT('Ctrl Pts',(-4.71371668580301,-164.378019107145,
8.16439679232994));
#34856=CARTESIAN_POINT('Ctrl Pts',(1.47018674401621E-11,-164.203019107145,
8.16439679232146));
#34857=CARTESIAN_POINT('Ctrl Pts',(4.71371668583241,-164.028019107145,8.16439679231297));
#34858=CARTESIAN_POINT('Ctrl Pts',(7.07057502873392,-163.853019107145,4.082198396148));
#34859=CARTESIAN_POINT('Ctrl Pts',(9.42743337163542,-163.678019107145,-1.69756769845304E-11));
#34860=CARTESIAN_POINT('Ctrl Pts',(7.07057502871922,-163.503019107145,-4.08219839617346));
#34861=CARTESIAN_POINT('Ctrl Pts',(4.71371668580301,-163.328019107145,-8.16439679232994));
#34862=CARTESIAN_POINT('Ctrl Pts',(-1.4702867290402E-11,-163.153019107145,
-8.16439679232146));
#34863=CARTESIAN_POINT('Ctrl Pts',(-4.71371668583241,-162.978019107145,
-8.16439679231297));
#34864=CARTESIAN_POINT('Ctrl Pts',(-7.07057502873392,-162.803019107145,
-4.082198396148));
#34865=CARTESIAN_POINT('Ctrl Pts',(-9.42743337163542,-162.628019107145,
1.69768315121407E-11));
#34866=CARTESIAN_POINT('Ctrl Pts',(-7.07057502871922,-162.453019107145,
4.08219839617346));
#34867=CARTESIAN_POINT('Ctrl Pts',(-4.71371668580301,-162.278019107145,
8.16439679232994));
#34868=CARTESIAN_POINT('Ctrl Pts',(1.47018674401621E-11,-162.103019107145,
8.16439679232146));
#34869=CARTESIAN_POINT('Ctrl Pts',(4.71371668583241,-161.928019107145,8.16439679231297));
#34870=CARTESIAN_POINT('Ctrl Pts',(7.07057502873392,-161.753019107145,4.082198396148));
#34871=CARTESIAN_POINT('Ctrl Pts',(9.42743337163542,-161.578019107145,-1.69756769845304E-11));
#34872=CARTESIAN_POINT('Ctrl Pts',(7.07057502871922,-161.403019107145,-4.08219839617346));
#34873=CARTESIAN_POINT('Ctrl Pts',(4.71371668580301,-161.228019107145,-8.16439679232994));
#34874=CARTESIAN_POINT('Ctrl Pts',(-1.4702867290402E-11,-161.053019107145,
-8.16439679232146));
#34875=CARTESIAN_POINT('Ctrl Pts',(-4.71371668583241,-160.878019107145,
-8.16439679231297));
#34876=CARTESIAN_POINT('Ctrl Pts',(-7.07057502873392,-160.703019107145,
-4.082198396148));
#34877=CARTESIAN_POINT('Ctrl Pts',(-9.42743337163542,-160.528019107145,
1.69768315121407E-11));
#34878=CARTESIAN_POINT('Ctrl Pts',(-7.07057502871922,-160.353019107145,
4.08219839617346));
#34879=CARTESIAN_POINT('Ctrl Pts',(-4.71371668580301,-160.178019107145,
8.16439679232994));
#34880=CARTESIAN_POINT('Ctrl Pts',(1.47018674401621E-11,-160.003019107145,
8.16439679232146));
#34881=CARTESIAN_POINT('Ctrl Pts',(4.71371668583241,-159.828019107145,8.16439679231297));
#34882=CARTESIAN_POINT('Ctrl Pts',(7.07057502873392,-159.653019107145,4.082198396148));
#34883=CARTESIAN_POINT('Ctrl Pts',(9.42743337163542,-159.478019107145,-1.69756769845304E-11));
#34884=CARTESIAN_POINT('Ctrl Pts',(7.07057502871922,-159.303019107145,-4.08219839617346));
#34885=CARTESIAN_POINT('Ctrl Pts',(4.71371668580301,-159.128019107145,-8.16439679232994));
#34886=CARTESIAN_POINT('Ctrl Pts',(-1.4702867290402E-11,-158.953019107145,
-8.16439679232146));
#34887=CARTESIAN_POINT('Ctrl Pts',(-4.71371668583241,-158.778019107145,
-8.16439679231297));
#34888=CARTESIAN_POINT('Ctrl Pts',(-7.07057502873392,-158.603019107145,
-4.082198396148));
#34889=CARTESIAN_POINT('Ctrl Pts',(-9.42743337163542,-158.428019107145,
1.69768315121407E-11));
#34890=CARTESIAN_POINT('Ctrl Pts',(-7.07057502871922,-158.253019107145,
4.08219839617346));
#34891=CARTESIAN_POINT('Ctrl Pts',(-4.71371668580301,-158.078019107145,
8.16439679232994));
#34892=CARTESIAN_POINT('Ctrl Pts',(1.47018674401621E-11,-157.903019107145,
8.16439679232146));
#34893=CARTESIAN_POINT('Ctrl Pts',(4.71371668583241,-157.728019107145,8.16439679231297));
#34894=CARTESIAN_POINT('Ctrl Pts',(7.07057502873392,-157.553019107145,4.082198396148));
#34895=CARTESIAN_POINT('Ctrl Pts',(9.42743337163542,-157.378019107145,-1.69756769845304E-11));
#34896=CARTESIAN_POINT('Ctrl Pts',(7.07057502871922,-157.203019107145,-4.08219839617346));
#34897=CARTESIAN_POINT('Ctrl Pts',(4.71371668580301,-157.028019107145,-8.16439679232994));
#34898=CARTESIAN_POINT('Ctrl Pts',(-1.4702867290402E-11,-156.853019107145,
-8.16439679232146));
#34899=CARTESIAN_POINT('Ctrl Pts',(-4.71371668583241,-156.678019107145,
-8.16439679231297));
#34900=CARTESIAN_POINT('Ctrl Pts',(-7.07057502873392,-156.503019107145,
-4.082198396148));
#34901=CARTESIAN_POINT('Ctrl Pts',(-9.42743337163542,-156.328019107145,
1.69768315121407E-11));
#34902=CARTESIAN_POINT('Ctrl Pts',(-7.07057502871922,-156.153019107145,
4.08219839617346));
#34903=CARTESIAN_POINT('Ctrl Pts',(-4.71371668580301,-155.978019107145,
8.16439679232994));
#34904=CARTESIAN_POINT('Ctrl Pts',(1.47018674401621E-11,-155.803019107145,
8.16439679232146));
#34905=CARTESIAN_POINT('Ctrl Pts',(4.71371668583241,-155.628019107145,8.16439679231297));
#34906=CARTESIAN_POINT('Ctrl Pts',(7.07057502873392,-155.453019107145,4.082198396148));
#34907=CARTESIAN_POINT('Ctrl Pts',(9.42743337163542,-155.278019107145,-1.69756769845304E-11));
#34908=CARTESIAN_POINT('Ctrl Pts',(7.07057502871922,-155.103019107145,-4.08219839617346));
#34909=CARTESIAN_POINT('Ctrl Pts',(4.71371668580301,-154.928019107145,-8.16439679232994));
#34910=CARTESIAN_POINT('Ctrl Pts',(-1.4702867290402E-11,-154.753019107145,
-8.16439679232146));
#34911=CARTESIAN_POINT('Ctrl Pts',(-4.71371668583241,-154.578019107145,
-8.16439679231297));
#34912=CARTESIAN_POINT('Ctrl Pts',(-7.07057502873392,-154.403019107145,
-4.082198396148));
#34913=CARTESIAN_POINT('Ctrl Pts',(-9.42743337163542,-154.228019107145,
1.69768315121407E-11));
#34914=CARTESIAN_POINT('Ctrl Pts',(-7.07057502871922,-154.053019107145,
4.08219839617346));
#34915=CARTESIAN_POINT('Ctrl Pts',(-4.71371668580301,-153.878019107145,
8.16439679232994));
#34916=CARTESIAN_POINT('Ctrl Pts',(1.47018674401621E-11,-153.703019107145,
8.16439679232146));
#34917=CARTESIAN_POINT('Ctrl Pts',(4.71371668583241,-153.528019107145,8.16439679231297));
#34918=CARTESIAN_POINT('Ctrl Pts',(7.07057502873392,-153.353019107145,4.082198396148));
#34919=CARTESIAN_POINT('Ctrl Pts',(9.42743337163542,-153.178019107145,-1.69756769845304E-11));
#34920=CARTESIAN_POINT('Ctrl Pts',(7.07057502871922,-153.003019107145,-4.08219839617346));
#34921=CARTESIAN_POINT('Ctrl Pts',(4.71371668580301,-152.828019107145,-8.16439679232994));
#34922=CARTESIAN_POINT('Ctrl Pts',(-1.4702867290402E-11,-152.653019107145,
-8.16439679232146));
#34923=CARTESIAN_POINT('Ctrl Pts',(-4.71371668583241,-152.478019107145,
-8.16439679231297));
#34924=CARTESIAN_POINT('Ctrl Pts',(-7.07057502873392,-152.303019107145,
-4.082198396148));
#34925=CARTESIAN_POINT('Ctrl Pts',(-9.42743337163542,-152.128019107145,
1.69768315121407E-11));
#34926=CARTESIAN_POINT('Ctrl Pts',(-7.07057502871922,-151.953019107145,
4.08219839617346));
#34927=CARTESIAN_POINT('Ctrl Pts',(-4.71371668580301,-151.778019107145,
8.16439679232994));
#34928=CARTESIAN_POINT('Ctrl Pts',(1.47018674401621E-11,-151.603019107145,
8.16439679232146));
#34929=CARTESIAN_POINT('Ctrl Pts',(4.71371668583241,-151.428019107145,8.16439679231297));
#34930=CARTESIAN_POINT('Ctrl Pts',(7.07057502873392,-151.253019107145,4.082198396148));
#34931=CARTESIAN_POINT('Ctrl Pts',(9.42743337163542,-151.078019107145,-1.69756769845304E-11));
#34932=CARTESIAN_POINT('Ctrl Pts',(7.07057502871922,-150.903019107145,-4.08219839617346));
#34933=CARTESIAN_POINT('Ctrl Pts',(4.71371668580301,-150.728019107145,-8.16439679232994));
#34934=CARTESIAN_POINT('Ctrl Pts',(-1.4702867290402E-11,-150.553019107145,
-8.16439679232146));
#34935=CARTESIAN_POINT('Ctrl Pts',(-4.71371668583241,-150.378019107145,
-8.16439679231297));
#34936=CARTESIAN_POINT('Ctrl Pts',(-7.07057502873392,-150.203019107145,
-4.082198396148));
#34937=CARTESIAN_POINT('Ctrl Pts',(-9.42743337163542,-150.028019107145,
1.69768315121407E-11));
#34938=CARTESIAN_POINT('Ctrl Pts',(-7.07057502871922,-149.853019107145,
4.08219839617346));
#34939=CARTESIAN_POINT('Ctrl Pts',(-4.71371668580301,-149.678019107145,
8.16439679232994));
#34940=CARTESIAN_POINT('Ctrl Pts',(1.47018674401621E-11,-149.503019107145,
8.16439679232146));
#34941=CARTESIAN_POINT('Ctrl Pts',(4.71371668583241,-149.328019107145,8.16439679231297));
#34942=CARTESIAN_POINT('Ctrl Pts',(7.07057502873392,-149.153019107145,4.082198396148));
#34943=CARTESIAN_POINT('Ctrl Pts',(9.42743337163542,-148.978019107145,-1.69756769845304E-11));
#34944=CARTESIAN_POINT('Ctrl Pts',(7.07057502871922,-148.803019107145,-4.08219839617346));
#34945=CARTESIAN_POINT('Ctrl Pts',(4.71371668580301,-148.628019107145,-8.16439679232994));
#34946=CARTESIAN_POINT('Ctrl Pts',(-1.4702867290402E-11,-148.453019107145,
-8.16439679232146));
#34947=CARTESIAN_POINT('Ctrl Pts',(-4.71371668583241,-148.278019107145,
-8.16439679231297));
#34948=CARTESIAN_POINT('Ctrl Pts',(-7.07057502873392,-148.103019107145,
-4.082198396148));
#34949=CARTESIAN_POINT('Ctrl Pts',(-9.42743337163542,-147.928019107145,
1.69768315121407E-11));
#34950=CARTESIAN_POINT('Ctrl Pts',(-7.07057502871922,-147.753019107145,
4.08219839617346));
#34951=CARTESIAN_POINT('Ctrl Pts',(-4.71371668580301,-147.578019107145,
8.16439679232994));
#34952=CARTESIAN_POINT('Ctrl Pts',(1.47018674401621E-11,-147.403019107145,
8.16439679232146));
#34953=CARTESIAN_POINT('Ctrl Pts',(4.71371668583241,-147.228019107145,8.16439679231297));
#34954=CARTESIAN_POINT('Ctrl Pts',(7.07057502873392,-147.053019107145,4.082198396148));
#34955=CARTESIAN_POINT('Ctrl Pts',(9.42743337163542,-146.878019107145,-1.69756769845304E-11));
#34956=CARTESIAN_POINT('Ctrl Pts',(7.07057502871922,-146.703019107145,-4.08219839617346));
#34957=CARTESIAN_POINT('Ctrl Pts',(4.71371668580301,-146.528019107145,-8.16439679232994));
#34958=CARTESIAN_POINT('Ctrl Pts',(-1.4702867290402E-11,-146.353019107145,
-8.16439679232146));
#34959=CARTESIAN_POINT('Ctrl Pts',(-4.71371668583241,-146.178019107145,
-8.16439679231297));
#34960=CARTESIAN_POINT('Ctrl Pts',(-7.07057502873392,-146.003019107145,
-4.082198396148));
#34961=CARTESIAN_POINT('Ctrl Pts',(-9.42743337163542,-145.828019107145,
1.69768315121407E-11));
#34962=CARTESIAN_POINT('Ctrl Pts',(-7.07057502871922,-145.653019107145,
4.08219839617346));
#34963=CARTESIAN_POINT('Ctrl Pts',(-4.71371668580301,-145.478019107145,
8.16439679232994));
#34964=CARTESIAN_POINT('Ctrl Pts',(1.47018674401621E-11,-145.303019107145,
8.16439679232146));
#34965=CARTESIAN_POINT('Ctrl Pts',(4.71371668583241,-145.128019107145,8.16439679231297));
#34966=CARTESIAN_POINT('Ctrl Pts',(7.07057502873392,-144.953019107145,4.082198396148));
#34967=CARTESIAN_POINT('Ctrl Pts',(9.42743337163542,-144.778019107145,-1.69756769845304E-11));
#34968=CARTESIAN_POINT('Ctrl Pts',(7.07057502871922,-144.603019107145,-4.08219839617346));
#34969=CARTESIAN_POINT('Ctrl Pts',(4.71371668580301,-144.428019107145,-8.16439679232994));
#34970=CARTESIAN_POINT('Ctrl Pts',(-1.4702867290402E-11,-144.253019107145,
-8.16439679232146));
#34971=CARTESIAN_POINT('Ctrl Pts',(-4.71371668583241,-144.078019107145,
-8.16439679231297));
#34972=CARTESIAN_POINT('Ctrl Pts',(-7.07057502873392,-143.903019107145,
-4.082198396148));
#34973=CARTESIAN_POINT('Ctrl Pts',(-9.42743337163542,-143.728019107145,
1.69768315121407E-11));
#34974=CARTESIAN_POINT('Ctrl Pts',(-7.07057502871922,-143.553019107145,
4.08219839617346));
#34975=CARTESIAN_POINT('Ctrl Pts',(-4.71371668580301,-143.378019107145,
8.16439679232994));
#34976=CARTESIAN_POINT('Ctrl Pts',(1.47018674401621E-11,-143.203019107145,
8.16439679232146));
#34977=CARTESIAN_POINT('Ctrl Pts',(4.71371668583241,-143.028019107145,8.16439679231297));
#34978=CARTESIAN_POINT('Ctrl Pts',(7.07057502873392,-142.853019107145,4.082198396148));
#34979=CARTESIAN_POINT('Ctrl Pts',(9.42743337163542,-142.678019107145,-1.69756769845304E-11));
#34980=CARTESIAN_POINT('Ctrl Pts',(7.07057502871922,-142.503019107145,-4.08219839617346));
#34981=CARTESIAN_POINT('Ctrl Pts',(4.71371668580301,-142.328019107145,-8.16439679232994));
#34982=CARTESIAN_POINT('Ctrl Pts',(-1.4702867290402E-11,-142.153019107145,
-8.16439679232146));
#34983=CARTESIAN_POINT('Ctrl Pts',(-4.71371668583241,-141.978019107145,
-8.16439679231297));
#34984=CARTESIAN_POINT('Ctrl Pts',(-7.07057502873392,-141.803019107145,
-4.082198396148));
#34985=CARTESIAN_POINT('Ctrl Pts',(-9.42743337163542,-141.628019107145,
1.69768315121407E-11));
#34986=CARTESIAN_POINT('Ctrl Pts',(-7.07057502871922,-141.453019107145,
4.08219839617346));
#34987=CARTESIAN_POINT('Ctrl Pts',(-4.71371668580301,-141.278019107145,
8.16439679232994));
#34988=CARTESIAN_POINT('Ctrl Pts',(1.47018674401621E-11,-141.103019107145,
8.16439679232146));
#34989=CARTESIAN_POINT('Ctrl Pts',(4.71371668583241,-140.928019107145,8.16439679231297));
#34990=CARTESIAN_POINT('Ctrl Pts',(7.07057502873392,-140.753019107145,4.082198396148));
#34991=CARTESIAN_POINT('Ctrl Pts',(9.42743337163542,-140.578019107145,-1.69756769845304E-11));
#34992=CARTESIAN_POINT('Ctrl Pts',(7.07057502871922,-140.403019107145,-4.08219839617346));
#34993=CARTESIAN_POINT('Ctrl Pts',(4.71371668580301,-140.228019107145,-8.16439679232994));
#34994=CARTESIAN_POINT('Ctrl Pts',(-1.4702867290402E-11,-140.053019107145,
-8.16439679232146));
#34995=CARTESIAN_POINT('Ctrl Pts',(-4.71371668583241,-139.878019107145,
-8.16439679231297));
#34996=CARTESIAN_POINT('Ctrl Pts',(-7.07057502873392,-139.703019107145,
-4.082198396148));
#34997=CARTESIAN_POINT('Ctrl Pts',(-9.42743337163542,-139.528019107145,
1.69768315121407E-11));
#34998=CARTESIAN_POINT('Ctrl Pts',(-7.07057502871922,-139.353019107145,
4.08219839617346));
#34999=CARTESIAN_POINT('Ctrl Pts',(-4.71371668580301,-139.178019107145,
8.16439679232994));
#35000=CARTESIAN_POINT('Ctrl Pts',(1.47018674401621E-11,-139.003019107145,
8.16439679232146));
#35001=CARTESIAN_POINT('Ctrl Pts',(4.71371668583241,-138.828019107145,8.16439679231297));
#35002=CARTESIAN_POINT('Ctrl Pts',(7.07057502873392,-138.653019107145,4.082198396148));
#35003=CARTESIAN_POINT('Ctrl Pts',(9.42743337163542,-138.478019107145,-1.69756769845304E-11));
#35004=CARTESIAN_POINT('Ctrl Pts',(7.07057502871922,-138.303019107145,-4.08219839617346));
#35005=CARTESIAN_POINT('Ctrl Pts',(4.71371668580301,-138.128019107145,-8.16439679232994));
#35006=CARTESIAN_POINT('Ctrl Pts',(-1.4702867290402E-11,-137.953019107145,
-8.16439679232146));
#35007=CARTESIAN_POINT('Ctrl Pts',(-4.71371668583241,-137.778019107145,
-8.16439679231297));
#35008=CARTESIAN_POINT('Ctrl Pts',(-7.07057502873392,-137.603019107145,
-4.082198396148));
#35009=CARTESIAN_POINT('Ctrl Pts',(-9.42743337163542,-137.428019107145,
1.69768315121407E-11));
#35010=CARTESIAN_POINT('Ctrl Pts',(-7.07057502871922,-137.253019107145,
4.08219839617346));
#35011=CARTESIAN_POINT('Ctrl Pts',(-4.71371668580301,-137.078019107145,
8.16439679232994));
#35012=CARTESIAN_POINT('Ctrl Pts',(1.47018674401621E-11,-136.903019107145,
8.16439679232146));
#35013=CARTESIAN_POINT('Ctrl Pts',(4.71371668583241,-136.728019107145,8.16439679231297));
#35014=CARTESIAN_POINT('Ctrl Pts',(7.07057502873392,-136.553019107145,4.082198396148));
#35015=CARTESIAN_POINT('Ctrl Pts',(9.42743337163542,-136.378019107145,-1.69756769845304E-11));
#35016=CARTESIAN_POINT('Ctrl Pts',(7.07057502871922,-136.203019107145,-4.08219839617346));
#35017=CARTESIAN_POINT('Ctrl Pts',(4.71371668580301,-136.028019107145,-8.16439679232994));
#35018=CARTESIAN_POINT('Ctrl Pts',(-1.4702867290402E-11,-135.853019107145,
-8.16439679232146));
#35019=CARTESIAN_POINT('Ctrl Pts',(-4.71371668583241,-135.678019107145,
-8.16439679231297));
#35020=CARTESIAN_POINT('Ctrl Pts',(-7.07057502873392,-135.503019107145,
-4.082198396148));
#35021=CARTESIAN_POINT('Ctrl Pts',(-9.42743337163542,-135.328019107145,
1.69768315121407E-11));
#35022=CARTESIAN_POINT('Ctrl Pts',(-7.07057502871922,-135.153019107145,
4.08219839617346));
#35023=CARTESIAN_POINT('Ctrl Pts',(-4.71371668580301,-134.978019107145,
8.16439679232994));
#35024=CARTESIAN_POINT('Ctrl Pts',(1.47018674401621E-11,-134.803019107145,
8.16439679232146));
#35025=CARTESIAN_POINT('Ctrl Pts',(4.71371668583241,-134.628019107145,8.16439679231297));
#35026=CARTESIAN_POINT('Ctrl Pts',(7.07057502873392,-134.453019107145,4.082198396148));
#35027=CARTESIAN_POINT('Ctrl Pts',(9.42743337163542,-134.278019107145,-1.69756769845304E-11));
#35028=CARTESIAN_POINT('Ctrl Pts',(7.07057502871922,-134.103019107145,-4.08219839617346));
#35029=CARTESIAN_POINT('Ctrl Pts',(4.71371668580301,-133.928019107145,-8.16439679232994));
#35030=CARTESIAN_POINT('Ctrl Pts',(-1.4702867290402E-11,-133.753019107145,
-8.16439679232146));
#35031=CARTESIAN_POINT('Ctrl Pts',(-4.71371668583241,-133.578019107145,
-8.16439679231297));
#35032=CARTESIAN_POINT('Ctrl Pts',(-7.07057502873392,-133.403019107145,
-4.082198396148));
#35033=CARTESIAN_POINT('Ctrl Pts',(-9.42743337163542,-133.228019107145,
1.69768315121407E-11));
#35034=CARTESIAN_POINT('Ctrl Pts',(-7.07057502871922,-133.053019107145,
4.08219839617346));
#35035=CARTESIAN_POINT('Ctrl Pts',(-4.71371668580301,-132.878019107145,
8.16439679232994));
#35036=CARTESIAN_POINT('Ctrl Pts',(1.47018674401621E-11,-132.703019107145,
8.16439679232146));
#35037=CARTESIAN_POINT('Ctrl Pts',(4.71371668583241,-132.528019107145,8.16439679231297));
#35038=CARTESIAN_POINT('Ctrl Pts',(7.07057502873392,-132.353019107145,4.082198396148));
#35039=CARTESIAN_POINT('Ctrl Pts',(9.42743337163542,-132.178019107145,-1.69756769845304E-11));
#35040=CARTESIAN_POINT('Ctrl Pts',(7.07057502871922,-132.003019107145,-4.08219839617346));
#35041=CARTESIAN_POINT('Ctrl Pts',(4.71371668580301,-131.828019107145,-8.16439679232994));
#35042=CARTESIAN_POINT('Ctrl Pts',(-1.4702867290402E-11,-131.653019107145,
-8.16439679232146));
#35043=CARTESIAN_POINT('Ctrl Pts',(-4.71371668583241,-131.478019107145,
-8.16439679231297));
#35044=CARTESIAN_POINT('Ctrl Pts',(-7.07057502873392,-131.303019107145,
-4.082198396148));
#35045=CARTESIAN_POINT('Ctrl Pts',(-9.42743337163542,-131.128019107145,
1.69768315121407E-11));
#35046=CARTESIAN_POINT('Ctrl Pts',(-7.07057502871922,-130.953019107145,
4.08219839617346));
#35047=CARTESIAN_POINT('Ctrl Pts',(-4.71371668580301,-130.778019107145,
8.16439679232994));
#35048=CARTESIAN_POINT('Ctrl Pts',(1.47018674401621E-11,-130.603019107145,
8.16439679232146));
#35049=CARTESIAN_POINT('Ctrl Pts',(4.71371668583241,-130.428019107145,8.16439679231297));
#35050=CARTESIAN_POINT('Ctrl Pts',(7.07057502873392,-130.253019107145,4.082198396148));
#35051=CARTESIAN_POINT('Ctrl Pts',(9.42743337163542,-130.078019107145,-1.69756769845304E-11));
#35052=CARTESIAN_POINT('Ctrl Pts',(7.07057502871922,-129.903019107145,-4.08219839617346));
#35053=CARTESIAN_POINT('Ctrl Pts',(4.71371668580301,-129.728019107145,-8.16439679232994));
#35054=CARTESIAN_POINT('Ctrl Pts',(-1.4702867290402E-11,-129.553019107145,
-8.16439679232146));
#35055=CARTESIAN_POINT('Ctrl Pts',(-4.71371668583241,-129.378019107145,
-8.16439679231297));
#35056=CARTESIAN_POINT('Ctrl Pts',(-7.07057502873392,-129.203019107145,
-4.082198396148));
#35057=CARTESIAN_POINT('Ctrl Pts',(-9.42743337163542,-129.028019107145,
1.69768315121407E-11));
#35058=CARTESIAN_POINT('Ctrl Pts',(-7.07057502871922,-128.853019107145,
4.08219839617346));
#35059=CARTESIAN_POINT('Ctrl Pts',(-4.71371668580301,-128.678019107145,
8.16439679232994));
#35060=CARTESIAN_POINT('Ctrl Pts',(1.47018674401621E-11,-128.503019107145,
8.16439679232146));
#35061=CARTESIAN_POINT('Ctrl Pts',(4.71371668583241,-128.328019107145,8.16439679231297));
#35062=CARTESIAN_POINT('Ctrl Pts',(7.07057502873392,-128.153019107145,4.082198396148));
#35063=CARTESIAN_POINT('Ctrl Pts',(9.42743337163542,-127.978019107145,-1.69756769845304E-11));
#35064=CARTESIAN_POINT('Ctrl Pts',(7.07057502871922,-127.803019107145,-4.08219839617346));
#35065=CARTESIAN_POINT('Ctrl Pts',(4.71371668580301,-127.628019107145,-8.16439679232994));
#35066=CARTESIAN_POINT('Ctrl Pts',(-1.4702867290402E-11,-127.453019107145,
-8.16439679232146));
#35067=CARTESIAN_POINT('Ctrl Pts',(-4.71371668583241,-127.278019107145,
-8.16439679231297));
#35068=CARTESIAN_POINT('Ctrl Pts',(-7.07057502873392,-127.103019107145,
-4.082198396148));
#35069=CARTESIAN_POINT('Ctrl Pts',(-9.42743337163542,-126.928019107145,
1.69768315121407E-11));
#35070=CARTESIAN_POINT('Ctrl Pts',(-7.07057502871922,-126.753019107145,
4.08219839617346));
#35071=CARTESIAN_POINT('Ctrl Pts',(-4.71371668580301,-126.578019107145,
8.16439679232994));
#35072=CARTESIAN_POINT('Ctrl Pts',(1.47018674401621E-11,-126.403019107145,
8.16439679232146));
#35073=CARTESIAN_POINT('Ctrl Pts',(4.71371668583241,-126.228019107145,8.16439679231297));
#35074=CARTESIAN_POINT('Ctrl Pts',(7.07057502873392,-126.053019107145,4.082198396148));
#35075=CARTESIAN_POINT('Ctrl Pts',(9.42743337163542,-125.878019107145,-1.69756769845304E-11));
#35076=CARTESIAN_POINT('Ctrl Pts',(7.07057502871922,-125.703019107145,-4.08219839617346));
#35077=CARTESIAN_POINT('Ctrl Pts',(4.71371668580301,-125.528019107145,-8.16439679232994));
#35078=CARTESIAN_POINT('Ctrl Pts',(-1.4702867290402E-11,-125.353019107145,
-8.16439679232146));
#35079=CARTESIAN_POINT('Ctrl Pts',(-4.71371668583241,-125.178019107145,
-8.16439679231297));
#35080=CARTESIAN_POINT('Ctrl Pts',(-7.07057502873392,-125.003019107145,
-4.082198396148));
#35081=CARTESIAN_POINT('Ctrl Pts',(-9.42743337163542,-124.828019107145,
1.69768315121407E-11));
#35082=CARTESIAN_POINT('Ctrl Pts',(-7.07057502871922,-124.653019107145,
4.08219839617346));
#35083=CARTESIAN_POINT('Ctrl Pts',(-4.71371668580301,-124.478019107145,
8.16439679232994));
#35084=CARTESIAN_POINT('Ctrl Pts',(1.47018674401621E-11,-124.303019107145,
8.16439679232146));
#35085=CARTESIAN_POINT('Ctrl Pts',(4.71371668583241,-124.128019107145,8.16439679231297));
#35086=CARTESIAN_POINT('Ctrl Pts',(7.07057502873392,-123.953019107145,4.082198396148));
#35087=CARTESIAN_POINT('Ctrl Pts',(9.42743337163542,-123.778019107145,-1.69756769845304E-11));
#35088=CARTESIAN_POINT('Ctrl Pts',(7.07057502871922,-123.603019107145,-4.08219839617346));
#35089=CARTESIAN_POINT('Ctrl Pts',(4.71371668580301,-123.428019107145,-8.16439679232994));
#35090=CARTESIAN_POINT('Ctrl Pts',(-1.4702867290402E-11,-123.253019107145,
-8.16439679232146));
#35091=CARTESIAN_POINT('Ctrl Pts',(-4.71371668583241,-123.078019107145,
-8.16439679231297));
#35092=CARTESIAN_POINT('Ctrl Pts',(-7.07057502873392,-122.903019107145,
-4.082198396148));
#35093=CARTESIAN_POINT('Ctrl Pts',(-9.42743337163542,-122.728019107145,
1.69768315121407E-11));
#35094=CARTESIAN_POINT('Ctrl Pts',(-7.07057502871922,-122.553019107145,
4.08219839617346));
#35095=CARTESIAN_POINT('Ctrl Pts',(-4.71371668580301,-122.378019107145,
8.16439679232994));
#35096=CARTESIAN_POINT('Ctrl Pts',(1.47018674401621E-11,-122.203019107145,
8.16439679232146));
#35097=CARTESIAN_POINT('Ctrl Pts',(4.71371668583241,-122.028019107145,8.16439679231297));
#35098=CARTESIAN_POINT('Ctrl Pts',(7.07057502873392,-121.853019107145,4.082198396148));
#35099=CARTESIAN_POINT('Ctrl Pts',(9.42743337163542,-121.678019107145,-1.69756769845304E-11));
#35100=CARTESIAN_POINT('Ctrl Pts',(7.07057502871922,-121.503019107145,-4.08219839617346));
#35101=CARTESIAN_POINT('Ctrl Pts',(4.71371668580301,-121.328019107145,-8.16439679232994));
#35102=CARTESIAN_POINT('Ctrl Pts',(-1.4702867290402E-11,-121.153019107145,
-8.16439679232146));
#35103=CARTESIAN_POINT('Ctrl Pts',(-4.71371668583241,-120.978019107145,
-8.16439679231297));
#35104=CARTESIAN_POINT('Ctrl Pts',(-7.07057502873392,-120.803019107145,
-4.082198396148));
#35105=CARTESIAN_POINT('Ctrl Pts',(-9.42743337163542,-120.628019107145,
1.69768315121407E-11));
#35106=CARTESIAN_POINT('Ctrl Pts',(-7.07057502871922,-120.453019107145,
4.08219839617346));
#35107=CARTESIAN_POINT('Ctrl Pts',(-4.71371668580301,-120.278019107145,
8.16439679232994));
#35108=CARTESIAN_POINT('Ctrl Pts',(1.47018674401621E-11,-120.103019107145,
8.16439679232146));
#35109=CARTESIAN_POINT('Ctrl Pts',(4.71371668583241,-119.928019107145,8.16439679231297));
#35110=CARTESIAN_POINT('Ctrl Pts',(7.07057502873392,-119.753019107145,4.082198396148));
#35111=CARTESIAN_POINT('Ctrl Pts',(9.42743337163542,-119.578019107145,-1.69756769845304E-11));
#35112=CARTESIAN_POINT('Ctrl Pts',(7.07057502871922,-119.403019107145,-4.08219839617346));
#35113=CARTESIAN_POINT('Ctrl Pts',(4.71371668580301,-119.228019107145,-8.16439679232994));
#35114=CARTESIAN_POINT('Ctrl Pts',(-1.4702867290402E-11,-119.053019107145,
-8.16439679232146));
#35115=CARTESIAN_POINT('Ctrl Pts',(-4.71371668583241,-118.878019107145,
-8.16439679231297));
#35116=CARTESIAN_POINT('Ctrl Pts',(-7.07057502873392,-118.703019107145,
-4.082198396148));
#35117=CARTESIAN_POINT('Ctrl Pts',(-9.42743337163542,-118.528019107145,
1.69768315121407E-11));
#35118=CARTESIAN_POINT('Ctrl Pts',(-7.07057502871922,-118.353019107145,
4.08219839617346));
#35119=CARTESIAN_POINT('Ctrl Pts',(-4.71371668580301,-118.178019107145,
8.16439679232994));
#35120=CARTESIAN_POINT('Ctrl Pts',(1.47018674401621E-11,-118.003019107145,
8.16439679232146));
#35121=CARTESIAN_POINT('Ctrl Pts',(4.71371668583241,-117.828019107145,8.16439679231297));
#35122=CARTESIAN_POINT('Ctrl Pts',(7.07057502873392,-117.653019107145,4.082198396148));
#35123=CARTESIAN_POINT('Ctrl Pts',(9.42743337163542,-117.478019107145,-1.69756769845304E-11));
#35124=CARTESIAN_POINT('Ctrl Pts',(7.07057502871922,-117.303019107145,-4.08219839617346));
#35125=CARTESIAN_POINT('Ctrl Pts',(4.71371668580301,-117.128019107145,-8.16439679232994));
#35126=CARTESIAN_POINT('Ctrl Pts',(-1.4702867290402E-11,-116.953019107145,
-8.16439679232146));
#35127=CARTESIAN_POINT('Ctrl Pts',(-4.71371668583241,-116.778019107145,
-8.16439679231297));
#35128=CARTESIAN_POINT('Ctrl Pts',(-7.07057502873392,-116.603019107145,
-4.082198396148));
#35129=CARTESIAN_POINT('Ctrl Pts',(-9.42743337163542,-116.428019107145,
1.69768315121407E-11));
#35130=CARTESIAN_POINT('Ctrl Pts',(-7.07057502871922,-116.253019107145,
4.08219839617346));
#35131=CARTESIAN_POINT('Ctrl Pts',(-4.71371668580301,-116.078019107145,
8.16439679232994));
#35132=CARTESIAN_POINT('Ctrl Pts',(1.47018674401621E-11,-115.903019107145,
8.16439679232146));
#35133=CARTESIAN_POINT('Ctrl Pts',(4.71371668583241,-115.728019107145,8.16439679231297));
#35134=CARTESIAN_POINT('Ctrl Pts',(7.07057502873392,-115.553019107145,4.082198396148));
#35135=CARTESIAN_POINT('Ctrl Pts',(9.42743337163542,-115.378019107145,-1.69756769845304E-11));
#35136=CARTESIAN_POINT('Ctrl Pts',(7.07057502871922,-115.203019107145,-4.08219839617346));
#35137=CARTESIAN_POINT('Ctrl Pts',(4.71371668580301,-115.028019107145,-8.16439679232994));
#35138=CARTESIAN_POINT('Ctrl Pts',(-1.4702867290402E-11,-114.853019107145,
-8.16439679232146));
#35139=CARTESIAN_POINT('Ctrl Pts',(-4.71371668583241,-114.678019107145,
-8.16439679231297));
#35140=CARTESIAN_POINT('Ctrl Pts',(-7.07057502873392,-114.503019107145,
-4.082198396148));
#35141=CARTESIAN_POINT('Ctrl Pts',(-9.42743337163542,-114.328019107145,
1.69768315121407E-11));
#35142=CARTESIAN_POINT('Ctrl Pts',(-7.07057502871922,-114.153019107145,
4.08219839617346));
#35143=CARTESIAN_POINT('Ctrl Pts',(-4.71371668580301,-113.978019107145,
8.16439679232994));
#35144=CARTESIAN_POINT('Ctrl Pts',(1.47018674401621E-11,-113.803019107145,
8.16439679232146));
#35145=CARTESIAN_POINT('Ctrl Pts',(4.71371668583241,-113.628019107145,8.16439679231297));
#35146=CARTESIAN_POINT('Ctrl Pts',(7.07057502873392,-113.453019107145,4.082198396148));
#35147=CARTESIAN_POINT('Ctrl Pts',(9.42743337163542,-113.278019107145,-1.69756769845304E-11));
#35148=CARTESIAN_POINT('Ctrl Pts',(7.07057502871922,-113.103019107145,-4.08219839617346));
#35149=CARTESIAN_POINT('Ctrl Pts',(4.71371668580301,-112.928019107145,-8.16439679232994));
#35150=CARTESIAN_POINT('Ctrl Pts',(-1.4702867290402E-11,-112.753019107145,
-8.16439679232146));
#35151=CARTESIAN_POINT('Ctrl Pts',(-4.71371668583241,-112.578019107145,
-8.16439679231297));
#35152=CARTESIAN_POINT('Ctrl Pts',(-7.07057502873392,-112.403019107145,
-4.082198396148));
#35153=CARTESIAN_POINT('Ctrl Pts',(-9.42743337163542,-112.228019107145,
1.69768315121407E-11));
#35154=CARTESIAN_POINT('Ctrl Pts',(-7.07057502871922,-112.053019107145,
4.08219839617346));
#35155=CARTESIAN_POINT('Ctrl Pts',(-4.71371668580301,-111.878019107145,
8.16439679232994));
#35156=CARTESIAN_POINT('Ctrl Pts',(1.47018674401621E-11,-111.703019107145,
8.16439679232146));
#35157=CARTESIAN_POINT('Ctrl Pts',(4.71371668583241,-111.528019107145,8.16439679231297));
#35158=CARTESIAN_POINT('Ctrl Pts',(7.07057502873392,-111.353019107145,4.082198396148));
#35159=CARTESIAN_POINT('Ctrl Pts',(9.42743337163542,-111.178019107145,-1.69756769845304E-11));
#35160=CARTESIAN_POINT('Ctrl Pts',(7.07057502871922,-111.003019107145,-4.08219839617346));
#35161=CARTESIAN_POINT('Ctrl Pts',(4.71371668580301,-110.828019107145,-8.16439679232994));
#35162=CARTESIAN_POINT('Ctrl Pts',(-1.4702867290402E-11,-110.653019107145,
-8.16439679232146));
#35163=CARTESIAN_POINT('Ctrl Pts',(-4.71371668583241,-110.478019107145,
-8.16439679231297));
#35164=CARTESIAN_POINT('Ctrl Pts',(-7.07057502873392,-110.303019107145,
-4.082198396148));
#35165=CARTESIAN_POINT('Ctrl Pts',(-9.42743337163542,-110.128019107145,
1.69768315121407E-11));
#35166=CARTESIAN_POINT('Ctrl Pts',(-7.07057502871922,-109.953019107145,
4.08219839617346));
#35167=CARTESIAN_POINT('Ctrl Pts',(-4.71371668580301,-109.778019107145,
8.16439679232994));
#35168=CARTESIAN_POINT('Ctrl Pts',(1.47018674401621E-11,-109.603019107145,
8.16439679232146));
#35169=CARTESIAN_POINT('Ctrl Pts',(4.71371668583241,-109.428019107145,8.16439679231297));
#35170=CARTESIAN_POINT('Ctrl Pts',(7.07057502873392,-109.253019107145,4.082198396148));
#35171=CARTESIAN_POINT('Ctrl Pts',(9.42743337163542,-109.078019107145,-1.69756769845304E-11));
#35172=CARTESIAN_POINT('Ctrl Pts',(7.07057502871922,-108.903019107145,-4.08219839617346));
#35173=CARTESIAN_POINT('Ctrl Pts',(4.71371668580301,-108.728019107145,-8.16439679232994));
#35174=CARTESIAN_POINT('Ctrl Pts',(-1.4702867290402E-11,-108.553019107145,
-8.16439679232146));
#35175=CARTESIAN_POINT('Ctrl Pts',(-4.71371668583241,-108.378019107145,
-8.16439679231297));
#35176=CARTESIAN_POINT('Ctrl Pts',(-7.07057502873392,-108.203019107145,
-4.082198396148));
#35177=CARTESIAN_POINT('Ctrl Pts',(-9.42743337163542,-108.028019107145,
1.69768315121407E-11));
#35178=CARTESIAN_POINT('Ctrl Pts',(-7.07057502871922,-107.853019107145,
4.08219839617346));
#35179=CARTESIAN_POINT('Ctrl Pts',(-4.71371668580301,-107.678019107145,
8.16439679232994));
#35180=CARTESIAN_POINT('Ctrl Pts',(1.47018674401621E-11,-107.503019107145,
8.16439679232146));
#35181=CARTESIAN_POINT('Ctrl Pts',(4.71371668583241,-107.328019107145,8.16439679231297));
#35182=CARTESIAN_POINT('Ctrl Pts',(7.07057502873392,-107.153019107145,4.082198396148));
#35183=CARTESIAN_POINT('Ctrl Pts',(9.42743337163542,-106.978019107145,-1.69756769845304E-11));
#35184=CARTESIAN_POINT('Ctrl Pts',(7.07057502871922,-106.803019107145,-4.08219839617346));
#35185=CARTESIAN_POINT('Ctrl Pts',(4.71371668580301,-106.628019107145,-8.16439679232994));
#35186=CARTESIAN_POINT('Ctrl Pts',(-1.4702867290402E-11,-106.453019107145,
-8.16439679232146));
#35187=CARTESIAN_POINT('Ctrl Pts',(-4.71371668583241,-106.278019107145,
-8.16439679231297));
#35188=CARTESIAN_POINT('Ctrl Pts',(-7.07057502873392,-106.103019107145,
-4.082198396148));
#35189=CARTESIAN_POINT('Ctrl Pts',(-9.42743337163542,-105.928019107145,
1.69768315121407E-11));
#35190=CARTESIAN_POINT('Ctrl Pts',(-7.07057502871922,-105.753019107145,
4.08219839617346));
#35191=CARTESIAN_POINT('Ctrl Pts',(-4.71371668580301,-105.578019107145,
8.16439679232994));
#35192=CARTESIAN_POINT('Ctrl Pts',(1.47018674401621E-11,-105.403019107145,
8.16439679232146));
#35193=CARTESIAN_POINT('Ctrl Pts',(4.71371668583241,-105.228019107145,8.16439679231297));
#35194=CARTESIAN_POINT('Ctrl Pts',(7.07057502873392,-105.053019107145,4.082198396148));
#35195=CARTESIAN_POINT('Ctrl Pts',(9.42743337163542,-104.878019107145,-1.69756769845304E-11));
#35196=CARTESIAN_POINT('Ctrl Pts',(7.07057502871922,-104.703019107145,-4.08219839617346));
#35197=CARTESIAN_POINT('Ctrl Pts',(4.71371668580301,-104.528019107145,-8.16439679232994));
#35198=CARTESIAN_POINT('Ctrl Pts',(-1.4702867290402E-11,-104.353019107145,
-8.16439679232146));
#35199=CARTESIAN_POINT('Ctrl Pts',(-4.71371668583241,-104.178019107145,
-8.16439679231297));
#35200=CARTESIAN_POINT('Ctrl Pts',(-7.07057502873392,-104.003019107145,
-4.082198396148));
#35201=CARTESIAN_POINT('Ctrl Pts',(-9.42743337163542,-103.828019107145,
1.69768315121407E-11));
#35202=CARTESIAN_POINT('Ctrl Pts',(-7.07057502871922,-103.653019107145,
4.08219839617346));
#35203=CARTESIAN_POINT('Ctrl Pts',(-4.71371668580301,-103.478019107145,
8.16439679232994));
#35204=CARTESIAN_POINT('Ctrl Pts',(1.47018674401621E-11,-103.303019107145,
8.16439679232146));
#35205=CARTESIAN_POINT('Ctrl Pts',(4.71371668583241,-103.128019107145,8.16439679231297));
#35206=CARTESIAN_POINT('Ctrl Pts',(7.07057502873392,-102.953019107145,4.082198396148));
#35207=CARTESIAN_POINT('Ctrl Pts',(9.42743337163542,-102.778019107145,-1.69756769845304E-11));
#35208=CARTESIAN_POINT('Ctrl Pts',(7.07057502871922,-102.603019107145,-4.08219839617346));
#35209=CARTESIAN_POINT('Ctrl Pts',(4.71371668580301,-102.428019107145,-8.16439679232994));
#35210=CARTESIAN_POINT('Ctrl Pts',(-1.4702867290402E-11,-102.253019107145,
-8.16439679232146));
#35211=CARTESIAN_POINT('Ctrl Pts',(-4.71371668583241,-102.078019107145,
-8.16439679231297));
#35212=CARTESIAN_POINT('Ctrl Pts',(-7.07057502873392,-101.903019107145,
-4.082198396148));
#35213=CARTESIAN_POINT('Ctrl Pts',(-9.42743337163542,-101.728019107145,
1.69768315121407E-11));
#35214=CARTESIAN_POINT('Ctrl Pts',(-7.07057502871922,-101.553019107145,
4.08219839617346));
#35215=CARTESIAN_POINT('Ctrl Pts',(-4.71371668580301,-101.378019107145,
8.16439679232994));
#35216=CARTESIAN_POINT('Ctrl Pts',(1.47018674401621E-11,-101.203019107145,
8.16439679232146));
#35217=CARTESIAN_POINT('Ctrl Pts',(4.71371668583241,-101.028019107145,8.16439679231297));
#35218=CARTESIAN_POINT('Ctrl Pts',(7.07057502873392,-100.853019107145,4.082198396148));
#35219=CARTESIAN_POINT('Ctrl Pts',(9.42743337163542,-100.678019107145,-1.69756769845304E-11));
#35220=CARTESIAN_POINT('Ctrl Pts',(7.07057502871922,-100.503019107145,-4.08219839617346));
#35221=CARTESIAN_POINT('Ctrl Pts',(4.71371668580301,-100.328019107145,-8.16439679232994));
#35222=CARTESIAN_POINT('Ctrl Pts',(-1.4702867290402E-11,-100.153019107145,
-8.16439679232146));
#35223=CARTESIAN_POINT('Ctrl Pts',(-4.71371668583241,-99.9780191071451,
-8.16439679231297));
#35224=CARTESIAN_POINT('Ctrl Pts',(-7.07057502873392,-99.8030191071451,
-4.082198396148));
#35225=CARTESIAN_POINT('Ctrl Pts',(-9.42743337163542,-99.6280191071451,
1.69768315121407E-11));
#35226=CARTESIAN_POINT('Ctrl Pts',(-7.07057502871922,-99.4530191071451,
4.08219839617346));
#35227=CARTESIAN_POINT('Ctrl Pts',(-4.71371668580301,-99.2780191071451,
8.16439679232994));
#35228=CARTESIAN_POINT('Ctrl Pts',(1.47018674401621E-11,-99.1030191071451,
8.16439679232146));
#35229=CARTESIAN_POINT('Ctrl Pts',(4.71371668583241,-98.9280191071451,8.16439679231297));
#35230=CARTESIAN_POINT('Ctrl Pts',(7.07057502873392,-98.7530191071451,4.082198396148));
#35231=CARTESIAN_POINT('Ctrl Pts',(9.42743337163542,-98.5780191071451,-1.69756769845304E-11));
#35232=CARTESIAN_POINT('Ctrl Pts',(7.07057502871922,-98.4030191071451,-4.08219839617346));
#35233=CARTESIAN_POINT('Ctrl Pts',(4.71371668580301,-98.2280191071451,-8.16439679232994));
#35234=CARTESIAN_POINT('Ctrl Pts',(-1.4702867290402E-11,-98.0530191071451,
-8.16439679232146));
#35235=CARTESIAN_POINT('Ctrl Pts',(-4.71371668583241,-97.8780191071451,
-8.16439679231297));
#35236=CARTESIAN_POINT('Ctrl Pts',(-7.07057502873392,-97.7030191071451,
-4.082198396148));
#35237=CARTESIAN_POINT('Ctrl Pts',(-9.42743337163542,-97.5280191071451,
1.69768315121407E-11));
#35238=CARTESIAN_POINT('Ctrl Pts',(-7.07057502871922,-97.3530191071451,
4.08219839617346));
#35239=CARTESIAN_POINT('Ctrl Pts',(-4.71371668580301,-97.1780191071451,
8.16439679232994));
#35240=CARTESIAN_POINT('Ctrl Pts',(1.47018674401621E-11,-97.0030191071451,
8.16439679232146));
#35241=CARTESIAN_POINT('Ctrl Pts',(4.71371668583241,-96.8280191071451,8.16439679231297));
#35242=CARTESIAN_POINT('Ctrl Pts',(7.07057502873392,-96.6530191071451,4.082198396148));
#35243=CARTESIAN_POINT('Ctrl Pts',(9.42743337163542,-96.4780191071451,-1.69756769845304E-11));
#35244=CARTESIAN_POINT('Ctrl Pts',(7.07057502871922,-96.3030191071451,-4.08219839617346));
#35245=CARTESIAN_POINT('Ctrl Pts',(4.71371668580301,-96.1280191071451,-8.16439679232994));
#35246=CARTESIAN_POINT('Ctrl Pts',(-1.4702867290402E-11,-95.9530191071451,
-8.16439679232146));
#35247=CARTESIAN_POINT('Ctrl Pts',(-4.71371668583241,-95.7780191071451,
-8.16439679231297));
#35248=CARTESIAN_POINT('Ctrl Pts',(-7.07057502873392,-95.6030191071451,
-4.082198396148));
#35249=CARTESIAN_POINT('Ctrl Pts',(-9.42743337163542,-95.4280191071451,
1.69768315121407E-11));
#35250=CARTESIAN_POINT('Ctrl Pts',(-7.07057502871922,-95.2530191071451,
4.08219839617346));
#35251=CARTESIAN_POINT('Ctrl Pts',(-4.71371668580301,-95.0780191071451,
8.16439679232994));
#35252=CARTESIAN_POINT('Ctrl Pts',(1.47018674401621E-11,-94.9030191071451,
8.16439679232146));
#35253=CARTESIAN_POINT('Ctrl Pts',(4.71371668583241,-94.7280191071451,8.16439679231297));
#35254=CARTESIAN_POINT('Ctrl Pts',(7.07057502873392,-94.5530191071451,4.082198396148));
#35255=CARTESIAN_POINT('Ctrl Pts',(9.42743337163542,-94.3780191071451,-1.69756769845304E-11));
#35256=CARTESIAN_POINT('Ctrl Pts',(7.07057502871922,-94.2030191071451,-4.08219839617346));
#35257=CARTESIAN_POINT('Ctrl Pts',(4.71371668580301,-94.0280191071451,-8.16439679232994));
#35258=CARTESIAN_POINT('Ctrl Pts',(-1.4702867290402E-11,-93.8530191071451,
-8.16439679232146));
#35259=CARTESIAN_POINT('Ctrl Pts',(-4.71371668583241,-93.6780191071451,
-8.16439679231297));
#35260=CARTESIAN_POINT('Ctrl Pts',(-7.07057502873392,-93.5030191071451,
-4.082198396148));
#35261=CARTESIAN_POINT('Ctrl Pts',(-9.42743337163542,-93.3280191071451,
1.69768315121407E-11));
#35262=CARTESIAN_POINT('Ctrl Pts',(-7.07057502871922,-93.1530191071451,
4.08219839617346));
#35263=CARTESIAN_POINT('Ctrl Pts',(-4.71371668580301,-92.9780191071451,
8.16439679232994));
#35264=CARTESIAN_POINT('Ctrl Pts',(1.47018674401621E-11,-92.8030191071451,
8.16439679232146));
#35265=CARTESIAN_POINT('Ctrl Pts',(4.71371668583241,-92.6280191071451,8.16439679231297));
#35266=CARTESIAN_POINT('Ctrl Pts',(7.07057502873392,-92.4530191071451,4.082198396148));
#35267=CARTESIAN_POINT('Ctrl Pts',(9.42743337163542,-92.2780191071451,-1.69756769845304E-11));
#35268=CARTESIAN_POINT('Ctrl Pts',(7.07057502871922,-92.1030191071451,-4.08219839617346));
#35269=CARTESIAN_POINT('Ctrl Pts',(4.71371668580301,-91.9280191071451,-8.16439679232994));
#35270=CARTESIAN_POINT('Ctrl Pts',(-1.4702867290402E-11,-91.7530191071451,
-8.16439679232146));
#35271=CARTESIAN_POINT('Ctrl Pts',(-4.71371668583241,-91.5780191071451,
-8.16439679231297));
#35272=CARTESIAN_POINT('Ctrl Pts',(-7.07057502873392,-91.4030191071451,
-4.082198396148));
#35273=CARTESIAN_POINT('Ctrl Pts',(-9.42743337163542,-91.2280191071451,
1.69768315121407E-11));
#35274=CARTESIAN_POINT('Ctrl Pts',(-7.07057502871922,-91.0530191071451,
4.08219839617346));
#35275=CARTESIAN_POINT('Ctrl Pts',(-4.71371668580301,-90.8780191071451,
8.16439679232994));
#35276=CARTESIAN_POINT('Ctrl Pts',(1.47018674401621E-11,-90.7030191071451,
8.16439679232146));
#35277=CARTESIAN_POINT('Ctrl Pts',(4.71371668583241,-90.5280191071451,8.16439679231297));
#35278=CARTESIAN_POINT('Ctrl Pts',(7.07057502873392,-90.3530191071451,4.082198396148));
#35279=CARTESIAN_POINT('Ctrl Pts',(9.42743337163542,-90.1780191071451,-1.69756769845304E-11));
#35280=CARTESIAN_POINT('Ctrl Pts',(7.07057502871922,-90.0030191071451,-4.08219839617346));
#35281=CARTESIAN_POINT('Ctrl Pts',(4.71371668580301,-89.8280191071451,-8.16439679232994));
#35282=CARTESIAN_POINT('Ctrl Pts',(-1.4702867290402E-11,-89.6530191071451,
-8.16439679232146));
#35283=CARTESIAN_POINT('Ctrl Pts',(-4.71371668583241,-89.4780191071451,
-8.16439679231297));
#35284=CARTESIAN_POINT('Ctrl Pts',(-7.07057502873392,-89.3030191071451,
-4.082198396148));
#35285=CARTESIAN_POINT('Ctrl Pts',(-9.42743337163542,-89.1280191071451,
1.69768315121407E-11));
#35286=CARTESIAN_POINT('Ctrl Pts',(-7.07057502871922,-88.9530191071451,
4.08219839617346));
#35287=CARTESIAN_POINT('Ctrl Pts',(-4.71371668580301,-88.7780191071451,
8.16439679232994));
#35288=CARTESIAN_POINT('Ctrl Pts',(1.47018674401621E-11,-88.6030191071451,
8.16439679232146));
#35289=CARTESIAN_POINT('Ctrl Pts',(4.71371668583241,-88.4280191071451,8.16439679231297));
#35290=CARTESIAN_POINT('Ctrl Pts',(7.07057502873392,-88.2530191071451,4.082198396148));
#35291=CARTESIAN_POINT('Ctrl Pts',(9.42743337163542,-88.0780191071452,-1.69756769845304E-11));
#35292=CARTESIAN_POINT('Ctrl Pts',(7.07057502871922,-87.9030191071451,-4.08219839617346));
#35293=CARTESIAN_POINT('Ctrl Pts',(4.71371668580301,-87.7280191071451,-8.16439679232994));
#35294=CARTESIAN_POINT('Ctrl Pts',(-1.4702867290402E-11,-87.5530191071451,
-8.16439679232146));
#35295=CARTESIAN_POINT('Ctrl Pts',(-4.71371668583241,-87.3780191071451,
-8.16439679231297));
#35296=CARTESIAN_POINT('Ctrl Pts',(-7.07057502873392,-87.2030191071451,
-4.082198396148));
#35297=CARTESIAN_POINT('Ctrl Pts',(-9.42743337163542,-87.0280191071451,
1.69768315121407E-11));
#35298=CARTESIAN_POINT('Ctrl Pts',(-7.07057502871922,-86.8530191071451,
4.08219839617346));
#35299=CARTESIAN_POINT('Ctrl Pts',(-4.71371668580301,-86.6780191071451,
8.16439679232994));
#35300=CARTESIAN_POINT('Ctrl Pts',(1.47018674401621E-11,-86.5030191071452,
8.16439679232146));
#35301=CARTESIAN_POINT('Ctrl Pts',(4.71371668583241,-86.3280191071451,8.16439679231297));
#35302=CARTESIAN_POINT('Ctrl Pts',(7.07057502873392,-86.1530191071451,4.082198396148));
#35303=CARTESIAN_POINT('Ctrl Pts',(9.42743337163542,-85.9780191071451,-1.69756769845304E-11));
#35304=CARTESIAN_POINT('Ctrl Pts',(7.07057502871922,-85.8030191071452,-4.08219839617346));
#35305=CARTESIAN_POINT('Ctrl Pts',(4.71371668580301,-85.6280191071451,-8.16439679232994));
#35306=CARTESIAN_POINT('Ctrl Pts',(-1.4702867290402E-11,-85.4530191071451,
-8.16439679232146));
#35307=CARTESIAN_POINT('Ctrl Pts',(-4.71371668583241,-85.2780191071451,
-8.16439679231297));
#35308=CARTESIAN_POINT('Ctrl Pts',(-7.07057502873392,-85.1030191071451,
-4.082198396148));
#35309=CARTESIAN_POINT('Ctrl Pts',(-9.42743337163542,-84.9280191071451,
1.69768315121407E-11));
#35310=CARTESIAN_POINT('Ctrl Pts',(-7.07057502871922,-84.7530191071451,
4.08219839617346));
#35311=CARTESIAN_POINT('Ctrl Pts',(-4.71371668580301,-84.5780191071451,
8.16439679232994));
#35312=CARTESIAN_POINT('Ctrl Pts',(1.47018674401621E-11,-84.4030191071451,
8.16439679232146));
#35313=CARTESIAN_POINT('Ctrl Pts',(4.71371668583241,-84.2280191071451,8.16439679231297));
#35314=CARTESIAN_POINT('Ctrl Pts',(7.07057502873392,-84.0530191071451,4.082198396148));
#35315=CARTESIAN_POINT('Ctrl Pts',(9.42743337163542,-83.8780191071451,-1.69756769845304E-11));
#35316=CARTESIAN_POINT('Ctrl Pts',(7.07057502871922,-83.7030191071452,-4.08219839617346));
#35317=CARTESIAN_POINT('Ctrl Pts',(4.71371668580301,-83.5280191071451,-8.16439679232994));
#35318=CARTESIAN_POINT('Ctrl Pts',(-1.4702867290402E-11,-83.3530191071451,
-8.16439679232146));
#35319=CARTESIAN_POINT('Ctrl Pts',(-4.71371668583241,-83.1780191071451,
-8.16439679231297));
#35320=CARTESIAN_POINT('Ctrl Pts',(-7.07057502873392,-83.0030191071451,
-4.082198396148));
#35321=CARTESIAN_POINT('Ctrl Pts',(-9.42743337163542,-82.8280191071451,
1.69768315121407E-11));
#35322=CARTESIAN_POINT('Ctrl Pts',(-7.07057502871922,-82.6530191071451,
4.08219839617346));
#35323=CARTESIAN_POINT('Ctrl Pts',(-4.71371668580301,-82.4780191071451,
8.16439679232994));
#35324=CARTESIAN_POINT('Ctrl Pts',(1.47018674401621E-11,-82.3030191071451,
8.16439679232146));
#35325=CARTESIAN_POINT('Ctrl Pts',(4.71371668583241,-82.1280191071452,8.16439679231297));
#35326=CARTESIAN_POINT('Ctrl Pts',(7.07057502873392,-81.9530191071452,4.082198396148));
#35327=CARTESIAN_POINT('Ctrl Pts',(9.42743337163542,-81.7780191071451,-1.69756769845304E-11));
#35328=CARTESIAN_POINT('Ctrl Pts',(7.07057502871922,-81.6030191071452,-4.08219839617346));
#35329=CARTESIAN_POINT('Ctrl Pts',(4.71371668580301,-81.4280191071452,-8.16439679232994));
#35330=CARTESIAN_POINT('Ctrl Pts',(-1.4702867290402E-11,-81.2530191071451,
-8.16439679232146));
#35331=CARTESIAN_POINT('Ctrl Pts',(-4.71371668583241,-81.0780191071451,
-8.16439679231297));
#35332=CARTESIAN_POINT('Ctrl Pts',(-7.07057502873392,-80.9030191071452,
-4.082198396148));
#35333=CARTESIAN_POINT('Ctrl Pts',(-9.42743337163542,-80.7280191071451,
1.69768315121407E-11));
#35334=CARTESIAN_POINT('Ctrl Pts',(-7.07057502871922,-80.5530191071452,
4.08219839617346));
#35335=CARTESIAN_POINT('Ctrl Pts',(-4.71371668580301,-80.3780191071451,
8.16439679232994));
#35336=CARTESIAN_POINT('Ctrl Pts',(1.47018674401621E-11,-80.2030191071451,
8.16439679232146));
#35337=CARTESIAN_POINT('Ctrl Pts',(4.71371668583241,-80.0280191071451,8.16439679231297));
#35338=CARTESIAN_POINT('Ctrl Pts',(7.07057502873392,-79.8530191071451,4.082198396148));
#35339=CARTESIAN_POINT('Ctrl Pts',(9.42743337163542,-79.6780191071451,-1.69756769845304E-11));
#35340=CARTESIAN_POINT('Ctrl Pts',(7.07057502871922,-79.5030191071451,-4.08219839617346));
#35341=CARTESIAN_POINT('Ctrl Pts',(4.71371668580301,-79.3280191071452,-8.16439679232994));
#35342=CARTESIAN_POINT('Ctrl Pts',(-1.4702867290402E-11,-79.1530191071452,
-8.16439679232146));
#35343=CARTESIAN_POINT('Ctrl Pts',(-4.71371668583241,-78.9780191071451,
-8.16439679231297));
#35344=CARTESIAN_POINT('Ctrl Pts',(-7.07057502873392,-78.8030191071452,
-4.082198396148));
#35345=CARTESIAN_POINT('Ctrl Pts',(-9.42743337163542,-78.6280191071451,
1.69768315121407E-11));
#35346=CARTESIAN_POINT('Ctrl Pts',(-7.07057502871922,-78.4530191071451,
4.08219839617346));
#35347=CARTESIAN_POINT('Ctrl Pts',(-4.71371668580301,-78.2780191071452,
8.16439679232994));
#35348=CARTESIAN_POINT('Ctrl Pts',(1.47018674401621E-11,-78.1030191071452,
8.16439679232146));
#35349=CARTESIAN_POINT('Ctrl Pts',(4.71371668583241,-77.9280191071451,8.16439679231297));
#35350=CARTESIAN_POINT('Ctrl Pts',(7.07057502873392,-77.7530191071452,4.082198396148));
#35351=CARTESIAN_POINT('Ctrl Pts',(9.42743337163542,-77.5780191071452,-1.69756769845304E-11));
#35352=CARTESIAN_POINT('Ctrl Pts',(7.07057502871922,-77.4030191071451,-4.08219839617346));
#35353=CARTESIAN_POINT('Ctrl Pts',(4.71371668580301,-77.2280191071452,-8.16439679232994));
#35354=CARTESIAN_POINT('Ctrl Pts',(-1.4702867290402E-11,-77.0530191071452,
-8.16439679232146));
#35355=CARTESIAN_POINT('Ctrl Pts',(-4.71371668583241,-76.8780191071451,
-8.16439679231297));
#35356=CARTESIAN_POINT('Ctrl Pts',(-7.07057502873392,-76.7030191071452,
-4.082198396148));
#35357=CARTESIAN_POINT('Ctrl Pts',(-9.42743337163542,-76.5280191071452,
1.69768315121407E-11));
#35358=CARTESIAN_POINT('Ctrl Pts',(-7.07057502871922,-76.3530191071451,
4.08219839617346));
#35359=CARTESIAN_POINT('Ctrl Pts',(-4.71371668580301,-76.1780191071451,
8.16439679232994));
#35360=CARTESIAN_POINT('Ctrl Pts',(1.47018674401621E-11,-76.0030191071452,
8.16439679232146));
#35361=CARTESIAN_POINT('Ctrl Pts',(4.71371668583241,-75.8280191071452,8.16439679231297));
#35362=CARTESIAN_POINT('Ctrl Pts',(7.07057502873392,-75.6530191071451,4.082198396148));
#35363=CARTESIAN_POINT('Ctrl Pts',(9.42743337163542,-75.4780191071452,-1.69756769845304E-11));
#35364=CARTESIAN_POINT('Ctrl Pts',(7.07057502871922,-75.3030191071451,-4.08219839617346));
#35365=CARTESIAN_POINT('Ctrl Pts',(4.71371668580301,-75.1280191071451,-8.16439679232994));
#35366=CARTESIAN_POINT('Ctrl Pts',(-1.4702867290402E-11,-74.9530191071452,
-8.16439679232146));
#35367=CARTESIAN_POINT('Ctrl Pts',(-4.71371668583241,-74.7780191071452,
-8.16439679231297));
#35368=CARTESIAN_POINT('Ctrl Pts',(-7.07057502873392,-74.6030191071451,
-4.082198396148));
#35369=CARTESIAN_POINT('Ctrl Pts',(-9.42743337163542,-74.4280191071451,
1.69768315121407E-11));
#35370=CARTESIAN_POINT('Ctrl Pts',(-7.07057502871922,-74.2530191071452,
4.08219839617346));
#35371=CARTESIAN_POINT('Ctrl Pts',(-4.71371668580301,-74.0780191071452,
8.16439679232994));
#35372=CARTESIAN_POINT('Ctrl Pts',(1.47018674401621E-11,-73.9030191071452,
8.16439679232146));
#35373=CARTESIAN_POINT('Ctrl Pts',(4.71371668583241,-73.7280191071452,8.16439679231297));
#35374=CARTESIAN_POINT('Ctrl Pts',(7.07057502873392,-73.5530191071451,4.082198396148));
#35375=CARTESIAN_POINT('Ctrl Pts',(9.42743337163542,-73.3780191071452,-1.69756769845304E-11));
#35376=CARTESIAN_POINT('Ctrl Pts',(7.07057502871922,-73.2030191071452,-4.08219839617346));
#35377=CARTESIAN_POINT('Ctrl Pts',(4.71371668580301,-73.0280191071452,-8.16439679232994));
#35378=CARTESIAN_POINT('Ctrl Pts',(-1.4702867290402E-11,-72.8530191071452,
-8.16439679232146));
#35379=CARTESIAN_POINT('Ctrl Pts',(-4.71371668583241,-72.6780191071452,
-8.16439679231297));
#35380=CARTESIAN_POINT('Ctrl Pts',(-7.07057502873392,-72.5030191071451,
-4.082198396148));
#35381=CARTESIAN_POINT('Ctrl Pts',(-9.42743337163542,-72.3280191071452,
1.69768315121407E-11));
#35382=CARTESIAN_POINT('Ctrl Pts',(-7.07057502871922,-72.1530191071452,
4.08219839617346));
#35383=CARTESIAN_POINT('Ctrl Pts',(-4.71371668580301,-71.9780191071451,
8.16439679232994));
#35384=CARTESIAN_POINT('Ctrl Pts',(1.47018674401621E-11,-71.8030191071452,
8.16439679232146));
#35385=CARTESIAN_POINT('Ctrl Pts',(4.71371668583241,-71.6280191071452,8.16439679231297));
#35386=CARTESIAN_POINT('Ctrl Pts',(7.07057502873392,-71.4530191071452,4.082198396148));
#35387=CARTESIAN_POINT('Ctrl Pts',(9.42743337163542,-71.2780191071452,-1.69756769845304E-11));
#35388=CARTESIAN_POINT('Ctrl Pts',(7.07057502871922,-71.1030191071452,-4.08219839617346));
#35389=CARTESIAN_POINT('Ctrl Pts',(4.71371668580301,-70.9280191071451,-8.16439679232994));
#35390=CARTESIAN_POINT('Ctrl Pts',(-1.4702867290402E-11,-70.7530191071451,
-8.16439679232146));
#35391=CARTESIAN_POINT('Ctrl Pts',(-4.71371668583241,-70.5780191071452,
-8.16439679231297));
#35392=CARTESIAN_POINT('Ctrl Pts',(-7.07057502873392,-70.4030191071452,
-4.082198396148));
#35393=CARTESIAN_POINT('Ctrl Pts',(-9.42743337163542,-70.2280191071452,
1.69768315121407E-11));
#35394=CARTESIAN_POINT('Ctrl Pts',(-7.07057502871922,-70.0530191071452,
4.08219839617346));
#35395=CARTESIAN_POINT('Ctrl Pts',(-4.71371668580301,-69.8780191071452,
8.16439679232994));
#35396=CARTESIAN_POINT('Ctrl Pts',(1.47018674401621E-11,-69.7030191071452,
8.16439679232146));
#35397=CARTESIAN_POINT('Ctrl Pts',(4.71371668583241,-69.5280191071452,8.16439679231297));
#35398=CARTESIAN_POINT('Ctrl Pts',(7.07057502873392,-69.3530191071452,4.082198396148));
#35399=CARTESIAN_POINT('Ctrl Pts',(9.42743337163542,-69.1780191071452,-1.69756769845304E-11));
#35400=CARTESIAN_POINT('Ctrl Pts',(7.07057502871922,-69.0030191071452,-4.08219839617346));
#35401=CARTESIAN_POINT('Ctrl Pts',(4.71371668580301,-68.8280191071452,-8.16439679232994));
#35402=CARTESIAN_POINT('Ctrl Pts',(-1.4702867290402E-11,-68.6530191071452,
-8.16439679232146));
#35403=CARTESIAN_POINT('Ctrl Pts',(-4.71371668583241,-68.4780191071452,
-8.16439679231297));
#35404=CARTESIAN_POINT('Ctrl Pts',(-7.07057502873392,-68.3030191071452,
-4.082198396148));
#35405=CARTESIAN_POINT('Ctrl Pts',(-9.42743337163542,-68.1280191071452,
1.69768315121407E-11));
#35406=CARTESIAN_POINT('Ctrl Pts',(-7.07057502871922,-67.9530191071452,
4.08219839617346));
#35407=CARTESIAN_POINT('Ctrl Pts',(-4.71371668580301,-67.7780191071452,
8.16439679232994));
#35408=CARTESIAN_POINT('Ctrl Pts',(1.47018674401621E-11,-67.6030191071452,
8.16439679232146));
#35409=CARTESIAN_POINT('Ctrl Pts',(4.71371668583241,-67.4280191071452,8.16439679231297));
#35410=CARTESIAN_POINT('Ctrl Pts',(7.07057502873392,-67.2530191071452,4.082198396148));
#35411=CARTESIAN_POINT('Ctrl Pts',(9.42743337163542,-67.0780191071452,-1.69756769845304E-11));
#35412=CARTESIAN_POINT('Ctrl Pts',(7.07057502871922,-66.9030191071452,-4.08219839617346));
#35413=CARTESIAN_POINT('Ctrl Pts',(4.71371668580301,-66.7280191071452,-8.16439679232994));
#35414=CARTESIAN_POINT('Ctrl Pts',(-1.4702867290402E-11,-66.5530191071452,
-8.16439679232146));
#35415=CARTESIAN_POINT('Ctrl Pts',(-4.71371668583241,-66.3780191071452,
-8.16439679231297));
#35416=CARTESIAN_POINT('Ctrl Pts',(-7.07057502873392,-66.2030191071452,
-4.082198396148));
#35417=CARTESIAN_POINT('Ctrl Pts',(-9.42743337163542,-66.0280191071452,
1.69768315121407E-11));
#35418=CARTESIAN_POINT('Ctrl Pts',(-7.07057502871922,-65.8530191071452,
4.08219839617346));
#35419=CARTESIAN_POINT('Ctrl Pts',(-4.71371668580301,-65.6780191071452,
8.16439679232994));
#35420=CARTESIAN_POINT('Ctrl Pts',(1.47018674401621E-11,-65.5030191071452,
8.16439679232146));
#35421=CARTESIAN_POINT('Ctrl Pts',(4.71371668583241,-65.3280191071452,8.16439679231297));
#35422=CARTESIAN_POINT('Ctrl Pts',(7.07057502873392,-65.1530191071452,4.082198396148));
#35423=CARTESIAN_POINT('Ctrl Pts',(9.42743337163542,-64.9780191071452,-1.69756769845304E-11));
#35424=CARTESIAN_POINT('Ctrl Pts',(7.07057502871922,-64.8030191071452,-4.08219839617346));
#35425=CARTESIAN_POINT('Ctrl Pts',(4.71371668580301,-64.6280191071452,-8.16439679232994));
#35426=CARTESIAN_POINT('Ctrl Pts',(-1.4702867290402E-11,-64.4530191071452,
-8.16439679232146));
#35427=CARTESIAN_POINT('Ctrl Pts',(-4.71371668583241,-64.2780191071452,
-8.16439679231297));
#35428=CARTESIAN_POINT('Ctrl Pts',(-7.07057502873392,-64.1030191071452,
-4.082198396148));
#35429=CARTESIAN_POINT('Ctrl Pts',(-9.42743337163542,-63.9280191071452,
1.69768315121407E-11));
#35430=CARTESIAN_POINT('Ctrl Pts',(-7.07057502871922,-63.7530191071452,
4.08219839617346));
#35431=CARTESIAN_POINT('Ctrl Pts',(-4.71371668580301,-63.5780191071452,
8.16439679232994));
#35432=CARTESIAN_POINT('Ctrl Pts',(1.47018674401621E-11,-63.4030191071452,
8.16439679232146));
#35433=CARTESIAN_POINT('Ctrl Pts',(4.71371668583241,-63.2280191071452,8.16439679231297));
#35434=CARTESIAN_POINT('Ctrl Pts',(7.07057502873392,-63.0530191071452,4.082198396148));
#35435=CARTESIAN_POINT('Ctrl Pts',(9.42743337163542,-62.8780191071452,-1.69756769845304E-11));
#35436=CARTESIAN_POINT('Ctrl Pts',(7.07057502871922,-62.7030191071452,-4.08219839617346));
#35437=CARTESIAN_POINT('Ctrl Pts',(4.71371668580301,-62.5280191071452,-8.16439679232994));
#35438=CARTESIAN_POINT('Ctrl Pts',(-1.4702867290402E-11,-62.3530191071452,
-8.16439679232146));
#35439=CARTESIAN_POINT('Ctrl Pts',(-4.71371668583241,-62.1780191071452,
-8.16439679231297));
#35440=CARTESIAN_POINT('Ctrl Pts',(-7.07057502873392,-62.0030191071452,
-4.082198396148));
#35441=CARTESIAN_POINT('Ctrl Pts',(-9.42743337163542,-61.8280191071452,
1.69768315121407E-11));
#35442=CARTESIAN_POINT('Ctrl Pts',(-7.07057502871922,-61.6530191071452,
4.08219839617346));
#35443=CARTESIAN_POINT('Ctrl Pts',(-4.71371668580301,-61.4780191071452,
8.16439679232994));
#35444=CARTESIAN_POINT('Ctrl Pts',(1.47018674401621E-11,-61.3030191071452,
8.16439679232146));
#35445=CARTESIAN_POINT('Ctrl Pts',(4.71371668583241,-61.1280191071452,8.16439679231297));
#35446=CARTESIAN_POINT('Ctrl Pts',(7.07057502873392,-60.9530191071452,4.082198396148));
#35447=CARTESIAN_POINT('Ctrl Pts',(9.42743337163542,-60.7780191071452,-1.69756769845304E-11));
#35448=CARTESIAN_POINT('Ctrl Pts',(7.07057502871922,-60.6030191071452,-4.08219839617346));
#35449=CARTESIAN_POINT('Ctrl Pts',(4.71371668580301,-60.4280191071452,-8.16439679232994));
#35450=CARTESIAN_POINT('Ctrl Pts',(-1.4702867290402E-11,-60.2530191071452,
-8.16439679232146));
#35451=CARTESIAN_POINT('Ctrl Pts',(-4.71371668583241,-60.0780191071452,
-8.16439679231297));
#35452=CARTESIAN_POINT('Ctrl Pts',(-7.07057502873392,-59.9030191071452,
-4.082198396148));
#35453=CARTESIAN_POINT('Ctrl Pts',(-9.42743337163542,-59.7280191071452,
1.69768315121407E-11));
#35454=CARTESIAN_POINT('Ctrl Pts',(-7.07057502871922,-59.5530191071452,
4.08219839617346));
#35455=CARTESIAN_POINT('Ctrl Pts',(-4.71371668580301,-59.3780191071452,
8.16439679232994));
#35456=CARTESIAN_POINT('Ctrl Pts',(1.47018674401621E-11,-59.2030191071452,
8.16439679232146));
#35457=CARTESIAN_POINT('Ctrl Pts',(4.71371668583241,-59.0280191071452,8.16439679231297));
#35458=CARTESIAN_POINT('Ctrl Pts',(7.07057502873392,-58.8530191071452,4.082198396148));
#35459=CARTESIAN_POINT('Ctrl Pts',(9.42743337163542,-58.6780191071452,-1.69756769845304E-11));
#35460=CARTESIAN_POINT('Ctrl Pts',(7.07057502871922,-58.5030191071452,-4.08219839617346));
#35461=CARTESIAN_POINT('Ctrl Pts',(4.71371668580301,-58.3280191071452,-8.16439679232994));
#35462=CARTESIAN_POINT('Ctrl Pts',(-1.4702867290402E-11,-58.1530191071452,
-8.16439679232146));
#35463=CARTESIAN_POINT('Ctrl Pts',(-4.71371668583241,-57.9780191071452,
-8.16439679231297));
#35464=CARTESIAN_POINT('Ctrl Pts',(-7.07057502873392,-57.8030191071452,
-4.082198396148));
#35465=CARTESIAN_POINT('Ctrl Pts',(-9.42743337163542,-57.6280191071452,
1.69768315121407E-11));
#35466=CARTESIAN_POINT('Ctrl Pts',(-7.07057502871922,-57.4530191071452,
4.08219839617346));
#35467=CARTESIAN_POINT('Ctrl Pts',(-4.71371668580301,-57.2780191071452,
8.16439679232994));
#35468=CARTESIAN_POINT('Ctrl Pts',(1.47018674401621E-11,-57.1030191071452,
8.16439679232146));
#35469=CARTESIAN_POINT('Ctrl Pts',(4.71371668583241,-56.9280191071452,8.16439679231297));
#35470=CARTESIAN_POINT('Ctrl Pts',(7.07057502873392,-56.7530191071452,4.082198396148));
#35471=CARTESIAN_POINT('Ctrl Pts',(9.42743337163542,-56.5780191071452,-1.69756769845304E-11));
#35472=CARTESIAN_POINT('Ctrl Pts',(7.07057502871922,-56.4030191071452,-4.08219839617346));
#35473=CARTESIAN_POINT('Ctrl Pts',(4.71371668580301,-56.2280191071452,-8.16439679232994));
#35474=CARTESIAN_POINT('Ctrl Pts',(-1.4702867290402E-11,-56.0530191071452,
-8.16439679232146));
#35475=CARTESIAN_POINT('Ctrl Pts',(-4.71371668583241,-55.8780191071452,
-8.16439679231297));
#35476=CARTESIAN_POINT('Ctrl Pts',(-7.07057502873392,-55.7030191071452,
-4.082198396148));
#35477=CARTESIAN_POINT('Ctrl Pts',(-9.42743337163542,-55.5280191071452,
1.69768315121407E-11));
#35478=CARTESIAN_POINT('Ctrl Pts',(-7.07057502871922,-55.3530191071452,
4.08219839617346));
#35479=CARTESIAN_POINT('Ctrl Pts',(-4.71371668580301,-55.1780191071452,
8.16439679232994));
#35480=CARTESIAN_POINT('Ctrl Pts',(1.47018674401621E-11,-55.0030191071452,
8.16439679232146));
#35481=CARTESIAN_POINT('Ctrl Pts',(4.71371668583241,-54.8280191071452,8.16439679231297));
#35482=CARTESIAN_POINT('Ctrl Pts',(7.07057502873392,-54.6530191071452,4.082198396148));
#35483=CARTESIAN_POINT('Ctrl Pts',(9.42743337163542,-54.4780191071452,-1.69756769845304E-11));
#35484=CARTESIAN_POINT('Ctrl Pts',(7.07057502871922,-54.3030191071452,-4.08219839617346));
#35485=CARTESIAN_POINT('Ctrl Pts',(4.71371668580301,-54.1280191071452,-8.16439679232994));
#35486=CARTESIAN_POINT('Ctrl Pts',(-1.4702867290402E-11,-53.9530191071452,
-8.16439679232146));
#35487=CARTESIAN_POINT('Ctrl Pts',(-4.71371668583241,-53.7780191071452,
-8.16439679231297));
#35488=CARTESIAN_POINT('Ctrl Pts',(-7.07057502873392,-53.6030191071452,
-4.082198396148));
#35489=CARTESIAN_POINT('Ctrl Pts',(-9.42743337163542,-53.4280191071452,
1.69768315121407E-11));
#35490=CARTESIAN_POINT('Ctrl Pts',(-7.07057502871922,-53.2530191071452,
4.08219839617346));
#35491=CARTESIAN_POINT('Ctrl Pts',(-4.71371668580301,-53.0780191071452,
8.16439679232994));
#35492=CARTESIAN_POINT('Ctrl Pts',(1.47018674401621E-11,-52.9030191071452,
8.16439679232146));
#35493=CARTESIAN_POINT('Ctrl Pts',(4.71371668583241,-52.7280191071452,8.16439679231297));
#35494=CARTESIAN_POINT('Ctrl Pts',(7.07057502873392,-52.5530191071452,4.082198396148));
#35495=CARTESIAN_POINT('Ctrl Pts',(9.42743337163542,-52.3780191071452,-1.69756769845304E-11));
#35496=CARTESIAN_POINT('Ctrl Pts',(7.07057502871922,-52.2030191071452,-4.08219839617346));
#35497=CARTESIAN_POINT('Ctrl Pts',(4.71371668580301,-52.0280191071452,-8.16439679232994));
#35498=CARTESIAN_POINT('Ctrl Pts',(-1.4702867290402E-11,-51.8530191071452,
-8.16439679232146));
#35499=CARTESIAN_POINT('Ctrl Pts',(-4.71371668583241,-51.6780191071452,
-8.16439679231297));
#35500=CARTESIAN_POINT('Ctrl Pts',(-7.07057502873392,-51.5030191071452,
-4.082198396148));
#35501=CARTESIAN_POINT('Ctrl Pts',(-9.42743337163542,-51.3280191071452,
1.69768315121407E-11));
#35502=CARTESIAN_POINT('Ctrl Pts',(-7.07057502871922,-51.1530191071452,
4.08219839617346));
#35503=CARTESIAN_POINT('Ctrl Pts',(-4.71371668580301,-50.9780191071452,
8.16439679232994));
#35504=CARTESIAN_POINT('Ctrl Pts',(1.47018674401621E-11,-50.8030191071452,
8.16439679232146));
#35505=CARTESIAN_POINT('Ctrl Pts',(4.71371668583241,-50.6280191071452,8.16439679231297));
#35506=CARTESIAN_POINT('Ctrl Pts',(7.07057502873392,-50.4530191071452,4.082198396148));
#35507=CARTESIAN_POINT('Ctrl Pts',(9.42743337163542,-50.2780191071452,-1.69756769845304E-11));
#35508=CARTESIAN_POINT('Ctrl Pts',(7.07057502871922,-50.1030191071452,-4.08219839617346));
#35509=CARTESIAN_POINT('Ctrl Pts',(4.71371668580301,-49.9280191071452,-8.16439679232994));
#35510=CARTESIAN_POINT('Ctrl Pts',(-1.4702867290402E-11,-49.7530191071452,
-8.16439679232146));
#35511=CARTESIAN_POINT('Ctrl Pts',(-4.71371668583241,-49.5780191071452,
-8.16439679231297));
#35512=CARTESIAN_POINT('Ctrl Pts',(-7.07057502873392,-49.4030191071452,
-4.082198396148));
#35513=CARTESIAN_POINT('Ctrl Pts',(-9.42743337163542,-49.2280191071452,
1.69768315121407E-11));
#35514=CARTESIAN_POINT('Ctrl Pts',(-7.07057502871922,-49.0530191071452,
4.08219839617346));
#35515=CARTESIAN_POINT('Ctrl Pts',(-4.71371668580301,-48.8780191071452,
8.16439679232994));
#35516=CARTESIAN_POINT('Ctrl Pts',(1.47018674401621E-11,-48.7030191071452,
8.16439679232146));
#35517=CARTESIAN_POINT('Ctrl Pts',(4.71371668583241,-48.5280191071452,8.16439679231297));
#35518=CARTESIAN_POINT('Ctrl Pts',(7.07057502873392,-48.3530191071452,4.082198396148));
#35519=CARTESIAN_POINT('Ctrl Pts',(9.42743337163542,-48.1780191071452,-1.69756769845304E-11));
#35520=CARTESIAN_POINT('Ctrl Pts',(7.07057502871922,-48.0030191071452,-4.08219839617346));
#35521=CARTESIAN_POINT('Ctrl Pts',(4.71371668580301,-47.8280191071452,-8.16439679232994));
#35522=CARTESIAN_POINT('Ctrl Pts',(-1.4702867290402E-11,-47.6530191071452,
-8.16439679232146));
#35523=CARTESIAN_POINT('Ctrl Pts',(-4.71371668583241,-47.4780191071452,
-8.16439679231297));
#35524=CARTESIAN_POINT('Ctrl Pts',(-7.07057502873392,-47.3030191071452,
-4.082198396148));
#35525=CARTESIAN_POINT('Ctrl Pts',(-9.42743337163542,-47.1280191071452,
1.69768315121407E-11));
#35526=CARTESIAN_POINT('Ctrl Pts',(-7.07057502871922,-46.9530191071452,
4.08219839617346));
#35527=CARTESIAN_POINT('Ctrl Pts',(-4.71371668580301,-46.7780191071452,
8.16439679232994));
#35528=CARTESIAN_POINT('Ctrl Pts',(1.47018674401621E-11,-46.6030191071452,
8.16439679232146));
#35529=CARTESIAN_POINT('Ctrl Pts',(4.71371668583241,-46.4280191071452,8.16439679231297));
#35530=CARTESIAN_POINT('Ctrl Pts',(7.07057502873392,-46.2530191071452,4.082198396148));
#35531=CARTESIAN_POINT('Ctrl Pts',(9.42743337163542,-46.0780191071452,-1.69756769845304E-11));
#35532=CARTESIAN_POINT('Ctrl Pts',(7.07057502871922,-45.9030191071452,-4.08219839617346));
#35533=CARTESIAN_POINT('Ctrl Pts',(4.71371668580301,-45.7280191071452,-8.16439679232994));
#35534=CARTESIAN_POINT('Ctrl Pts',(-1.4702867290402E-11,-45.5530191071452,
-8.16439679232146));
#35535=CARTESIAN_POINT('Ctrl Pts',(-4.71371668583241,-45.3780191071452,
-8.16439679231297));
#35536=CARTESIAN_POINT('Ctrl Pts',(-7.07057502873392,-45.2030191071452,
-4.082198396148));
#35537=CARTESIAN_POINT('Ctrl Pts',(-9.42743337163542,-45.0280191071452,
1.69768315121407E-11));
#35538=CARTESIAN_POINT('Ctrl Pts',(-7.07057502871922,-44.8530191071452,
4.08219839617346));
#35539=CARTESIAN_POINT('Ctrl Pts',(-4.71371668580301,-44.6780191071452,
8.16439679232994));
#35540=CARTESIAN_POINT('Ctrl Pts',(1.47018674401621E-11,-44.5030191071452,
8.16439679232146));
#35541=CARTESIAN_POINT('Ctrl Pts',(4.71371668583241,-44.3280191071452,8.16439679231297));
#35542=CARTESIAN_POINT('Ctrl Pts',(7.07057502873392,-44.1530191071452,4.082198396148));
#35543=CARTESIAN_POINT('Ctrl Pts',(9.42743337163542,-43.9780191071452,-1.69756769845304E-11));
#35544=CARTESIAN_POINT('Ctrl Pts',(7.07057502871922,-43.8030191071452,-4.08219839617346));
#35545=CARTESIAN_POINT('Ctrl Pts',(4.71371668580301,-43.6280191071452,-8.16439679232994));
#35546=CARTESIAN_POINT('Ctrl Pts',(-1.4702867290402E-11,-43.4530191071452,
-8.16439679232146));
#35547=CARTESIAN_POINT('Ctrl Pts',(-1.51301075899711E-11,-213.429517970998,
-8.40164026751963));
#35548=CARTESIAN_POINT('Ctrl Pts',(-4.85068927010199,-213.254517970998,
-8.4016402675109));
#35549=CARTESIAN_POINT('Ctrl Pts',(-7.27603390513785,-213.079517970998,
-4.20082013374671));
#35550=CARTESIAN_POINT('Ctrl Pts',(-9.70137854017372,-212.904517970998,
1.74701493417668E-11));
#35551=CARTESIAN_POINT('Ctrl Pts',(-7.27603390512272,-212.729517970998,
4.20082013377292));
#35552=CARTESIAN_POINT('Ctrl Pts',(-4.85068927007173,-212.554517970998,
8.40164026752836));
#35553=CARTESIAN_POINT('Ctrl Pts',(1.5129078685785E-11,-212.379517970998,
8.40164026751963));
#35554=CARTESIAN_POINT('Ctrl Pts',(4.85068927010198,-212.204517970998,8.4016402675109));
#35555=CARTESIAN_POINT('Ctrl Pts',(7.27603390513785,-212.029517970998,4.20082013374672));
#35556=CARTESIAN_POINT('Ctrl Pts',(9.70137854017372,-211.854517970998,-1.74689612655491E-11));
#35557=CARTESIAN_POINT('Ctrl Pts',(7.27603390512273,-211.679517970998,-4.20082013377291));
#35558=CARTESIAN_POINT('Ctrl Pts',(4.85068927007173,-211.504517970998,-8.40164026752836));
#35559=CARTESIAN_POINT('Ctrl Pts',(-1.51301075899711E-11,-211.329517970998,
-8.40164026751963));
#35560=CARTESIAN_POINT('Ctrl Pts',(-4.85068927010199,-211.154517970998,
-8.4016402675109));
#35561=CARTESIAN_POINT('Ctrl Pts',(-7.27603390513785,-210.979517970998,
-4.20082013374671));
#35562=CARTESIAN_POINT('Ctrl Pts',(-9.70137854017372,-210.804517970998,
1.74701493417668E-11));
#35563=CARTESIAN_POINT('Ctrl Pts',(-7.27603390512272,-210.629517970998,
4.20082013377292));
#35564=CARTESIAN_POINT('Ctrl Pts',(-4.85068927007173,-210.454517970998,
8.40164026752836));
#35565=CARTESIAN_POINT('Ctrl Pts',(1.5129078685785E-11,-210.279517970998,
8.40164026751963));
#35566=CARTESIAN_POINT('Ctrl Pts',(4.85068927010198,-210.104517970998,8.4016402675109));
#35567=CARTESIAN_POINT('Ctrl Pts',(7.27603390513785,-209.929517970998,4.20082013374672));
#35568=CARTESIAN_POINT('Ctrl Pts',(9.70137854017372,-209.754517970998,-1.74689612655491E-11));
#35569=CARTESIAN_POINT('Ctrl Pts',(7.27603390512273,-209.579517970998,-4.20082013377291));
#35570=CARTESIAN_POINT('Ctrl Pts',(4.85068927007173,-209.404517970998,-8.40164026752836));
#35571=CARTESIAN_POINT('Ctrl Pts',(-1.51301075899711E-11,-209.229517970998,
-8.40164026751963));
#35572=CARTESIAN_POINT('Ctrl Pts',(-4.85068927010199,-209.054517970998,
-8.4016402675109));
#35573=CARTESIAN_POINT('Ctrl Pts',(-7.27603390513785,-208.879517970998,
-4.20082013374671));
#35574=CARTESIAN_POINT('Ctrl Pts',(-9.70137854017372,-208.704517970998,
1.74701493417668E-11));
#35575=CARTESIAN_POINT('Ctrl Pts',(-7.27603390512272,-208.529517970998,
4.20082013377292));
#35576=CARTESIAN_POINT('Ctrl Pts',(-4.85068927007173,-208.354517970998,
8.40164026752836));
#35577=CARTESIAN_POINT('Ctrl Pts',(1.5129078685785E-11,-208.179517970998,
8.40164026751963));
#35578=CARTESIAN_POINT('Ctrl Pts',(4.85068927010198,-208.004517970998,8.4016402675109));
#35579=CARTESIAN_POINT('Ctrl Pts',(7.27603390513785,-207.829517970998,4.20082013374672));
#35580=CARTESIAN_POINT('Ctrl Pts',(9.70137854017372,-207.654517970998,-1.74689612655491E-11));
#35581=CARTESIAN_POINT('Ctrl Pts',(7.27603390512273,-207.479517970998,-4.20082013377291));
#35582=CARTESIAN_POINT('Ctrl Pts',(4.85068927007173,-207.304517970998,-8.40164026752836));
#35583=CARTESIAN_POINT('Ctrl Pts',(-1.51301075899711E-11,-207.129517970998,
-8.40164026751963));
#35584=CARTESIAN_POINT('Ctrl Pts',(-4.85068927010199,-206.954517970998,
-8.4016402675109));
#35585=CARTESIAN_POINT('Ctrl Pts',(-7.27603390513785,-206.779517970998,
-4.20082013374671));
#35586=CARTESIAN_POINT('Ctrl Pts',(-9.70137854017372,-206.604517970998,
1.74701493417668E-11));
#35587=CARTESIAN_POINT('Ctrl Pts',(-7.27603390512272,-206.429517970998,
4.20082013377292));
#35588=CARTESIAN_POINT('Ctrl Pts',(-4.85068927007173,-206.254517970998,
8.40164026752836));
#35589=CARTESIAN_POINT('Ctrl Pts',(1.5129078685785E-11,-206.079517970998,
8.40164026751963));
#35590=CARTESIAN_POINT('Ctrl Pts',(4.85068927010198,-205.904517970998,8.4016402675109));
#35591=CARTESIAN_POINT('Ctrl Pts',(7.27603390513785,-205.729517970998,4.20082013374672));
#35592=CARTESIAN_POINT('Ctrl Pts',(9.70137854017372,-205.554517970998,-1.74689612655491E-11));
#35593=CARTESIAN_POINT('Ctrl Pts',(7.27603390512273,-205.379517970998,-4.20082013377291));
#35594=CARTESIAN_POINT('Ctrl Pts',(4.85068927007173,-205.204517970998,-8.40164026752836));
#35595=CARTESIAN_POINT('Ctrl Pts',(-1.51301075899711E-11,-205.029517970998,
-8.40164026751963));
#35596=CARTESIAN_POINT('Ctrl Pts',(-4.85068927010199,-204.854517970998,
-8.4016402675109));
#35597=CARTESIAN_POINT('Ctrl Pts',(-7.27603390513785,-204.679517970998,
-4.20082013374671));
#35598=CARTESIAN_POINT('Ctrl Pts',(-9.70137854017372,-204.504517970998,
1.74701493417668E-11));
#35599=CARTESIAN_POINT('Ctrl Pts',(-7.27603390512272,-204.329517970998,
4.20082013377292));
#35600=CARTESIAN_POINT('Ctrl Pts',(-4.85068927007173,-204.154517970998,
8.40164026752836));
#35601=CARTESIAN_POINT('Ctrl Pts',(1.5129078685785E-11,-203.979517970998,
8.40164026751963));
#35602=CARTESIAN_POINT('Ctrl Pts',(4.85068927010198,-203.804517970998,8.4016402675109));
#35603=CARTESIAN_POINT('Ctrl Pts',(7.27603390513785,-203.629517970998,4.20082013374672));
#35604=CARTESIAN_POINT('Ctrl Pts',(9.70137854017372,-203.454517970998,-1.74689612655491E-11));
#35605=CARTESIAN_POINT('Ctrl Pts',(7.27603390512273,-203.279517970998,-4.20082013377291));
#35606=CARTESIAN_POINT('Ctrl Pts',(4.85068927007173,-203.104517970998,-8.40164026752836));
#35607=CARTESIAN_POINT('Ctrl Pts',(-1.51301075899711E-11,-202.929517970998,
-8.40164026751963));
#35608=CARTESIAN_POINT('Ctrl Pts',(-4.85068927010199,-202.754517970998,
-8.4016402675109));
#35609=CARTESIAN_POINT('Ctrl Pts',(-7.27603390513785,-202.579517970998,
-4.20082013374671));
#35610=CARTESIAN_POINT('Ctrl Pts',(-9.70137854017372,-202.404517970998,
1.74701493417668E-11));
#35611=CARTESIAN_POINT('Ctrl Pts',(-7.27603390512272,-202.229517970998,
4.20082013377292));
#35612=CARTESIAN_POINT('Ctrl Pts',(-4.85068927007173,-202.054517970998,
8.40164026752836));
#35613=CARTESIAN_POINT('Ctrl Pts',(1.5129078685785E-11,-201.879517970998,
8.40164026751963));
#35614=CARTESIAN_POINT('Ctrl Pts',(4.85068927010198,-201.704517970998,8.4016402675109));
#35615=CARTESIAN_POINT('Ctrl Pts',(7.27603390513785,-201.529517970998,4.20082013374672));
#35616=CARTESIAN_POINT('Ctrl Pts',(9.70137854017372,-201.354517970998,-1.74689612655491E-11));
#35617=CARTESIAN_POINT('Ctrl Pts',(7.27603390512273,-201.179517970998,-4.20082013377291));
#35618=CARTESIAN_POINT('Ctrl Pts',(4.85068927007173,-201.004517970998,-8.40164026752836));
#35619=CARTESIAN_POINT('Ctrl Pts',(-1.51301075899711E-11,-200.829517970998,
-8.40164026751963));
#35620=CARTESIAN_POINT('Ctrl Pts',(-4.85068927010199,-200.654517970998,
-8.4016402675109));
#35621=CARTESIAN_POINT('Ctrl Pts',(-7.27603390513785,-200.479517970998,
-4.20082013374671));
#35622=CARTESIAN_POINT('Ctrl Pts',(-9.70137854017372,-200.304517970998,
1.74701493417668E-11));
#35623=CARTESIAN_POINT('Ctrl Pts',(-7.27603390512272,-200.129517970998,
4.20082013377292));
#35624=CARTESIAN_POINT('Ctrl Pts',(-4.85068927007173,-199.954517970998,
8.40164026752836));
#35625=CARTESIAN_POINT('Ctrl Pts',(1.5129078685785E-11,-199.779517970998,
8.40164026751963));
#35626=CARTESIAN_POINT('Ctrl Pts',(4.85068927010198,-199.604517970998,8.4016402675109));
#35627=CARTESIAN_POINT('Ctrl Pts',(7.27603390513785,-199.429517970998,4.20082013374672));
#35628=CARTESIAN_POINT('Ctrl Pts',(9.70137854017372,-199.254517970998,-1.74689612655491E-11));
#35629=CARTESIAN_POINT('Ctrl Pts',(7.27603390512273,-199.079517970998,-4.20082013377291));
#35630=CARTESIAN_POINT('Ctrl Pts',(4.85068927007173,-198.904517970998,-8.40164026752836));
#35631=CARTESIAN_POINT('Ctrl Pts',(-1.51301075899711E-11,-198.729517970998,
-8.40164026751963));
#35632=CARTESIAN_POINT('Ctrl Pts',(-4.85068927010199,-198.554517970998,
-8.4016402675109));
#35633=CARTESIAN_POINT('Ctrl Pts',(-7.27603390513785,-198.379517970998,
-4.20082013374671));
#35634=CARTESIAN_POINT('Ctrl Pts',(-9.70137854017372,-198.204517970998,
1.74701493417668E-11));
#35635=CARTESIAN_POINT('Ctrl Pts',(-7.27603390512272,-198.029517970998,
4.20082013377292));
#35636=CARTESIAN_POINT('Ctrl Pts',(-4.85068927007173,-197.854517970998,
8.40164026752836));
#35637=CARTESIAN_POINT('Ctrl Pts',(1.5129078685785E-11,-197.679517970998,
8.40164026751963));
#35638=CARTESIAN_POINT('Ctrl Pts',(4.85068927010198,-197.504517970998,8.4016402675109));
#35639=CARTESIAN_POINT('Ctrl Pts',(7.27603390513785,-197.329517970998,4.20082013374672));
#35640=CARTESIAN_POINT('Ctrl Pts',(9.70137854017372,-197.154517970998,-1.74689612655491E-11));
#35641=CARTESIAN_POINT('Ctrl Pts',(7.27603390512273,-196.979517970998,-4.20082013377291));
#35642=CARTESIAN_POINT('Ctrl Pts',(4.85068927007173,-196.804517970998,-8.40164026752836));
#35643=CARTESIAN_POINT('Ctrl Pts',(-1.51301075899711E-11,-196.629517970998,
-8.40164026751963));
#35644=CARTESIAN_POINT('Ctrl Pts',(-4.85068927010199,-196.454517970998,
-8.4016402675109));
#35645=CARTESIAN_POINT('Ctrl Pts',(-7.27603390513785,-196.279517970998,
-4.20082013374671));
#35646=CARTESIAN_POINT('Ctrl Pts',(-9.70137854017372,-196.104517970998,
1.74701493417668E-11));
#35647=CARTESIAN_POINT('Ctrl Pts',(-7.27603390512272,-195.929517970998,
4.20082013377292));
#35648=CARTESIAN_POINT('Ctrl Pts',(-4.85068927007173,-195.754517970998,
8.40164026752836));
#35649=CARTESIAN_POINT('Ctrl Pts',(1.5129078685785E-11,-195.579517970998,
8.40164026751963));
#35650=CARTESIAN_POINT('Ctrl Pts',(4.85068927010198,-195.404517970998,8.4016402675109));
#35651=CARTESIAN_POINT('Ctrl Pts',(7.27603390513785,-195.229517970998,4.20082013374672));
#35652=CARTESIAN_POINT('Ctrl Pts',(9.70137854017372,-195.054517970998,-1.74689612655491E-11));
#35653=CARTESIAN_POINT('Ctrl Pts',(7.27603390512273,-194.879517970998,-4.20082013377291));
#35654=CARTESIAN_POINT('Ctrl Pts',(4.85068927007173,-194.704517970998,-8.40164026752836));
#35655=CARTESIAN_POINT('Ctrl Pts',(-1.51301075899711E-11,-194.529517970998,
-8.40164026751963));
#35656=CARTESIAN_POINT('Ctrl Pts',(-4.85068927010199,-194.354517970998,
-8.4016402675109));
#35657=CARTESIAN_POINT('Ctrl Pts',(-7.27603390513785,-194.179517970998,
-4.20082013374671));
#35658=CARTESIAN_POINT('Ctrl Pts',(-9.70137854017372,-194.004517970998,
1.74701493417668E-11));
#35659=CARTESIAN_POINT('Ctrl Pts',(-7.27603390512272,-193.829517970998,
4.20082013377292));
#35660=CARTESIAN_POINT('Ctrl Pts',(-4.85068927007173,-193.654517970998,
8.40164026752836));
#35661=CARTESIAN_POINT('Ctrl Pts',(1.5129078685785E-11,-193.479517970998,
8.40164026751963));
#35662=CARTESIAN_POINT('Ctrl Pts',(4.85068927010198,-193.304517970998,8.4016402675109));
#35663=CARTESIAN_POINT('Ctrl Pts',(7.27603390513785,-193.129517970998,4.20082013374672));
#35664=CARTESIAN_POINT('Ctrl Pts',(9.70137854017372,-192.954517970998,-1.74689612655491E-11));
#35665=CARTESIAN_POINT('Ctrl Pts',(7.27603390512273,-192.779517970998,-4.20082013377291));
#35666=CARTESIAN_POINT('Ctrl Pts',(4.85068927007173,-192.604517970998,-8.40164026752836));
#35667=CARTESIAN_POINT('Ctrl Pts',(-1.51301075899711E-11,-192.429517970998,
-8.40164026751963));
#35668=CARTESIAN_POINT('Ctrl Pts',(-4.85068927010199,-192.254517970998,
-8.4016402675109));
#35669=CARTESIAN_POINT('Ctrl Pts',(-7.27603390513785,-192.079517970998,
-4.20082013374671));
#35670=CARTESIAN_POINT('Ctrl Pts',(-9.70137854017372,-191.904517970998,
1.74701493417668E-11));
#35671=CARTESIAN_POINT('Ctrl Pts',(-7.27603390512272,-191.729517970998,
4.20082013377292));
#35672=CARTESIAN_POINT('Ctrl Pts',(-4.85068927007173,-191.554517970998,
8.40164026752836));
#35673=CARTESIAN_POINT('Ctrl Pts',(1.5129078685785E-11,-191.379517970998,
8.40164026751963));
#35674=CARTESIAN_POINT('Ctrl Pts',(4.85068927010198,-191.204517970998,8.4016402675109));
#35675=CARTESIAN_POINT('Ctrl Pts',(7.27603390513785,-191.029517970998,4.20082013374672));
#35676=CARTESIAN_POINT('Ctrl Pts',(9.70137854017372,-190.854517970998,-1.74689612655491E-11));
#35677=CARTESIAN_POINT('Ctrl Pts',(7.27603390512273,-190.679517970998,-4.20082013377291));
#35678=CARTESIAN_POINT('Ctrl Pts',(4.85068927007173,-190.504517970998,-8.40164026752836));
#35679=CARTESIAN_POINT('Ctrl Pts',(-1.51301075899711E-11,-190.329517970998,
-8.40164026751963));
#35680=CARTESIAN_POINT('Ctrl Pts',(-4.85068927010199,-190.154517970998,
-8.4016402675109));
#35681=CARTESIAN_POINT('Ctrl Pts',(-7.27603390513785,-189.979517970998,
-4.20082013374671));
#35682=CARTESIAN_POINT('Ctrl Pts',(-9.70137854017372,-189.804517970998,
1.74701493417668E-11));
#35683=CARTESIAN_POINT('Ctrl Pts',(-7.27603390512272,-189.629517970998,
4.20082013377292));
#35684=CARTESIAN_POINT('Ctrl Pts',(-4.85068927007173,-189.454517970998,
8.40164026752836));
#35685=CARTESIAN_POINT('Ctrl Pts',(1.5129078685785E-11,-189.279517970998,
8.40164026751963));
#35686=CARTESIAN_POINT('Ctrl Pts',(4.85068927010198,-189.104517970998,8.4016402675109));
#35687=CARTESIAN_POINT('Ctrl Pts',(7.27603390513785,-188.929517970998,4.20082013374672));
#35688=CARTESIAN_POINT('Ctrl Pts',(9.70137854017372,-188.754517970998,-1.74689612655491E-11));
#35689=CARTESIAN_POINT('Ctrl Pts',(7.27603390512273,-188.579517970998,-4.20082013377291));
#35690=CARTESIAN_POINT('Ctrl Pts',(4.85068927007173,-188.404517970998,-8.40164026752836));
#35691=CARTESIAN_POINT('Ctrl Pts',(-1.51301075899711E-11,-188.229517970998,
-8.40164026751963));
#35692=CARTESIAN_POINT('Ctrl Pts',(-4.85068927010199,-188.054517970998,
-8.4016402675109));
#35693=CARTESIAN_POINT('Ctrl Pts',(-7.27603390513785,-187.879517970998,
-4.20082013374671));
#35694=CARTESIAN_POINT('Ctrl Pts',(-9.70137854017372,-187.704517970998,
1.74701493417668E-11));
#35695=CARTESIAN_POINT('Ctrl Pts',(-7.27603390512272,-187.529517970998,
4.20082013377292));
#35696=CARTESIAN_POINT('Ctrl Pts',(-4.85068927007173,-187.354517970998,
8.40164026752836));
#35697=CARTESIAN_POINT('Ctrl Pts',(1.5129078685785E-11,-187.179517970998,
8.40164026751963));
#35698=CARTESIAN_POINT('Ctrl Pts',(4.85068927010198,-187.004517970998,8.4016402675109));
#35699=CARTESIAN_POINT('Ctrl Pts',(7.27603390513785,-186.829517970998,4.20082013374672));
#35700=CARTESIAN_POINT('Ctrl Pts',(9.70137854017372,-186.654517970998,-1.74689612655491E-11));
#35701=CARTESIAN_POINT('Ctrl Pts',(7.27603390512273,-186.479517970998,-4.20082013377291));
#35702=CARTESIAN_POINT('Ctrl Pts',(4.85068927007173,-186.304517970998,-8.40164026752836));
#35703=CARTESIAN_POINT('Ctrl Pts',(-1.51301075899711E-11,-186.129517970998,
-8.40164026751963));
#35704=CARTESIAN_POINT('Ctrl Pts',(-4.85068927010199,-185.954517970998,
-8.4016402675109));
#35705=CARTESIAN_POINT('Ctrl Pts',(-7.27603390513785,-185.779517970998,
-4.20082013374671));
#35706=CARTESIAN_POINT('Ctrl Pts',(-9.70137854017372,-185.604517970998,
1.74701493417668E-11));
#35707=CARTESIAN_POINT('Ctrl Pts',(-7.27603390512272,-185.429517970998,
4.20082013377292));
#35708=CARTESIAN_POINT('Ctrl Pts',(-4.85068927007173,-185.254517970998,
8.40164026752836));
#35709=CARTESIAN_POINT('Ctrl Pts',(1.5129078685785E-11,-185.079517970998,
8.40164026751963));
#35710=CARTESIAN_POINT('Ctrl Pts',(4.85068927010198,-184.904517970998,8.4016402675109));
#35711=CARTESIAN_POINT('Ctrl Pts',(7.27603390513785,-184.729517970998,4.20082013374672));
#35712=CARTESIAN_POINT('Ctrl Pts',(9.70137854017372,-184.554517970998,-1.74689612655491E-11));
#35713=CARTESIAN_POINT('Ctrl Pts',(7.27603390512273,-184.379517970998,-4.20082013377291));
#35714=CARTESIAN_POINT('Ctrl Pts',(4.85068927007173,-184.204517970998,-8.40164026752836));
#35715=CARTESIAN_POINT('Ctrl Pts',(-1.51301075899711E-11,-184.029517970998,
-8.40164026751963));
#35716=CARTESIAN_POINT('Ctrl Pts',(-4.85068927010199,-183.854517970998,
-8.4016402675109));
#35717=CARTESIAN_POINT('Ctrl Pts',(-7.27603390513785,-183.679517970998,
-4.20082013374671));
#35718=CARTESIAN_POINT('Ctrl Pts',(-9.70137854017372,-183.504517970998,
1.74701493417668E-11));
#35719=CARTESIAN_POINT('Ctrl Pts',(-7.27603390512272,-183.329517970998,
4.20082013377292));
#35720=CARTESIAN_POINT('Ctrl Pts',(-4.85068927007173,-183.154517970998,
8.40164026752836));
#35721=CARTESIAN_POINT('Ctrl Pts',(1.5129078685785E-11,-182.979517970998,
8.40164026751963));
#35722=CARTESIAN_POINT('Ctrl Pts',(4.85068927010198,-182.804517970998,8.4016402675109));
#35723=CARTESIAN_POINT('Ctrl Pts',(7.27603390513785,-182.629517970998,4.20082013374672));
#35724=CARTESIAN_POINT('Ctrl Pts',(9.70137854017372,-182.454517970998,-1.74689612655491E-11));
#35725=CARTESIAN_POINT('Ctrl Pts',(7.27603390512273,-182.279517970998,-4.20082013377291));
#35726=CARTESIAN_POINT('Ctrl Pts',(4.85068927007173,-182.104517970998,-8.40164026752836));
#35727=CARTESIAN_POINT('Ctrl Pts',(-1.51301075899711E-11,-181.929517970998,
-8.40164026751963));
#35728=CARTESIAN_POINT('Ctrl Pts',(-4.85068927010199,-181.754517970998,
-8.4016402675109));
#35729=CARTESIAN_POINT('Ctrl Pts',(-7.27603390513785,-181.579517970998,
-4.20082013374671));
#35730=CARTESIAN_POINT('Ctrl Pts',(-9.70137854017372,-181.404517970998,
1.74701493417668E-11));
#35731=CARTESIAN_POINT('Ctrl Pts',(-7.27603390512272,-181.229517970998,
4.20082013377292));
#35732=CARTESIAN_POINT('Ctrl Pts',(-4.85068927007173,-181.054517970998,
8.40164026752836));
#35733=CARTESIAN_POINT('Ctrl Pts',(1.5129078685785E-11,-180.879517970998,
8.40164026751963));
#35734=CARTESIAN_POINT('Ctrl Pts',(4.85068927010198,-180.704517970998,8.4016402675109));
#35735=CARTESIAN_POINT('Ctrl Pts',(7.27603390513785,-180.529517970998,4.20082013374672));
#35736=CARTESIAN_POINT('Ctrl Pts',(9.70137854017372,-180.354517970998,-1.74689612655491E-11));
#35737=CARTESIAN_POINT('Ctrl Pts',(7.27603390512273,-180.179517970998,-4.20082013377291));
#35738=CARTESIAN_POINT('Ctrl Pts',(4.85068927007173,-180.004517970998,-8.40164026752836));
#35739=CARTESIAN_POINT('Ctrl Pts',(-1.51301075899711E-11,-179.829517970998,
-8.40164026751963));
#35740=CARTESIAN_POINT('Ctrl Pts',(-4.85068927010199,-179.654517970998,
-8.4016402675109));
#35741=CARTESIAN_POINT('Ctrl Pts',(-7.27603390513785,-179.479517970998,
-4.20082013374671));
#35742=CARTESIAN_POINT('Ctrl Pts',(-9.70137854017372,-179.304517970998,
1.74701493417668E-11));
#35743=CARTESIAN_POINT('Ctrl Pts',(-7.27603390512272,-179.129517970998,
4.20082013377292));
#35744=CARTESIAN_POINT('Ctrl Pts',(-4.85068927007173,-178.954517970998,
8.40164026752836));
#35745=CARTESIAN_POINT('Ctrl Pts',(1.5129078685785E-11,-178.779517970998,
8.40164026751963));
#35746=CARTESIAN_POINT('Ctrl Pts',(4.85068927010198,-178.604517970998,8.4016402675109));
#35747=CARTESIAN_POINT('Ctrl Pts',(7.27603390513785,-178.429517970998,4.20082013374672));
#35748=CARTESIAN_POINT('Ctrl Pts',(9.70137854017372,-178.254517970998,-1.74689612655491E-11));
#35749=CARTESIAN_POINT('Ctrl Pts',(7.27603390512273,-178.079517970998,-4.20082013377291));
#35750=CARTESIAN_POINT('Ctrl Pts',(4.85068927007173,-177.904517970998,-8.40164026752836));
#35751=CARTESIAN_POINT('Ctrl Pts',(-1.51301075899711E-11,-177.729517970998,
-8.40164026751963));
#35752=CARTESIAN_POINT('Ctrl Pts',(-4.85068927010199,-177.554517970998,
-8.4016402675109));
#35753=CARTESIAN_POINT('Ctrl Pts',(-7.27603390513785,-177.379517970998,
-4.20082013374671));
#35754=CARTESIAN_POINT('Ctrl Pts',(-9.70137854017372,-177.204517970998,
1.74701493417668E-11));
#35755=CARTESIAN_POINT('Ctrl Pts',(-7.27603390512272,-177.029517970998,
4.20082013377292));
#35756=CARTESIAN_POINT('Ctrl Pts',(-4.85068927007173,-176.854517970998,
8.40164026752836));
#35757=CARTESIAN_POINT('Ctrl Pts',(1.5129078685785E-11,-176.679517970998,
8.40164026751963));
#35758=CARTESIAN_POINT('Ctrl Pts',(4.85068927010198,-176.504517970998,8.4016402675109));
#35759=CARTESIAN_POINT('Ctrl Pts',(7.27603390513785,-176.329517970998,4.20082013374672));
#35760=CARTESIAN_POINT('Ctrl Pts',(9.70137854017372,-176.154517970998,-1.74689612655491E-11));
#35761=CARTESIAN_POINT('Ctrl Pts',(7.27603390512273,-175.979517970998,-4.20082013377291));
#35762=CARTESIAN_POINT('Ctrl Pts',(4.85068927007173,-175.804517970998,-8.40164026752836));
#35763=CARTESIAN_POINT('Ctrl Pts',(-1.51301075899711E-11,-175.629517970998,
-8.40164026751963));
#35764=CARTESIAN_POINT('Ctrl Pts',(-4.85068927010199,-175.454517970998,
-8.4016402675109));
#35765=CARTESIAN_POINT('Ctrl Pts',(-7.27603390513785,-175.279517970998,
-4.20082013374671));
#35766=CARTESIAN_POINT('Ctrl Pts',(-9.70137854017372,-175.104517970998,
1.74701493417668E-11));
#35767=CARTESIAN_POINT('Ctrl Pts',(-7.27603390512272,-174.929517970998,
4.20082013377292));
#35768=CARTESIAN_POINT('Ctrl Pts',(-4.85068927007173,-174.754517970998,
8.40164026752836));
#35769=CARTESIAN_POINT('Ctrl Pts',(1.5129078685785E-11,-174.579517970998,
8.40164026751963));
#35770=CARTESIAN_POINT('Ctrl Pts',(4.85068927010198,-174.404517970998,8.4016402675109));
#35771=CARTESIAN_POINT('Ctrl Pts',(7.27603390513785,-174.229517970998,4.20082013374672));
#35772=CARTESIAN_POINT('Ctrl Pts',(9.70137854017372,-174.054517970998,-1.74689612655491E-11));
#35773=CARTESIAN_POINT('Ctrl Pts',(7.27603390512273,-173.879517970998,-4.20082013377291));
#35774=CARTESIAN_POINT('Ctrl Pts',(4.85068927007173,-173.704517970998,-8.40164026752836));
#35775=CARTESIAN_POINT('Ctrl Pts',(-1.51301075899711E-11,-173.529517970998,
-8.40164026751963));
#35776=CARTESIAN_POINT('Ctrl Pts',(-4.85068927010199,-173.354517970998,
-8.4016402675109));
#35777=CARTESIAN_POINT('Ctrl Pts',(-7.27603390513785,-173.179517970998,
-4.20082013374671));
#35778=CARTESIAN_POINT('Ctrl Pts',(-9.70137854017372,-173.004517970998,
1.74701493417668E-11));
#35779=CARTESIAN_POINT('Ctrl Pts',(-7.27603390512272,-172.829517970998,
4.20082013377292));
#35780=CARTESIAN_POINT('Ctrl Pts',(-4.85068927007173,-172.654517970998,
8.40164026752836));
#35781=CARTESIAN_POINT('Ctrl Pts',(1.5129078685785E-11,-172.479517970998,
8.40164026751963));
#35782=CARTESIAN_POINT('Ctrl Pts',(4.85068927010198,-172.304517970998,8.4016402675109));
#35783=CARTESIAN_POINT('Ctrl Pts',(7.27603390513785,-172.129517970998,4.20082013374672));
#35784=CARTESIAN_POINT('Ctrl Pts',(9.70137854017372,-171.954517970998,-1.74689612655491E-11));
#35785=CARTESIAN_POINT('Ctrl Pts',(7.27603390512273,-171.779517970998,-4.20082013377291));
#35786=CARTESIAN_POINT('Ctrl Pts',(4.85068927007173,-171.604517970998,-8.40164026752836));
#35787=CARTESIAN_POINT('Ctrl Pts',(-1.51301075899711E-11,-171.429517970998,
-8.40164026751963));
#35788=CARTESIAN_POINT('Ctrl Pts',(-4.85068927010199,-171.254517970998,
-8.4016402675109));
#35789=CARTESIAN_POINT('Ctrl Pts',(-7.27603390513785,-171.079517970998,
-4.20082013374671));
#35790=CARTESIAN_POINT('Ctrl Pts',(-9.70137854017372,-170.904517970998,
1.74701493417668E-11));
#35791=CARTESIAN_POINT('Ctrl Pts',(-7.27603390512272,-170.729517970998,
4.20082013377292));
#35792=CARTESIAN_POINT('Ctrl Pts',(-4.85068927007173,-170.554517970998,
8.40164026752836));
#35793=CARTESIAN_POINT('Ctrl Pts',(1.5129078685785E-11,-170.379517970998,
8.40164026751963));
#35794=CARTESIAN_POINT('Ctrl Pts',(4.85068927010198,-170.204517970998,8.4016402675109));
#35795=CARTESIAN_POINT('Ctrl Pts',(7.27603390513785,-170.029517970998,4.20082013374672));
#35796=CARTESIAN_POINT('Ctrl Pts',(9.70137854017372,-169.854517970998,-1.74689612655491E-11));
#35797=CARTESIAN_POINT('Ctrl Pts',(7.27603390512273,-169.679517970998,-4.20082013377291));
#35798=CARTESIAN_POINT('Ctrl Pts',(4.85068927007173,-169.504517970998,-8.40164026752836));
#35799=CARTESIAN_POINT('Ctrl Pts',(-1.51301075899711E-11,-169.329517970998,
-8.40164026751963));
#35800=CARTESIAN_POINT('Ctrl Pts',(-4.85068927010199,-169.154517970998,
-8.4016402675109));
#35801=CARTESIAN_POINT('Ctrl Pts',(-7.27603390513785,-168.979517970998,
-4.20082013374671));
#35802=CARTESIAN_POINT('Ctrl Pts',(-9.70137854017372,-168.804517970998,
1.74701493417668E-11));
#35803=CARTESIAN_POINT('Ctrl Pts',(-7.27603390512272,-168.629517970998,
4.20082013377292));
#35804=CARTESIAN_POINT('Ctrl Pts',(-4.85068927007173,-168.454517970998,
8.40164026752836));
#35805=CARTESIAN_POINT('Ctrl Pts',(1.5129078685785E-11,-168.279517970998,
8.40164026751963));
#35806=CARTESIAN_POINT('Ctrl Pts',(4.85068927010198,-168.104517970998,8.4016402675109));
#35807=CARTESIAN_POINT('Ctrl Pts',(7.27603390513785,-167.929517970998,4.20082013374672));
#35808=CARTESIAN_POINT('Ctrl Pts',(9.70137854017372,-167.754517970998,-1.74689612655491E-11));
#35809=CARTESIAN_POINT('Ctrl Pts',(7.27603390512273,-167.579517970998,-4.20082013377291));
#35810=CARTESIAN_POINT('Ctrl Pts',(4.85068927007173,-167.404517970998,-8.40164026752836));
#35811=CARTESIAN_POINT('Ctrl Pts',(-1.51301075899711E-11,-167.229517970998,
-8.40164026751963));
#35812=CARTESIAN_POINT('Ctrl Pts',(-4.85068927010199,-167.054517970998,
-8.4016402675109));
#35813=CARTESIAN_POINT('Ctrl Pts',(-7.27603390513785,-166.879517970998,
-4.20082013374671));
#35814=CARTESIAN_POINT('Ctrl Pts',(-9.70137854017372,-166.704517970998,
1.74701493417668E-11));
#35815=CARTESIAN_POINT('Ctrl Pts',(-7.27603390512272,-166.529517970998,
4.20082013377292));
#35816=CARTESIAN_POINT('Ctrl Pts',(-4.85068927007173,-166.354517970998,
8.40164026752836));
#35817=CARTESIAN_POINT('Ctrl Pts',(1.5129078685785E-11,-166.179517970998,
8.40164026751963));
#35818=CARTESIAN_POINT('Ctrl Pts',(4.85068927010198,-166.004517970998,8.4016402675109));
#35819=CARTESIAN_POINT('Ctrl Pts',(7.27603390513785,-165.829517970998,4.20082013374672));
#35820=CARTESIAN_POINT('Ctrl Pts',(9.70137854017372,-165.654517970998,-1.74689612655491E-11));
#35821=CARTESIAN_POINT('Ctrl Pts',(7.27603390512273,-165.479517970998,-4.20082013377291));
#35822=CARTESIAN_POINT('Ctrl Pts',(4.85068927007173,-165.304517970998,-8.40164026752836));
#35823=CARTESIAN_POINT('Ctrl Pts',(-1.51301075899711E-11,-165.129517970998,
-8.40164026751963));
#35824=CARTESIAN_POINT('Ctrl Pts',(-4.85068927010199,-164.954517970998,
-8.4016402675109));
#35825=CARTESIAN_POINT('Ctrl Pts',(-7.27603390513785,-164.779517970998,
-4.20082013374671));
#35826=CARTESIAN_POINT('Ctrl Pts',(-9.70137854017372,-164.604517970998,
1.74701493417668E-11));
#35827=CARTESIAN_POINT('Ctrl Pts',(-7.27603390512272,-164.429517970998,
4.20082013377292));
#35828=CARTESIAN_POINT('Ctrl Pts',(-4.85068927007173,-164.254517970998,
8.40164026752836));
#35829=CARTESIAN_POINT('Ctrl Pts',(1.5129078685785E-11,-164.079517970998,
8.40164026751963));
#35830=CARTESIAN_POINT('Ctrl Pts',(4.85068927010198,-163.904517970998,8.4016402675109));
#35831=CARTESIAN_POINT('Ctrl Pts',(7.27603390513785,-163.729517970998,4.20082013374672));
#35832=CARTESIAN_POINT('Ctrl Pts',(9.70137854017372,-163.554517970998,-1.74689612655491E-11));
#35833=CARTESIAN_POINT('Ctrl Pts',(7.27603390512273,-163.379517970998,-4.20082013377291));
#35834=CARTESIAN_POINT('Ctrl Pts',(4.85068927007173,-163.204517970998,-8.40164026752836));
#35835=CARTESIAN_POINT('Ctrl Pts',(-1.51301075899711E-11,-163.029517970998,
-8.40164026751963));
#35836=CARTESIAN_POINT('Ctrl Pts',(-4.85068927010199,-162.854517970998,
-8.4016402675109));
#35837=CARTESIAN_POINT('Ctrl Pts',(-7.27603390513785,-162.679517970998,
-4.20082013374671));
#35838=CARTESIAN_POINT('Ctrl Pts',(-9.70137854017372,-162.504517970998,
1.74701493417668E-11));
#35839=CARTESIAN_POINT('Ctrl Pts',(-7.27603390512272,-162.329517970998,
4.20082013377292));
#35840=CARTESIAN_POINT('Ctrl Pts',(-4.85068927007173,-162.154517970998,
8.40164026752836));
#35841=CARTESIAN_POINT('Ctrl Pts',(1.5129078685785E-11,-161.979517970998,
8.40164026751963));
#35842=CARTESIAN_POINT('Ctrl Pts',(4.85068927010198,-161.804517970998,8.4016402675109));
#35843=CARTESIAN_POINT('Ctrl Pts',(7.27603390513785,-161.629517970998,4.20082013374672));
#35844=CARTESIAN_POINT('Ctrl Pts',(9.70137854017372,-161.454517970998,-1.74689612655491E-11));
#35845=CARTESIAN_POINT('Ctrl Pts',(7.27603390512273,-161.279517970998,-4.20082013377291));
#35846=CARTESIAN_POINT('Ctrl Pts',(4.85068927007173,-161.104517970998,-8.40164026752836));
#35847=CARTESIAN_POINT('Ctrl Pts',(-1.51301075899711E-11,-160.929517970998,
-8.40164026751963));
#35848=CARTESIAN_POINT('Ctrl Pts',(-4.85068927010199,-160.754517970998,
-8.4016402675109));
#35849=CARTESIAN_POINT('Ctrl Pts',(-7.27603390513785,-160.579517970998,
-4.20082013374671));
#35850=CARTESIAN_POINT('Ctrl Pts',(-9.70137854017372,-160.404517970998,
1.74701493417668E-11));
#35851=CARTESIAN_POINT('Ctrl Pts',(-7.27603390512272,-160.229517970998,
4.20082013377292));
#35852=CARTESIAN_POINT('Ctrl Pts',(-4.85068927007173,-160.054517970998,
8.40164026752836));
#35853=CARTESIAN_POINT('Ctrl Pts',(1.5129078685785E-11,-159.879517970998,
8.40164026751963));
#35854=CARTESIAN_POINT('Ctrl Pts',(4.85068927010198,-159.704517970998,8.4016402675109));
#35855=CARTESIAN_POINT('Ctrl Pts',(7.27603390513785,-159.529517970998,4.20082013374672));
#35856=CARTESIAN_POINT('Ctrl Pts',(9.70137854017372,-159.354517970998,-1.74689612655491E-11));
#35857=CARTESIAN_POINT('Ctrl Pts',(7.27603390512273,-159.179517970998,-4.20082013377291));
#35858=CARTESIAN_POINT('Ctrl Pts',(4.85068927007173,-159.004517970998,-8.40164026752836));
#35859=CARTESIAN_POINT('Ctrl Pts',(-1.51301075899711E-11,-158.829517970998,
-8.40164026751963));
#35860=CARTESIAN_POINT('Ctrl Pts',(-4.85068927010199,-158.654517970998,
-8.4016402675109));
#35861=CARTESIAN_POINT('Ctrl Pts',(-7.27603390513785,-158.479517970998,
-4.20082013374671));
#35862=CARTESIAN_POINT('Ctrl Pts',(-9.70137854017372,-158.304517970998,
1.74701493417668E-11));
#35863=CARTESIAN_POINT('Ctrl Pts',(-7.27603390512272,-158.129517970998,
4.20082013377292));
#35864=CARTESIAN_POINT('Ctrl Pts',(-4.85068927007173,-157.954517970998,
8.40164026752836));
#35865=CARTESIAN_POINT('Ctrl Pts',(1.5129078685785E-11,-157.779517970998,
8.40164026751963));
#35866=CARTESIAN_POINT('Ctrl Pts',(4.85068927010198,-157.604517970998,8.4016402675109));
#35867=CARTESIAN_POINT('Ctrl Pts',(7.27603390513785,-157.429517970998,4.20082013374672));
#35868=CARTESIAN_POINT('Ctrl Pts',(9.70137854017372,-157.254517970998,-1.74689612655491E-11));
#35869=CARTESIAN_POINT('Ctrl Pts',(7.27603390512273,-157.079517970998,-4.20082013377291));
#35870=CARTESIAN_POINT('Ctrl Pts',(4.85068927007173,-156.904517970998,-8.40164026752836));
#35871=CARTESIAN_POINT('Ctrl Pts',(-1.51301075899711E-11,-156.729517970998,
-8.40164026751963));
#35872=CARTESIAN_POINT('Ctrl Pts',(-4.85068927010199,-156.554517970998,
-8.4016402675109));
#35873=CARTESIAN_POINT('Ctrl Pts',(-7.27603390513785,-156.379517970998,
-4.20082013374671));
#35874=CARTESIAN_POINT('Ctrl Pts',(-9.70137854017372,-156.204517970998,
1.74701493417668E-11));
#35875=CARTESIAN_POINT('Ctrl Pts',(-7.27603390512272,-156.029517970998,
4.20082013377292));
#35876=CARTESIAN_POINT('Ctrl Pts',(-4.85068927007173,-155.854517970998,
8.40164026752836));
#35877=CARTESIAN_POINT('Ctrl Pts',(1.5129078685785E-11,-155.679517970998,
8.40164026751963));
#35878=CARTESIAN_POINT('Ctrl Pts',(4.85068927010198,-155.504517970998,8.4016402675109));
#35879=CARTESIAN_POINT('Ctrl Pts',(7.27603390513785,-155.329517970998,4.20082013374672));
#35880=CARTESIAN_POINT('Ctrl Pts',(9.70137854017372,-155.154517970998,-1.74689612655491E-11));
#35881=CARTESIAN_POINT('Ctrl Pts',(7.27603390512273,-154.979517970998,-4.20082013377291));
#35882=CARTESIAN_POINT('Ctrl Pts',(4.85068927007173,-154.804517970998,-8.40164026752836));
#35883=CARTESIAN_POINT('Ctrl Pts',(-1.51301075899711E-11,-154.629517970998,
-8.40164026751963));
#35884=CARTESIAN_POINT('Ctrl Pts',(-4.85068927010199,-154.454517970998,
-8.4016402675109));
#35885=CARTESIAN_POINT('Ctrl Pts',(-7.27603390513785,-154.279517970998,
-4.20082013374671));
#35886=CARTESIAN_POINT('Ctrl Pts',(-9.70137854017372,-154.104517970998,
1.74701493417668E-11));
#35887=CARTESIAN_POINT('Ctrl Pts',(-7.27603390512272,-153.929517970998,
4.20082013377292));
#35888=CARTESIAN_POINT('Ctrl Pts',(-4.85068927007173,-153.754517970998,
8.40164026752836));
#35889=CARTESIAN_POINT('Ctrl Pts',(1.5129078685785E-11,-153.579517970998,
8.40164026751963));
#35890=CARTESIAN_POINT('Ctrl Pts',(4.85068927010198,-153.404517970998,8.4016402675109));
#35891=CARTESIAN_POINT('Ctrl Pts',(7.27603390513785,-153.229517970998,4.20082013374672));
#35892=CARTESIAN_POINT('Ctrl Pts',(9.70137854017372,-153.054517970998,-1.74689612655491E-11));
#35893=CARTESIAN_POINT('Ctrl Pts',(7.27603390512273,-152.879517970998,-4.20082013377291));
#35894=CARTESIAN_POINT('Ctrl Pts',(4.85068927007173,-152.704517970998,-8.40164026752836));
#35895=CARTESIAN_POINT('Ctrl Pts',(-1.51301075899711E-11,-152.529517970998,
-8.40164026751963));
#35896=CARTESIAN_POINT('Ctrl Pts',(-4.85068927010199,-152.354517970998,
-8.4016402675109));
#35897=CARTESIAN_POINT('Ctrl Pts',(-7.27603390513785,-152.179517970998,
-4.20082013374671));
#35898=CARTESIAN_POINT('Ctrl Pts',(-9.70137854017372,-152.004517970998,
1.74701493417668E-11));
#35899=CARTESIAN_POINT('Ctrl Pts',(-7.27603390512272,-151.829517970998,
4.20082013377292));
#35900=CARTESIAN_POINT('Ctrl Pts',(-4.85068927007173,-151.654517970998,
8.40164026752836));
#35901=CARTESIAN_POINT('Ctrl Pts',(1.5129078685785E-11,-151.479517970998,
8.40164026751963));
#35902=CARTESIAN_POINT('Ctrl Pts',(4.85068927010198,-151.304517970998,8.4016402675109));
#35903=CARTESIAN_POINT('Ctrl Pts',(7.27603390513785,-151.129517970998,4.20082013374672));
#35904=CARTESIAN_POINT('Ctrl Pts',(9.70137854017372,-150.954517970998,-1.74689612655491E-11));
#35905=CARTESIAN_POINT('Ctrl Pts',(7.27603390512273,-150.779517970998,-4.20082013377291));
#35906=CARTESIAN_POINT('Ctrl Pts',(4.85068927007173,-150.604517970998,-8.40164026752836));
#35907=CARTESIAN_POINT('Ctrl Pts',(-1.51301075899711E-11,-150.429517970998,
-8.40164026751963));
#35908=CARTESIAN_POINT('Ctrl Pts',(-4.85068927010199,-150.254517970998,
-8.4016402675109));
#35909=CARTESIAN_POINT('Ctrl Pts',(-7.27603390513785,-150.079517970998,
-4.20082013374671));
#35910=CARTESIAN_POINT('Ctrl Pts',(-9.70137854017372,-149.904517970998,
1.74701493417668E-11));
#35911=CARTESIAN_POINT('Ctrl Pts',(-7.27603390512272,-149.729517970998,
4.20082013377292));
#35912=CARTESIAN_POINT('Ctrl Pts',(-4.85068927007173,-149.554517970998,
8.40164026752836));
#35913=CARTESIAN_POINT('Ctrl Pts',(1.5129078685785E-11,-149.379517970998,
8.40164026751963));
#35914=CARTESIAN_POINT('Ctrl Pts',(4.85068927010198,-149.204517970998,8.4016402675109));
#35915=CARTESIAN_POINT('Ctrl Pts',(7.27603390513785,-149.029517970998,4.20082013374672));
#35916=CARTESIAN_POINT('Ctrl Pts',(9.70137854017372,-148.854517970998,-1.74689612655491E-11));
#35917=CARTESIAN_POINT('Ctrl Pts',(7.27603390512273,-148.679517970998,-4.20082013377291));
#35918=CARTESIAN_POINT('Ctrl Pts',(4.85068927007173,-148.504517970998,-8.40164026752836));
#35919=CARTESIAN_POINT('Ctrl Pts',(-1.51301075899711E-11,-148.329517970998,
-8.40164026751963));
#35920=CARTESIAN_POINT('Ctrl Pts',(-4.85068927010199,-148.154517970998,
-8.4016402675109));
#35921=CARTESIAN_POINT('Ctrl Pts',(-7.27603390513785,-147.979517970998,
-4.20082013374671));
#35922=CARTESIAN_POINT('Ctrl Pts',(-9.70137854017372,-147.804517970998,
1.74701493417668E-11));
#35923=CARTESIAN_POINT('Ctrl Pts',(-7.27603390512272,-147.629517970998,
4.20082013377292));
#35924=CARTESIAN_POINT('Ctrl Pts',(-4.85068927007173,-147.454517970998,
8.40164026752836));
#35925=CARTESIAN_POINT('Ctrl Pts',(1.5129078685785E-11,-147.279517970998,
8.40164026751963));
#35926=CARTESIAN_POINT('Ctrl Pts',(4.85068927010198,-147.104517970998,8.4016402675109));
#35927=CARTESIAN_POINT('Ctrl Pts',(7.27603390513785,-146.929517970998,4.20082013374672));
#35928=CARTESIAN_POINT('Ctrl Pts',(9.70137854017372,-146.754517970998,-1.74689612655491E-11));
#35929=CARTESIAN_POINT('Ctrl Pts',(7.27603390512273,-146.579517970998,-4.20082013377291));
#35930=CARTESIAN_POINT('Ctrl Pts',(4.85068927007173,-146.404517970998,-8.40164026752836));
#35931=CARTESIAN_POINT('Ctrl Pts',(-1.51301075899711E-11,-146.229517970998,
-8.40164026751963));
#35932=CARTESIAN_POINT('Ctrl Pts',(-4.85068927010199,-146.054517970998,
-8.4016402675109));
#35933=CARTESIAN_POINT('Ctrl Pts',(-7.27603390513785,-145.879517970998,
-4.20082013374671));
#35934=CARTESIAN_POINT('Ctrl Pts',(-9.70137854017372,-145.704517970998,
1.74701493417668E-11));
#35935=CARTESIAN_POINT('Ctrl Pts',(-7.27603390512272,-145.529517970998,
4.20082013377292));
#35936=CARTESIAN_POINT('Ctrl Pts',(-4.85068927007173,-145.354517970998,
8.40164026752836));
#35937=CARTESIAN_POINT('Ctrl Pts',(1.5129078685785E-11,-145.179517970998,
8.40164026751963));
#35938=CARTESIAN_POINT('Ctrl Pts',(4.85068927010198,-145.004517970998,8.4016402675109));
#35939=CARTESIAN_POINT('Ctrl Pts',(7.27603390513785,-144.829517970998,4.20082013374672));
#35940=CARTESIAN_POINT('Ctrl Pts',(9.70137854017372,-144.654517970998,-1.74689612655491E-11));
#35941=CARTESIAN_POINT('Ctrl Pts',(7.27603390512273,-144.479517970998,-4.20082013377291));
#35942=CARTESIAN_POINT('Ctrl Pts',(4.85068927007173,-144.304517970998,-8.40164026752836));
#35943=CARTESIAN_POINT('Ctrl Pts',(-1.51301075899711E-11,-144.129517970998,
-8.40164026751963));
#35944=CARTESIAN_POINT('Ctrl Pts',(-4.85068927010199,-143.954517970998,
-8.4016402675109));
#35945=CARTESIAN_POINT('Ctrl Pts',(-7.27603390513785,-143.779517970998,
-4.20082013374671));
#35946=CARTESIAN_POINT('Ctrl Pts',(-9.70137854017372,-143.604517970998,
1.74701493417668E-11));
#35947=CARTESIAN_POINT('Ctrl Pts',(-7.27603390512272,-143.429517970998,
4.20082013377292));
#35948=CARTESIAN_POINT('Ctrl Pts',(-4.85068927007173,-143.254517970998,
8.40164026752836));
#35949=CARTESIAN_POINT('Ctrl Pts',(1.5129078685785E-11,-143.079517970998,
8.40164026751963));
#35950=CARTESIAN_POINT('Ctrl Pts',(4.85068927010198,-142.904517970998,8.4016402675109));
#35951=CARTESIAN_POINT('Ctrl Pts',(7.27603390513785,-142.729517970998,4.20082013374672));
#35952=CARTESIAN_POINT('Ctrl Pts',(9.70137854017372,-142.554517970998,-1.74689612655491E-11));
#35953=CARTESIAN_POINT('Ctrl Pts',(7.27603390512273,-142.379517970998,-4.20082013377291));
#35954=CARTESIAN_POINT('Ctrl Pts',(4.85068927007173,-142.204517970998,-8.40164026752836));
#35955=CARTESIAN_POINT('Ctrl Pts',(-1.51301075899711E-11,-142.029517970998,
-8.40164026751963));
#35956=CARTESIAN_POINT('Ctrl Pts',(-4.85068927010199,-141.854517970998,
-8.4016402675109));
#35957=CARTESIAN_POINT('Ctrl Pts',(-7.27603390513785,-141.679517970998,
-4.20082013374671));
#35958=CARTESIAN_POINT('Ctrl Pts',(-9.70137854017372,-141.504517970998,
1.74701493417668E-11));
#35959=CARTESIAN_POINT('Ctrl Pts',(-7.27603390512272,-141.329517970998,
4.20082013377292));
#35960=CARTESIAN_POINT('Ctrl Pts',(-4.85068927007173,-141.154517970998,
8.40164026752836));
#35961=CARTESIAN_POINT('Ctrl Pts',(1.5129078685785E-11,-140.979517970998,
8.40164026751963));
#35962=CARTESIAN_POINT('Ctrl Pts',(4.85068927010198,-140.804517970998,8.4016402675109));
#35963=CARTESIAN_POINT('Ctrl Pts',(7.27603390513785,-140.629517970998,4.20082013374672));
#35964=CARTESIAN_POINT('Ctrl Pts',(9.70137854017372,-140.454517970998,-1.74689612655491E-11));
#35965=CARTESIAN_POINT('Ctrl Pts',(7.27603390512273,-140.279517970998,-4.20082013377291));
#35966=CARTESIAN_POINT('Ctrl Pts',(4.85068927007173,-140.104517970998,-8.40164026752836));
#35967=CARTESIAN_POINT('Ctrl Pts',(-1.51301075899711E-11,-139.929517970998,
-8.40164026751963));
#35968=CARTESIAN_POINT('Ctrl Pts',(-4.85068927010199,-139.754517970998,
-8.4016402675109));
#35969=CARTESIAN_POINT('Ctrl Pts',(-7.27603390513785,-139.579517970998,
-4.20082013374671));
#35970=CARTESIAN_POINT('Ctrl Pts',(-9.70137854017372,-139.404517970998,
1.74701493417668E-11));
#35971=CARTESIAN_POINT('Ctrl Pts',(-7.27603390512272,-139.229517970998,
4.20082013377292));
#35972=CARTESIAN_POINT('Ctrl Pts',(-4.85068927007173,-139.054517970998,
8.40164026752836));
#35973=CARTESIAN_POINT('Ctrl Pts',(1.5129078685785E-11,-138.879517970998,
8.40164026751963));
#35974=CARTESIAN_POINT('Ctrl Pts',(4.85068927010198,-138.704517970998,8.4016402675109));
#35975=CARTESIAN_POINT('Ctrl Pts',(7.27603390513785,-138.529517970998,4.20082013374672));
#35976=CARTESIAN_POINT('Ctrl Pts',(9.70137854017372,-138.354517970998,-1.74689612655491E-11));
#35977=CARTESIAN_POINT('Ctrl Pts',(7.27603390512273,-138.179517970998,-4.20082013377291));
#35978=CARTESIAN_POINT('Ctrl Pts',(4.85068927007173,-138.004517970998,-8.40164026752836));
#35979=CARTESIAN_POINT('Ctrl Pts',(-1.51301075899711E-11,-137.829517970998,
-8.40164026751963));
#35980=CARTESIAN_POINT('Ctrl Pts',(-4.85068927010199,-137.654517970998,
-8.4016402675109));
#35981=CARTESIAN_POINT('Ctrl Pts',(-7.27603390513785,-137.479517970998,
-4.20082013374671));
#35982=CARTESIAN_POINT('Ctrl Pts',(-9.70137854017372,-137.304517970998,
1.74701493417668E-11));
#35983=CARTESIAN_POINT('Ctrl Pts',(-7.27603390512272,-137.129517970998,
4.20082013377292));
#35984=CARTESIAN_POINT('Ctrl Pts',(-4.85068927007173,-136.954517970998,
8.40164026752836));
#35985=CARTESIAN_POINT('Ctrl Pts',(1.5129078685785E-11,-136.779517970998,
8.40164026751963));
#35986=CARTESIAN_POINT('Ctrl Pts',(4.85068927010198,-136.604517970998,8.4016402675109));
#35987=CARTESIAN_POINT('Ctrl Pts',(7.27603390513785,-136.429517970998,4.20082013374672));
#35988=CARTESIAN_POINT('Ctrl Pts',(9.70137854017372,-136.254517970999,-1.74689612655491E-11));
#35989=CARTESIAN_POINT('Ctrl Pts',(7.27603390512273,-136.079517970998,-4.20082013377291));
#35990=CARTESIAN_POINT('Ctrl Pts',(4.85068927007173,-135.904517970998,-8.40164026752836));
#35991=CARTESIAN_POINT('Ctrl Pts',(-1.51301075899711E-11,-135.729517970998,
-8.40164026751963));
#35992=CARTESIAN_POINT('Ctrl Pts',(-4.85068927010199,-135.554517970998,
-8.4016402675109));
#35993=CARTESIAN_POINT('Ctrl Pts',(-7.27603390513785,-135.379517970998,
-4.20082013374671));
#35994=CARTESIAN_POINT('Ctrl Pts',(-9.70137854017372,-135.204517970998,
1.74701493417668E-11));
#35995=CARTESIAN_POINT('Ctrl Pts',(-7.27603390512272,-135.029517970998,
4.20082013377292));
#35996=CARTESIAN_POINT('Ctrl Pts',(-4.85068927007173,-134.854517970998,
8.40164026752836));
#35997=CARTESIAN_POINT('Ctrl Pts',(1.5129078685785E-11,-134.679517970998,
8.40164026751963));
#35998=CARTESIAN_POINT('Ctrl Pts',(4.85068927010198,-134.504517970998,8.4016402675109));
#35999=CARTESIAN_POINT('Ctrl Pts',(7.27603390513785,-134.329517970998,4.20082013374672));
#36000=CARTESIAN_POINT('Ctrl Pts',(9.70137854017372,-134.154517970998,-1.74689612655491E-11));
#36001=CARTESIAN_POINT('Ctrl Pts',(7.27603390512273,-133.979517970998,-4.20082013377291));
#36002=CARTESIAN_POINT('Ctrl Pts',(4.85068927007173,-133.804517970998,-8.40164026752836));
#36003=CARTESIAN_POINT('Ctrl Pts',(-1.51301075899711E-11,-133.629517970998,
-8.40164026751963));
#36004=CARTESIAN_POINT('Ctrl Pts',(-4.85068927010199,-133.454517970998,
-8.4016402675109));
#36005=CARTESIAN_POINT('Ctrl Pts',(-7.27603390513785,-133.279517970998,
-4.20082013374671));
#36006=CARTESIAN_POINT('Ctrl Pts',(-9.70137854017372,-133.104517970998,
1.74701493417668E-11));
#36007=CARTESIAN_POINT('Ctrl Pts',(-7.27603390512272,-132.929517970998,
4.20082013377292));
#36008=CARTESIAN_POINT('Ctrl Pts',(-4.85068927007173,-132.754517970998,
8.40164026752836));
#36009=CARTESIAN_POINT('Ctrl Pts',(1.5129078685785E-11,-132.579517970998,
8.40164026751963));
#36010=CARTESIAN_POINT('Ctrl Pts',(4.85068927010198,-132.404517970998,8.4016402675109));
#36011=CARTESIAN_POINT('Ctrl Pts',(7.27603390513785,-132.229517970998,4.20082013374672));
#36012=CARTESIAN_POINT('Ctrl Pts',(9.70137854017372,-132.054517970998,-1.74689612655491E-11));
#36013=CARTESIAN_POINT('Ctrl Pts',(7.27603390512273,-131.879517970998,-4.20082013377291));
#36014=CARTESIAN_POINT('Ctrl Pts',(4.85068927007173,-131.704517970998,-8.40164026752836));
#36015=CARTESIAN_POINT('Ctrl Pts',(-1.51301075899711E-11,-131.529517970998,
-8.40164026751963));
#36016=CARTESIAN_POINT('Ctrl Pts',(-4.85068927010199,-131.354517970998,
-8.4016402675109));
#36017=CARTESIAN_POINT('Ctrl Pts',(-7.27603390513785,-131.179517970998,
-4.20082013374671));
#36018=CARTESIAN_POINT('Ctrl Pts',(-9.70137854017372,-131.004517970998,
1.74701493417668E-11));
#36019=CARTESIAN_POINT('Ctrl Pts',(-7.27603390512272,-130.829517970998,
4.20082013377292));
#36020=CARTESIAN_POINT('Ctrl Pts',(-4.85068927007173,-130.654517970998,
8.40164026752836));
#36021=CARTESIAN_POINT('Ctrl Pts',(1.5129078685785E-11,-130.479517970998,
8.40164026751963));
#36022=CARTESIAN_POINT('Ctrl Pts',(4.85068927010198,-130.304517970998,8.4016402675109));
#36023=CARTESIAN_POINT('Ctrl Pts',(7.27603390513785,-130.129517970998,4.20082013374672));
#36024=CARTESIAN_POINT('Ctrl Pts',(9.70137854017372,-129.954517970998,-1.74689612655491E-11));
#36025=CARTESIAN_POINT('Ctrl Pts',(7.27603390512273,-129.779517970998,-4.20082013377291));
#36026=CARTESIAN_POINT('Ctrl Pts',(4.85068927007173,-129.604517970998,-8.40164026752836));
#36027=CARTESIAN_POINT('Ctrl Pts',(-1.51301075899711E-11,-129.429517970998,
-8.40164026751963));
#36028=CARTESIAN_POINT('Ctrl Pts',(-4.85068927010199,-129.254517970998,
-8.4016402675109));
#36029=CARTESIAN_POINT('Ctrl Pts',(-7.27603390513785,-129.079517970998,
-4.20082013374671));
#36030=CARTESIAN_POINT('Ctrl Pts',(-9.70137854017372,-128.904517970998,
1.74701493417668E-11));
#36031=CARTESIAN_POINT('Ctrl Pts',(-7.27603390512272,-128.729517970998,
4.20082013377292));
#36032=CARTESIAN_POINT('Ctrl Pts',(-4.85068927007173,-128.554517970998,
8.40164026752836));
#36033=CARTESIAN_POINT('Ctrl Pts',(1.5129078685785E-11,-128.379517970998,
8.40164026751963));
#36034=CARTESIAN_POINT('Ctrl Pts',(4.85068927010198,-128.204517970998,8.4016402675109));
#36035=CARTESIAN_POINT('Ctrl Pts',(7.27603390513785,-128.029517970998,4.20082013374672));
#36036=CARTESIAN_POINT('Ctrl Pts',(9.70137854017372,-127.854517970998,-1.74689612655491E-11));
#36037=CARTESIAN_POINT('Ctrl Pts',(7.27603390512273,-127.679517970998,-4.20082013377291));
#36038=CARTESIAN_POINT('Ctrl Pts',(4.85068927007173,-127.504517970998,-8.40164026752836));
#36039=CARTESIAN_POINT('Ctrl Pts',(-1.51301075899711E-11,-127.329517970998,
-8.40164026751963));
#36040=CARTESIAN_POINT('Ctrl Pts',(-4.85068927010199,-127.154517970998,
-8.4016402675109));
#36041=CARTESIAN_POINT('Ctrl Pts',(-7.27603390513785,-126.979517970998,
-4.20082013374671));
#36042=CARTESIAN_POINT('Ctrl Pts',(-9.70137854017372,-126.804517970998,
1.74701493417668E-11));
#36043=CARTESIAN_POINT('Ctrl Pts',(-7.27603390512272,-126.629517970998,
4.20082013377292));
#36044=CARTESIAN_POINT('Ctrl Pts',(-4.85068927007173,-126.454517970998,
8.40164026752836));
#36045=CARTESIAN_POINT('Ctrl Pts',(1.5129078685785E-11,-126.279517970998,
8.40164026751963));
#36046=CARTESIAN_POINT('Ctrl Pts',(4.85068927010198,-126.104517970998,8.4016402675109));
#36047=CARTESIAN_POINT('Ctrl Pts',(7.27603390513785,-125.929517970998,4.20082013374672));
#36048=CARTESIAN_POINT('Ctrl Pts',(9.70137854017372,-125.754517970998,-1.74689612655491E-11));
#36049=CARTESIAN_POINT('Ctrl Pts',(7.27603390512273,-125.579517970998,-4.20082013377291));
#36050=CARTESIAN_POINT('Ctrl Pts',(4.85068927007173,-125.404517970998,-8.40164026752836));
#36051=CARTESIAN_POINT('Ctrl Pts',(-1.51301075899711E-11,-125.229517970998,
-8.40164026751963));
#36052=CARTESIAN_POINT('Ctrl Pts',(-4.85068927010199,-125.054517970998,
-8.4016402675109));
#36053=CARTESIAN_POINT('Ctrl Pts',(-7.27603390513785,-124.879517970998,
-4.20082013374671));
#36054=CARTESIAN_POINT('Ctrl Pts',(-9.70137854017372,-124.704517970998,
1.74701493417668E-11));
#36055=CARTESIAN_POINT('Ctrl Pts',(-7.27603390512272,-124.529517970998,
4.20082013377292));
#36056=CARTESIAN_POINT('Ctrl Pts',(-4.85068927007173,-124.354517970998,
8.40164026752836));
#36057=CARTESIAN_POINT('Ctrl Pts',(1.5129078685785E-11,-124.179517970998,
8.40164026751963));
#36058=CARTESIAN_POINT('Ctrl Pts',(4.85068927010198,-124.004517970998,8.4016402675109));
#36059=CARTESIAN_POINT('Ctrl Pts',(7.27603390513785,-123.829517970998,4.20082013374672));
#36060=CARTESIAN_POINT('Ctrl Pts',(9.70137854017372,-123.654517970998,-1.74689612655491E-11));
#36061=CARTESIAN_POINT('Ctrl Pts',(7.27603390512273,-123.479517970998,-4.20082013377291));
#36062=CARTESIAN_POINT('Ctrl Pts',(4.85068927007173,-123.304517970998,-8.40164026752836));
#36063=CARTESIAN_POINT('Ctrl Pts',(-1.51301075899711E-11,-123.129517970998,
-8.40164026751963));
#36064=CARTESIAN_POINT('Ctrl Pts',(-4.85068927010199,-122.954517970998,
-8.4016402675109));
#36065=CARTESIAN_POINT('Ctrl Pts',(-7.27603390513785,-122.779517970998,
-4.20082013374671));
#36066=CARTESIAN_POINT('Ctrl Pts',(-9.70137854017372,-122.604517970998,
1.74701493417668E-11));
#36067=CARTESIAN_POINT('Ctrl Pts',(-7.27603390512272,-122.429517970998,
4.20082013377292));
#36068=CARTESIAN_POINT('Ctrl Pts',(-4.85068927007173,-122.254517970998,
8.40164026752836));
#36069=CARTESIAN_POINT('Ctrl Pts',(1.5129078685785E-11,-122.079517970998,
8.40164026751963));
#36070=CARTESIAN_POINT('Ctrl Pts',(4.85068927010198,-121.904517970998,8.4016402675109));
#36071=CARTESIAN_POINT('Ctrl Pts',(7.27603390513785,-121.729517970998,4.20082013374672));
#36072=CARTESIAN_POINT('Ctrl Pts',(9.70137854017372,-121.554517970999,-1.74689612655491E-11));
#36073=CARTESIAN_POINT('Ctrl Pts',(7.27603390512273,-121.379517970998,-4.20082013377291));
#36074=CARTESIAN_POINT('Ctrl Pts',(4.85068927007173,-121.204517970998,-8.40164026752836));
#36075=CARTESIAN_POINT('Ctrl Pts',(-1.51301075899711E-11,-121.029517970998,
-8.40164026751963));
#36076=CARTESIAN_POINT('Ctrl Pts',(-4.85068927010199,-120.854517970999,
-8.4016402675109));
#36077=CARTESIAN_POINT('Ctrl Pts',(-7.27603390513785,-120.679517970999,
-4.20082013374671));
#36078=CARTESIAN_POINT('Ctrl Pts',(-9.70137854017372,-120.504517970999,
1.74701493417668E-11));
#36079=CARTESIAN_POINT('Ctrl Pts',(-7.27603390512272,-120.329517970998,
4.20082013377292));
#36080=CARTESIAN_POINT('Ctrl Pts',(-4.85068927007173,-120.154517970998,
8.40164026752836));
#36081=CARTESIAN_POINT('Ctrl Pts',(1.5129078685785E-11,-119.979517970999,
8.40164026751963));
#36082=CARTESIAN_POINT('Ctrl Pts',(4.85068927010198,-119.804517970999,8.4016402675109));
#36083=CARTESIAN_POINT('Ctrl Pts',(7.27603390513785,-119.629517970998,4.20082013374672));
#36084=CARTESIAN_POINT('Ctrl Pts',(9.70137854017372,-119.454517970998,-1.74689612655491E-11));
#36085=CARTESIAN_POINT('Ctrl Pts',(7.27603390512273,-119.279517970999,-4.20082013377291));
#36086=CARTESIAN_POINT('Ctrl Pts',(4.85068927007173,-119.104517970998,-8.40164026752836));
#36087=CARTESIAN_POINT('Ctrl Pts',(-1.51301075899711E-11,-118.929517970998,
-8.40164026751963));
#36088=CARTESIAN_POINT('Ctrl Pts',(-4.85068927010199,-118.754517970998,
-8.4016402675109));
#36089=CARTESIAN_POINT('Ctrl Pts',(-7.27603390513785,-118.579517970998,
-4.20082013374671));
#36090=CARTESIAN_POINT('Ctrl Pts',(-9.70137854017372,-118.404517970999,
1.74701493417668E-11));
#36091=CARTESIAN_POINT('Ctrl Pts',(-7.27603390512272,-118.229517970998,
4.20082013377292));
#36092=CARTESIAN_POINT('Ctrl Pts',(-4.85068927007173,-118.054517970998,
8.40164026752836));
#36093=CARTESIAN_POINT('Ctrl Pts',(1.5129078685785E-11,-117.879517970999,
8.40164026751963));
#36094=CARTESIAN_POINT('Ctrl Pts',(4.85068927010198,-117.704517970998,8.4016402675109));
#36095=CARTESIAN_POINT('Ctrl Pts',(7.27603390513785,-117.529517970998,4.20082013374672));
#36096=CARTESIAN_POINT('Ctrl Pts',(9.70137854017372,-117.354517970999,-1.74689612655491E-11));
#36097=CARTESIAN_POINT('Ctrl Pts',(7.27603390512273,-117.179517970999,-4.20082013377291));
#36098=CARTESIAN_POINT('Ctrl Pts',(4.85068927007173,-117.004517970999,-8.40164026752836));
#36099=CARTESIAN_POINT('Ctrl Pts',(-1.51301075899711E-11,-116.829517970998,
-8.40164026751963));
#36100=CARTESIAN_POINT('Ctrl Pts',(-4.85068927010199,-116.654517970998,
-8.4016402675109));
#36101=CARTESIAN_POINT('Ctrl Pts',(-7.27603390513785,-116.479517970999,
-4.20082013374671));
#36102=CARTESIAN_POINT('Ctrl Pts',(-9.70137854017372,-116.304517970999,
1.74701493417668E-11));
#36103=CARTESIAN_POINT('Ctrl Pts',(-7.27603390512272,-116.129517970999,
4.20082013377292));
#36104=CARTESIAN_POINT('Ctrl Pts',(-4.85068927007173,-115.954517970998,
8.40164026752836));
#36105=CARTESIAN_POINT('Ctrl Pts',(1.5129078685785E-11,-115.779517970998,
8.40164026751963));
#36106=CARTESIAN_POINT('Ctrl Pts',(4.85068927010198,-115.604517970999,8.4016402675109));
#36107=CARTESIAN_POINT('Ctrl Pts',(7.27603390513785,-115.429517970999,4.20082013374672));
#36108=CARTESIAN_POINT('Ctrl Pts',(9.70137854017372,-115.254517970999,-1.74689612655491E-11));
#36109=CARTESIAN_POINT('Ctrl Pts',(7.27603390512273,-115.079517970998,-4.20082013377291));
#36110=CARTESIAN_POINT('Ctrl Pts',(4.85068927007173,-114.904517970999,-8.40164026752836));
#36111=CARTESIAN_POINT('Ctrl Pts',(-1.51301075899711E-11,-114.729517970999,
-8.40164026751963));
#36112=CARTESIAN_POINT('Ctrl Pts',(-4.85068927010199,-114.554517970999,
-8.4016402675109));
#36113=CARTESIAN_POINT('Ctrl Pts',(-7.27603390513785,-114.379517970999,
-4.20082013374671));
#36114=CARTESIAN_POINT('Ctrl Pts',(-9.70137854017372,-114.204517970999,
1.74701493417668E-11));
#36115=CARTESIAN_POINT('Ctrl Pts',(-7.27603390512272,-114.029517970999,
4.20082013377292));
#36116=CARTESIAN_POINT('Ctrl Pts',(-4.85068927007173,-113.854517970999,
8.40164026752836));
#36117=CARTESIAN_POINT('Ctrl Pts',(1.5129078685785E-11,-113.679517970999,
8.40164026751963));
#36118=CARTESIAN_POINT('Ctrl Pts',(4.85068927010198,-113.504517970999,8.4016402675109));
#36119=CARTESIAN_POINT('Ctrl Pts',(7.27603390513785,-113.329517970999,4.20082013374672));
#36120=CARTESIAN_POINT('Ctrl Pts',(9.70137854017372,-113.154517970999,-1.74689612655491E-11));
#36121=CARTESIAN_POINT('Ctrl Pts',(7.27603390512273,-112.979517970999,-4.20082013377291));
#36122=CARTESIAN_POINT('Ctrl Pts',(4.85068927007173,-112.804517970999,-8.40164026752836));
#36123=CARTESIAN_POINT('Ctrl Pts',(-1.51301075899711E-11,-112.629517970999,
-8.40164026751963));
#36124=CARTESIAN_POINT('Ctrl Pts',(-4.85068927010199,-112.454517970998,
-8.4016402675109));
#36125=CARTESIAN_POINT('Ctrl Pts',(-7.27603390513785,-112.279517970998,
-4.20082013374671));
#36126=CARTESIAN_POINT('Ctrl Pts',(-9.70137854017372,-112.104517970999,
1.74701493417668E-11));
#36127=CARTESIAN_POINT('Ctrl Pts',(-7.27603390512272,-111.929517970999,
4.20082013377292));
#36128=CARTESIAN_POINT('Ctrl Pts',(-4.85068927007173,-111.754517970999,
8.40164026752836));
#36129=CARTESIAN_POINT('Ctrl Pts',(1.5129078685785E-11,-111.579517970999,
8.40164026751963));
#36130=CARTESIAN_POINT('Ctrl Pts',(4.85068927010198,-111.404517970998,8.4016402675109));
#36131=CARTESIAN_POINT('Ctrl Pts',(7.27603390513785,-111.229517970999,4.20082013374672));
#36132=CARTESIAN_POINT('Ctrl Pts',(9.70137854017372,-111.054517970999,-1.74689612655491E-11));
#36133=CARTESIAN_POINT('Ctrl Pts',(7.27603390512273,-110.879517970999,-4.20082013377291));
#36134=CARTESIAN_POINT('Ctrl Pts',(4.85068927007173,-110.704517970999,-8.40164026752836));
#36135=CARTESIAN_POINT('Ctrl Pts',(-1.51301075899711E-11,-110.529517970999,
-8.40164026751963));
#36136=CARTESIAN_POINT('Ctrl Pts',(-4.85068927010199,-110.354517970999,
-8.4016402675109));
#36137=CARTESIAN_POINT('Ctrl Pts',(-7.27603390513785,-110.179517970999,
-4.20082013374671));
#36138=CARTESIAN_POINT('Ctrl Pts',(-9.70137854017372,-110.004517970999,
1.74701493417668E-11));
#36139=CARTESIAN_POINT('Ctrl Pts',(-7.27603390512272,-109.829517970999,
4.20082013377292));
#36140=CARTESIAN_POINT('Ctrl Pts',(-4.85068927007173,-109.654517970999,
8.40164026752836));
#36141=CARTESIAN_POINT('Ctrl Pts',(1.5129078685785E-11,-109.479517970999,
8.40164026751963));
#36142=CARTESIAN_POINT('Ctrl Pts',(4.85068927010198,-109.304517970999,8.4016402675109));
#36143=CARTESIAN_POINT('Ctrl Pts',(7.27603390513785,-109.129517970999,4.20082013374672));
#36144=CARTESIAN_POINT('Ctrl Pts',(9.70137854017372,-108.954517970999,-1.74689612655491E-11));
#36145=CARTESIAN_POINT('Ctrl Pts',(7.27603390512273,-108.779517970999,-4.20082013377291));
#36146=CARTESIAN_POINT('Ctrl Pts',(4.85068927007173,-108.604517970999,-8.40164026752836));
#36147=CARTESIAN_POINT('Ctrl Pts',(-1.51301075899711E-11,-108.429517970999,
-8.40164026751963));
#36148=CARTESIAN_POINT('Ctrl Pts',(-4.85068927010199,-108.254517970999,
-8.4016402675109));
#36149=CARTESIAN_POINT('Ctrl Pts',(-7.27603390513785,-108.079517970999,
-4.20082013374671));
#36150=CARTESIAN_POINT('Ctrl Pts',(-9.70137854017372,-107.904517970999,
1.74701493417668E-11));
#36151=CARTESIAN_POINT('Ctrl Pts',(-7.27603390512272,-107.729517970999,
4.20082013377292));
#36152=CARTESIAN_POINT('Ctrl Pts',(-4.85068927007173,-107.554517970999,
8.40164026752836));
#36153=CARTESIAN_POINT('Ctrl Pts',(1.5129078685785E-11,-107.379517970999,
8.40164026751963));
#36154=CARTESIAN_POINT('Ctrl Pts',(4.85068927010198,-107.204517970999,8.4016402675109));
#36155=CARTESIAN_POINT('Ctrl Pts',(7.27603390513785,-107.029517970999,4.20082013374672));
#36156=CARTESIAN_POINT('Ctrl Pts',(9.70137854017372,-106.854517970999,-1.74689612655491E-11));
#36157=CARTESIAN_POINT('Ctrl Pts',(7.27603390512273,-106.679517970999,-4.20082013377291));
#36158=CARTESIAN_POINT('Ctrl Pts',(4.85068927007173,-106.504517970998,-8.40164026752836));
#36159=CARTESIAN_POINT('Ctrl Pts',(-1.51301075899711E-11,-106.329517970999,
-8.40164026751963));
#36160=CARTESIAN_POINT('Ctrl Pts',(-4.85068927010199,-106.154517970999,
-8.4016402675109));
#36161=CARTESIAN_POINT('Ctrl Pts',(-7.27603390513785,-105.979517970999,
-4.20082013374671));
#36162=CARTESIAN_POINT('Ctrl Pts',(-9.70137854017372,-105.804517970999,
1.74701493417668E-11));
#36163=CARTESIAN_POINT('Ctrl Pts',(-7.27603390512272,-105.629517970999,
4.20082013377292));
#36164=CARTESIAN_POINT('Ctrl Pts',(-4.85068927007173,-105.454517970999,
8.40164026752836));
#36165=CARTESIAN_POINT('Ctrl Pts',(1.5129078685785E-11,-105.279517970999,
8.40164026751963));
#36166=CARTESIAN_POINT('Ctrl Pts',(4.85068927010198,-105.104517970999,8.4016402675109));
#36167=CARTESIAN_POINT('Ctrl Pts',(7.27603390513785,-104.929517970999,4.20082013374672));
#36168=CARTESIAN_POINT('Ctrl Pts',(9.70137854017372,-104.754517970999,-1.74689612655491E-11));
#36169=CARTESIAN_POINT('Ctrl Pts',(7.27603390512273,-104.579517970999,-4.20082013377291));
#36170=CARTESIAN_POINT('Ctrl Pts',(4.85068927007173,-104.404517970999,-8.40164026752836));
#36171=CARTESIAN_POINT('Ctrl Pts',(-1.51301075899711E-11,-104.229517970999,
-8.40164026751963));
#36172=CARTESIAN_POINT('Ctrl Pts',(-4.85068927010199,-104.054517970999,
-8.4016402675109));
#36173=CARTESIAN_POINT('Ctrl Pts',(-7.27603390513785,-103.879517970999,
-4.20082013374671));
#36174=CARTESIAN_POINT('Ctrl Pts',(-9.70137854017372,-103.704517970999,
1.74701493417668E-11));
#36175=CARTESIAN_POINT('Ctrl Pts',(-7.27603390512272,-103.529517970999,
4.20082013377292));
#36176=CARTESIAN_POINT('Ctrl Pts',(-4.85068927007173,-103.354517970999,
8.40164026752836));
#36177=CARTESIAN_POINT('Ctrl Pts',(1.5129078685785E-11,-103.179517970999,
8.40164026751963));
#36178=CARTESIAN_POINT('Ctrl Pts',(4.85068927010198,-103.004517970999,8.4016402675109));
#36179=CARTESIAN_POINT('Ctrl Pts',(7.27603390513785,-102.829517970999,4.20082013374672));
#36180=CARTESIAN_POINT('Ctrl Pts',(9.70137854017372,-102.654517970999,-1.74689612655491E-11));
#36181=CARTESIAN_POINT('Ctrl Pts',(7.27603390512273,-102.479517970999,-4.20082013377291));
#36182=CARTESIAN_POINT('Ctrl Pts',(4.85068927007173,-102.304517970999,-8.40164026752836));
#36183=CARTESIAN_POINT('Ctrl Pts',(-1.51301075899711E-11,-102.129517970999,
-8.40164026751963));
#36184=CARTESIAN_POINT('Ctrl Pts',(-4.85068927010199,-101.954517970999,
-8.4016402675109));
#36185=CARTESIAN_POINT('Ctrl Pts',(-7.27603390513785,-101.779517970999,
-4.20082013374671));
#36186=CARTESIAN_POINT('Ctrl Pts',(-9.70137854017372,-101.604517970999,
1.74701493417668E-11));
#36187=CARTESIAN_POINT('Ctrl Pts',(-7.27603390512272,-101.429517970999,
4.20082013377292));
#36188=CARTESIAN_POINT('Ctrl Pts',(-4.85068927007173,-101.254517970999,
8.40164026752836));
#36189=CARTESIAN_POINT('Ctrl Pts',(1.5129078685785E-11,-101.079517970999,
8.40164026751963));
#36190=CARTESIAN_POINT('Ctrl Pts',(4.85068927010198,-100.904517970999,8.4016402675109));
#36191=CARTESIAN_POINT('Ctrl Pts',(7.27603390513785,-100.729517970999,4.20082013374672));
#36192=CARTESIAN_POINT('Ctrl Pts',(9.70137854017372,-100.554517970999,-1.74689612655491E-11));
#36193=CARTESIAN_POINT('Ctrl Pts',(7.27603390512273,-100.379517970999,-4.20082013377291));
#36194=CARTESIAN_POINT('Ctrl Pts',(4.85068927007173,-100.204517970999,-8.40164026752836));
#36195=CARTESIAN_POINT('Ctrl Pts',(-1.51301075899711E-11,-100.029517970999,
-8.40164026751963));
#36196=CARTESIAN_POINT('Ctrl Pts',(-4.85068927010199,-99.8545179709986,
-8.4016402675109));
#36197=CARTESIAN_POINT('Ctrl Pts',(-7.27603390513785,-99.6795179709985,
-4.20082013374671));
#36198=CARTESIAN_POINT('Ctrl Pts',(-9.70137854017372,-99.5045179709985,
1.74701493417668E-11));
#36199=CARTESIAN_POINT('Ctrl Pts',(-7.27603390512272,-99.3295179709985,
4.20082013377292));
#36200=CARTESIAN_POINT('Ctrl Pts',(-4.85068927007173,-99.1545179709985,
8.40164026752836));
#36201=CARTESIAN_POINT('Ctrl Pts',(1.5129078685785E-11,-98.9795179709985,
8.40164026751963));
#36202=CARTESIAN_POINT('Ctrl Pts',(4.85068927010198,-98.8045179709985,8.4016402675109));
#36203=CARTESIAN_POINT('Ctrl Pts',(7.27603390513785,-98.6295179709985,4.20082013374672));
#36204=CARTESIAN_POINT('Ctrl Pts',(9.70137854017372,-98.4545179709986,-1.74689612655491E-11));
#36205=CARTESIAN_POINT('Ctrl Pts',(7.27603390512273,-98.2795179709986,-4.20082013377291));
#36206=CARTESIAN_POINT('Ctrl Pts',(4.85068927007173,-98.1045179709986,-8.40164026752836));
#36207=CARTESIAN_POINT('Ctrl Pts',(-1.51301075899711E-11,-97.9295179709985,
-8.40164026751963));
#36208=CARTESIAN_POINT('Ctrl Pts',(-4.85068927010199,-97.7545179709985,
-8.4016402675109));
#36209=CARTESIAN_POINT('Ctrl Pts',(-7.27603390513785,-97.5795179709986,
-4.20082013374671));
#36210=CARTESIAN_POINT('Ctrl Pts',(-9.70137854017372,-97.4045179709985,
1.74701493417668E-11));
#36211=CARTESIAN_POINT('Ctrl Pts',(-7.27603390512272,-97.2295179709985,
4.20082013377292));
#36212=CARTESIAN_POINT('Ctrl Pts',(-4.85068927007173,-97.0545179709985,
8.40164026752836));
#36213=CARTESIAN_POINT('Ctrl Pts',(1.5129078685785E-11,-96.8795179709986,
8.40164026751963));
#36214=CARTESIAN_POINT('Ctrl Pts',(4.85068927010198,-96.7045179709986,8.4016402675109));
#36215=CARTESIAN_POINT('Ctrl Pts',(7.27603390513785,-96.5295179709985,4.20082013374672));
#36216=CARTESIAN_POINT('Ctrl Pts',(9.70137854017372,-96.3545179709985,-1.74689612655491E-11));
#36217=CARTESIAN_POINT('Ctrl Pts',(7.27603390512273,-96.1795179709985,-4.20082013377291));
#36218=CARTESIAN_POINT('Ctrl Pts',(4.85068927007173,-96.0045179709986,-8.40164026752836));
#36219=CARTESIAN_POINT('Ctrl Pts',(-1.51301075899711E-11,-95.8295179709985,
-8.40164026751963));
#36220=CARTESIAN_POINT('Ctrl Pts',(-4.85068927010199,-95.6545179709985,
-8.4016402675109));
#36221=CARTESIAN_POINT('Ctrl Pts',(-7.27603390513785,-95.4795179709985,
-4.20082013374671));
#36222=CARTESIAN_POINT('Ctrl Pts',(-9.70137854017372,-95.3045179709986,
1.74701493417668E-11));
#36223=CARTESIAN_POINT('Ctrl Pts',(-7.27603390512272,-95.1295179709986,
4.20082013377292));
#36224=CARTESIAN_POINT('Ctrl Pts',(-4.85068927007173,-94.9545179709986,
8.40164026752836));
#36225=CARTESIAN_POINT('Ctrl Pts',(1.5129078685785E-11,-94.7795179709985,
8.40164026751963));
#36226=CARTESIAN_POINT('Ctrl Pts',(4.85068927010198,-94.6045179709986,8.4016402675109));
#36227=CARTESIAN_POINT('Ctrl Pts',(7.27603390513785,-94.4295179709985,4.20082013374672));
#36228=CARTESIAN_POINT('Ctrl Pts',(9.70137854017372,-94.2545179709985,-1.74689612655491E-11));
#36229=CARTESIAN_POINT('Ctrl Pts',(7.27603390512273,-94.0795179709986,-4.20082013377291));
#36230=CARTESIAN_POINT('Ctrl Pts',(4.85068927007173,-93.9045179709986,-8.40164026752836));
#36231=CARTESIAN_POINT('Ctrl Pts',(-1.51301075899711E-11,-93.7295179709986,
-8.40164026751963));
#36232=CARTESIAN_POINT('Ctrl Pts',(-4.85068927010199,-93.5545179709985,
-8.4016402675109));
#36233=CARTESIAN_POINT('Ctrl Pts',(-7.27603390513785,-93.3795179709985,
-4.20082013374671));
#36234=CARTESIAN_POINT('Ctrl Pts',(-9.70137854017372,-93.2045179709986,
1.74701493417668E-11));
#36235=CARTESIAN_POINT('Ctrl Pts',(-7.27603390512272,-93.0295179709986,
4.20082013377292));
#36236=CARTESIAN_POINT('Ctrl Pts',(-4.85068927007173,-92.8545179709985,
8.40164026752836));
#36237=CARTESIAN_POINT('Ctrl Pts',(1.5129078685785E-11,-92.6795179709985,
8.40164026751963));
#36238=CARTESIAN_POINT('Ctrl Pts',(4.85068927010198,-92.5045179709985,8.4016402675109));
#36239=CARTESIAN_POINT('Ctrl Pts',(7.27603390513785,-92.3295179709986,4.20082013374672));
#36240=CARTESIAN_POINT('Ctrl Pts',(9.70137854017372,-92.1545179709986,-1.74689612655491E-11));
#36241=CARTESIAN_POINT('Ctrl Pts',(7.27603390512273,-91.9795179709986,-4.20082013377291));
#36242=CARTESIAN_POINT('Ctrl Pts',(4.85068927007173,-91.8045179709985,-8.40164026752836));
#36243=CARTESIAN_POINT('Ctrl Pts',(-1.51301075899711E-11,-91.6295179709986,
-8.40164026751963));
#36244=CARTESIAN_POINT('Ctrl Pts',(-4.85068927010199,-91.4545179709986,
-8.4016402675109));
#36245=CARTESIAN_POINT('Ctrl Pts',(-7.27603390513785,-91.2795179709986,
-4.20082013374671));
#36246=CARTESIAN_POINT('Ctrl Pts',(-9.70137854017372,-91.1045179709985,
1.74701493417668E-11));
#36247=CARTESIAN_POINT('Ctrl Pts',(-7.27603390512272,-90.9295179709986,
4.20082013377292));
#36248=CARTESIAN_POINT('Ctrl Pts',(-4.85068927007173,-90.7545179709986,
8.40164026752836));
#36249=CARTESIAN_POINT('Ctrl Pts',(1.5129078685785E-11,-90.5795179709986,
8.40164026751963));
#36250=CARTESIAN_POINT('Ctrl Pts',(4.85068927010198,-90.4045179709985,8.4016402675109));
#36251=CARTESIAN_POINT('Ctrl Pts',(7.27603390513785,-90.2295179709986,4.20082013374672));
#36252=CARTESIAN_POINT('Ctrl Pts',(9.70137854017372,-90.0545179709986,-1.74689612655491E-11));
#36253=CARTESIAN_POINT('Ctrl Pts',(7.27603390512273,-89.8795179709985,-4.20082013377291));
#36254=CARTESIAN_POINT('Ctrl Pts',(4.85068927007173,-89.7045179709986,-8.40164026752836));
#36255=CARTESIAN_POINT('Ctrl Pts',(-1.51301075899711E-11,-89.5295179709986,
-8.40164026751963));
#36256=CARTESIAN_POINT('Ctrl Pts',(-4.85068927010199,-89.3545179709986,
-8.4016402675109));
#36257=CARTESIAN_POINT('Ctrl Pts',(-7.27603390513785,-89.1795179709986,
-4.20082013374671));
#36258=CARTESIAN_POINT('Ctrl Pts',(-9.70137854017372,-89.0045179709985,
1.74701493417668E-11));
#36259=CARTESIAN_POINT('Ctrl Pts',(-7.27603390512272,-88.8295179709986,
4.20082013377292));
#36260=CARTESIAN_POINT('Ctrl Pts',(-4.85068927007173,-88.6545179709986,
8.40164026752836));
#36261=CARTESIAN_POINT('Ctrl Pts',(1.5129078685785E-11,-88.4795179709986,
8.40164026751963));
#36262=CARTESIAN_POINT('Ctrl Pts',(4.85068927010198,-88.3045179709985,8.4016402675109));
#36263=CARTESIAN_POINT('Ctrl Pts',(7.27603390513785,-88.1295179709985,4.20082013374672));
#36264=CARTESIAN_POINT('Ctrl Pts',(9.70137854017372,-87.9545179709986,-1.74689612655491E-11));
#36265=CARTESIAN_POINT('Ctrl Pts',(7.27603390512273,-87.7795179709986,-4.20082013377291));
#36266=CARTESIAN_POINT('Ctrl Pts',(4.85068927007173,-87.6045179709986,-8.40164026752836));
#36267=CARTESIAN_POINT('Ctrl Pts',(-1.51301075899711E-11,-87.4295179709986,
-8.40164026751963));
#36268=CARTESIAN_POINT('Ctrl Pts',(-4.85068927010199,-87.2545179709986,
-8.4016402675109));
#36269=CARTESIAN_POINT('Ctrl Pts',(-7.27603390513785,-87.0795179709986,
-4.20082013374671));
#36270=CARTESIAN_POINT('Ctrl Pts',(-9.70137854017372,-86.9045179709986,
1.74701493417668E-11));
#36271=CARTESIAN_POINT('Ctrl Pts',(-7.27603390512272,-86.7295179709986,
4.20082013377292));
#36272=CARTESIAN_POINT('Ctrl Pts',(-4.85068927007173,-86.5545179709986,
8.40164026752836));
#36273=CARTESIAN_POINT('Ctrl Pts',(1.5129078685785E-11,-86.3795179709986,
8.40164026751963));
#36274=CARTESIAN_POINT('Ctrl Pts',(4.85068927010198,-86.2045179709986,8.4016402675109));
#36275=CARTESIAN_POINT('Ctrl Pts',(7.27603390513785,-86.0295179709986,4.20082013374672));
#36276=CARTESIAN_POINT('Ctrl Pts',(9.70137854017372,-85.8545179709986,-1.74689612655491E-11));
#36277=CARTESIAN_POINT('Ctrl Pts',(7.27603390512273,-85.6795179709986,-4.20082013377291));
#36278=CARTESIAN_POINT('Ctrl Pts',(4.85068927007173,-85.5045179709986,-8.40164026752836));
#36279=CARTESIAN_POINT('Ctrl Pts',(-1.51301075899711E-11,-85.3295179709986,
-8.40164026751963));
#36280=CARTESIAN_POINT('Ctrl Pts',(-4.85068927010199,-85.1545179709986,
-8.4016402675109));
#36281=CARTESIAN_POINT('Ctrl Pts',(-7.27603390513785,-84.9795179709986,
-4.20082013374671));
#36282=CARTESIAN_POINT('Ctrl Pts',(-9.70137854017372,-84.8045179709986,
1.74701493417668E-11));
#36283=CARTESIAN_POINT('Ctrl Pts',(-7.27603390512272,-84.6295179709986,
4.20082013377292));
#36284=CARTESIAN_POINT('Ctrl Pts',(-4.85068927007173,-84.4545179709986,
8.40164026752836));
#36285=CARTESIAN_POINT('Ctrl Pts',(1.5129078685785E-11,-84.2795179709986,
8.40164026751963));
#36286=CARTESIAN_POINT('Ctrl Pts',(4.85068927010198,-84.1045179709986,8.4016402675109));
#36287=CARTESIAN_POINT('Ctrl Pts',(7.27603390513785,-83.9295179709986,4.20082013374672));
#36288=CARTESIAN_POINT('Ctrl Pts',(9.70137854017372,-83.7545179709985,-1.74689612655491E-11));
#36289=CARTESIAN_POINT('Ctrl Pts',(7.27603390512273,-83.5795179709986,-4.20082013377291));
#36290=CARTESIAN_POINT('Ctrl Pts',(4.85068927007173,-83.4045179709986,-8.40164026752836));
#36291=CARTESIAN_POINT('Ctrl Pts',(-1.51301075899711E-11,-83.2295179709986,
-8.40164026751963));
#36292=CARTESIAN_POINT('Ctrl Pts',(-4.85068927010199,-83.0545179709986,
-8.4016402675109));
#36293=CARTESIAN_POINT('Ctrl Pts',(-7.27603390513785,-82.8795179709986,
-4.20082013374671));
#36294=CARTESIAN_POINT('Ctrl Pts',(-9.70137854017372,-82.7045179709986,
1.74701493417668E-11));
#36295=CARTESIAN_POINT('Ctrl Pts',(-7.27603390512272,-82.5295179709986,
4.20082013377292));
#36296=CARTESIAN_POINT('Ctrl Pts',(-4.85068927007173,-82.3545179709986,
8.40164026752836));
#36297=CARTESIAN_POINT('Ctrl Pts',(1.5129078685785E-11,-82.1795179709986,
8.40164026751963));
#36298=CARTESIAN_POINT('Ctrl Pts',(4.85068927010198,-82.0045179709986,8.4016402675109));
#36299=CARTESIAN_POINT('Ctrl Pts',(7.27603390513785,-81.8295179709986,4.20082013374672));
#36300=CARTESIAN_POINT('Ctrl Pts',(9.70137854017372,-81.6545179709986,-1.74689612655491E-11));
#36301=CARTESIAN_POINT('Ctrl Pts',(7.27603390512273,-81.4795179709986,-4.20082013377291));
#36302=CARTESIAN_POINT('Ctrl Pts',(4.85068927007173,-81.3045179709986,-8.40164026752836));
#36303=CARTESIAN_POINT('Ctrl Pts',(-1.51301075899711E-11,-81.1295179709986,
-8.40164026751963));
#36304=CARTESIAN_POINT('Ctrl Pts',(-4.85068927010199,-80.9545179709986,
-8.4016402675109));
#36305=CARTESIAN_POINT('Ctrl Pts',(-7.27603390513785,-80.7795179709986,
-4.20082013374671));
#36306=CARTESIAN_POINT('Ctrl Pts',(-9.70137854017372,-80.6045179709986,
1.74701493417668E-11));
#36307=CARTESIAN_POINT('Ctrl Pts',(-7.27603390512272,-80.4295179709986,
4.20082013377292));
#36308=CARTESIAN_POINT('Ctrl Pts',(-4.85068927007173,-80.2545179709986,
8.40164026752836));
#36309=CARTESIAN_POINT('Ctrl Pts',(1.5129078685785E-11,-80.0795179709986,
8.40164026751963));
#36310=CARTESIAN_POINT('Ctrl Pts',(4.85068927010198,-79.9045179709986,8.4016402675109));
#36311=CARTESIAN_POINT('Ctrl Pts',(7.27603390513785,-79.7295179709986,4.20082013374672));
#36312=CARTESIAN_POINT('Ctrl Pts',(9.70137854017372,-79.5545179709986,-1.74689612655491E-11));
#36313=CARTESIAN_POINT('Ctrl Pts',(7.27603390512273,-79.3795179709986,-4.20082013377291));
#36314=CARTESIAN_POINT('Ctrl Pts',(4.85068927007173,-79.2045179709986,-8.40164026752836));
#36315=CARTESIAN_POINT('Ctrl Pts',(-1.51301075899711E-11,-79.0295179709986,
-8.40164026751963));
#36316=CARTESIAN_POINT('Ctrl Pts',(-4.85068927010199,-78.8545179709986,
-8.4016402675109));
#36317=CARTESIAN_POINT('Ctrl Pts',(-7.27603390513785,-78.6795179709986,
-4.20082013374671));
#36318=CARTESIAN_POINT('Ctrl Pts',(-9.70137854017372,-78.5045179709986,
1.74701493417668E-11));
#36319=CARTESIAN_POINT('Ctrl Pts',(-7.27603390512272,-78.3295179709986,
4.20082013377292));
#36320=CARTESIAN_POINT('Ctrl Pts',(-4.85068927007173,-78.1545179709986,
8.40164026752836));
#36321=CARTESIAN_POINT('Ctrl Pts',(1.5129078685785E-11,-77.9795179709986,
8.40164026751963));
#36322=CARTESIAN_POINT('Ctrl Pts',(4.85068927010198,-77.8045179709986,8.4016402675109));
#36323=CARTESIAN_POINT('Ctrl Pts',(7.27603390513785,-77.6295179709986,4.20082013374672));
#36324=CARTESIAN_POINT('Ctrl Pts',(9.70137854017372,-77.4545179709986,-1.74689612655491E-11));
#36325=CARTESIAN_POINT('Ctrl Pts',(7.27603390512273,-77.2795179709986,-4.20082013377291));
#36326=CARTESIAN_POINT('Ctrl Pts',(4.85068927007173,-77.1045179709986,-8.40164026752836));
#36327=CARTESIAN_POINT('Ctrl Pts',(-1.51301075899711E-11,-76.9295179709986,
-8.40164026751963));
#36328=CARTESIAN_POINT('Ctrl Pts',(-4.85068927010199,-76.7545179709986,
-8.4016402675109));
#36329=CARTESIAN_POINT('Ctrl Pts',(-7.27603390513785,-76.5795179709986,
-4.20082013374671));
#36330=CARTESIAN_POINT('Ctrl Pts',(-9.70137854017372,-76.4045179709986,
1.74701493417668E-11));
#36331=CARTESIAN_POINT('Ctrl Pts',(-7.27603390512272,-76.2295179709986,
4.20082013377292));
#36332=CARTESIAN_POINT('Ctrl Pts',(-4.85068927007173,-76.0545179709986,
8.40164026752836));
#36333=CARTESIAN_POINT('Ctrl Pts',(1.5129078685785E-11,-75.8795179709986,
8.40164026751963));
#36334=CARTESIAN_POINT('Ctrl Pts',(4.85068927010198,-75.7045179709986,8.4016402675109));
#36335=CARTESIAN_POINT('Ctrl Pts',(7.27603390513785,-75.5295179709986,4.20082013374672));
#36336=CARTESIAN_POINT('Ctrl Pts',(9.70137854017372,-75.3545179709986,-1.74689612655491E-11));
#36337=CARTESIAN_POINT('Ctrl Pts',(7.27603390512273,-75.1795179709986,-4.20082013377291));
#36338=CARTESIAN_POINT('Ctrl Pts',(4.85068927007173,-75.0045179709986,-8.40164026752836));
#36339=CARTESIAN_POINT('Ctrl Pts',(-1.51301075899711E-11,-74.8295179709986,
-8.40164026751963));
#36340=CARTESIAN_POINT('Ctrl Pts',(-4.85068927010199,-74.6545179709986,
-8.4016402675109));
#36341=CARTESIAN_POINT('Ctrl Pts',(-7.27603390513785,-74.4795179709986,
-4.20082013374671));
#36342=CARTESIAN_POINT('Ctrl Pts',(-9.70137854017372,-74.3045179709986,
1.74701493417668E-11));
#36343=CARTESIAN_POINT('Ctrl Pts',(-7.27603390512272,-74.1295179709986,
4.20082013377292));
#36344=CARTESIAN_POINT('Ctrl Pts',(-4.85068927007173,-73.9545179709986,
8.40164026752836));
#36345=CARTESIAN_POINT('Ctrl Pts',(1.5129078685785E-11,-73.7795179709986,
8.40164026751963));
#36346=CARTESIAN_POINT('Ctrl Pts',(4.85068927010198,-73.6045179709986,8.4016402675109));
#36347=CARTESIAN_POINT('Ctrl Pts',(7.27603390513785,-73.4295179709986,4.20082013374672));
#36348=CARTESIAN_POINT('Ctrl Pts',(9.70137854017372,-73.2545179709986,-1.74689612655491E-11));
#36349=CARTESIAN_POINT('Ctrl Pts',(7.27603390512273,-73.0795179709986,-4.20082013377291));
#36350=CARTESIAN_POINT('Ctrl Pts',(4.85068927007173,-72.9045179709986,-8.40164026752836));
#36351=CARTESIAN_POINT('Ctrl Pts',(-1.51301075899711E-11,-72.7295179709986,
-8.40164026751963));
#36352=CARTESIAN_POINT('Ctrl Pts',(-4.85068927010199,-72.5545179709986,
-8.4016402675109));
#36353=CARTESIAN_POINT('Ctrl Pts',(-7.27603390513785,-72.3795179709986,
-4.20082013374671));
#36354=CARTESIAN_POINT('Ctrl Pts',(-9.70137854017372,-72.2045179709986,
1.74701493417668E-11));
#36355=CARTESIAN_POINT('Ctrl Pts',(-7.27603390512272,-72.0295179709986,
4.20082013377292));
#36356=CARTESIAN_POINT('Ctrl Pts',(-4.85068927007173,-71.8545179709986,
8.40164026752836));
#36357=CARTESIAN_POINT('Ctrl Pts',(1.5129078685785E-11,-71.6795179709986,
8.40164026751963));
#36358=CARTESIAN_POINT('Ctrl Pts',(4.85068927010198,-71.5045179709986,8.4016402675109));
#36359=CARTESIAN_POINT('Ctrl Pts',(7.27603390513785,-71.3295179709986,4.20082013374672));
#36360=CARTESIAN_POINT('Ctrl Pts',(9.70137854017372,-71.1545179709986,-1.74689612655491E-11));
#36361=CARTESIAN_POINT('Ctrl Pts',(7.27603390512273,-70.9795179709986,-4.20082013377291));
#36362=CARTESIAN_POINT('Ctrl Pts',(4.85068927007173,-70.8045179709986,-8.40164026752836));
#36363=CARTESIAN_POINT('Ctrl Pts',(-1.51301075899711E-11,-70.6295179709986,
-8.40164026751963));
#36364=CARTESIAN_POINT('Ctrl Pts',(-4.85068927010199,-70.4545179709986,
-8.4016402675109));
#36365=CARTESIAN_POINT('Ctrl Pts',(-7.27603390513785,-70.2795179709986,
-4.20082013374671));
#36366=CARTESIAN_POINT('Ctrl Pts',(-9.70137854017372,-70.1045179709986,
1.74701493417668E-11));
#36367=CARTESIAN_POINT('Ctrl Pts',(-7.27603390512272,-69.9295179709986,
4.20082013377292));
#36368=CARTESIAN_POINT('Ctrl Pts',(-4.85068927007173,-69.7545179709986,
8.40164026752836));
#36369=CARTESIAN_POINT('Ctrl Pts',(1.5129078685785E-11,-69.5795179709986,
8.40164026751963));
#36370=CARTESIAN_POINT('Ctrl Pts',(4.85068927010198,-69.4045179709986,8.4016402675109));
#36371=CARTESIAN_POINT('Ctrl Pts',(7.27603390513785,-69.2295179709986,4.20082013374672));
#36372=CARTESIAN_POINT('Ctrl Pts',(9.70137854017372,-69.0545179709986,-1.74689612655491E-11));
#36373=CARTESIAN_POINT('Ctrl Pts',(7.27603390512273,-68.8795179709986,-4.20082013377291));
#36374=CARTESIAN_POINT('Ctrl Pts',(4.85068927007173,-68.7045179709986,-8.40164026752836));
#36375=CARTESIAN_POINT('Ctrl Pts',(-1.51301075899711E-11,-68.5295179709986,
-8.40164026751963));
#36376=CARTESIAN_POINT('Ctrl Pts',(-4.85068927010199,-68.3545179709986,
-8.4016402675109));
#36377=CARTESIAN_POINT('Ctrl Pts',(-7.27603390513785,-68.1795179709986,
-4.20082013374671));
#36378=CARTESIAN_POINT('Ctrl Pts',(-9.70137854017372,-68.0045179709986,
1.74701493417668E-11));
#36379=CARTESIAN_POINT('Ctrl Pts',(-7.27603390512272,-67.8295179709986,
4.20082013377292));
#36380=CARTESIAN_POINT('Ctrl Pts',(-4.85068927007173,-67.6545179709986,
8.40164026752836));
#36381=CARTESIAN_POINT('Ctrl Pts',(1.5129078685785E-11,-67.4795179709986,
8.40164026751963));
#36382=CARTESIAN_POINT('Ctrl Pts',(4.85068927010198,-67.3045179709986,8.4016402675109));
#36383=CARTESIAN_POINT('Ctrl Pts',(7.27603390513785,-67.1295179709986,4.20082013374672));
#36384=CARTESIAN_POINT('Ctrl Pts',(9.70137854017372,-66.9545179709986,-1.74689612655491E-11));
#36385=CARTESIAN_POINT('Ctrl Pts',(7.27603390512273,-66.7795179709986,-4.20082013377291));
#36386=CARTESIAN_POINT('Ctrl Pts',(4.85068927007173,-66.6045179709986,-8.40164026752836));
#36387=CARTESIAN_POINT('Ctrl Pts',(-1.51301075899711E-11,-66.4295179709986,
-8.40164026751963));
#36388=CARTESIAN_POINT('Ctrl Pts',(-4.85068927010199,-66.2545179709986,
-8.4016402675109));
#36389=CARTESIAN_POINT('Ctrl Pts',(-7.27603390513785,-66.0795179709986,
-4.20082013374671));
#36390=CARTESIAN_POINT('Ctrl Pts',(-9.70137854017372,-65.9045179709986,
1.74701493417668E-11));
#36391=CARTESIAN_POINT('Ctrl Pts',(-7.27603390512272,-65.7295179709986,
4.20082013377292));
#36392=CARTESIAN_POINT('Ctrl Pts',(-4.85068927007173,-65.5545179709986,
8.40164026752836));
#36393=CARTESIAN_POINT('Ctrl Pts',(1.5129078685785E-11,-65.3795179709986,
8.40164026751963));
#36394=CARTESIAN_POINT('Ctrl Pts',(4.85068927010198,-65.2045179709986,8.4016402675109));
#36395=CARTESIAN_POINT('Ctrl Pts',(7.27603390513785,-65.0295179709986,4.20082013374672));
#36396=CARTESIAN_POINT('Ctrl Pts',(9.70137854017372,-64.8545179709986,-1.74689612655491E-11));
#36397=CARTESIAN_POINT('Ctrl Pts',(7.27603390512273,-64.6795179709986,-4.20082013377291));
#36398=CARTESIAN_POINT('Ctrl Pts',(4.85068927007173,-64.5045179709986,-8.40164026752836));
#36399=CARTESIAN_POINT('Ctrl Pts',(-1.51301075899711E-11,-64.3295179709986,
-8.40164026751963));
#36400=CARTESIAN_POINT('Ctrl Pts',(-4.85068927010199,-64.1545179709986,
-8.4016402675109));
#36401=CARTESIAN_POINT('Ctrl Pts',(-7.27603390513785,-63.9795179709986,
-4.20082013374671));
#36402=CARTESIAN_POINT('Ctrl Pts',(-9.70137854017372,-63.8045179709986,
1.74701493417668E-11));
#36403=CARTESIAN_POINT('Ctrl Pts',(-7.27603390512272,-63.6295179709986,
4.20082013377292));
#36404=CARTESIAN_POINT('Ctrl Pts',(-4.85068927007173,-63.4545179709986,
8.40164026752836));
#36405=CARTESIAN_POINT('Ctrl Pts',(1.5129078685785E-11,-63.2795179709986,
8.40164026751963));
#36406=CARTESIAN_POINT('Ctrl Pts',(4.85068927010198,-63.1045179709986,8.4016402675109));
#36407=CARTESIAN_POINT('Ctrl Pts',(7.27603390513785,-62.9295179709986,4.20082013374672));
#36408=CARTESIAN_POINT('Ctrl Pts',(9.70137854017372,-62.7545179709986,-1.74689612655491E-11));
#36409=CARTESIAN_POINT('Ctrl Pts',(7.27603390512273,-62.5795179709986,-4.20082013377291));
#36410=CARTESIAN_POINT('Ctrl Pts',(4.85068927007173,-62.4045179709986,-8.40164026752836));
#36411=CARTESIAN_POINT('Ctrl Pts',(-1.51301075899711E-11,-62.2295179709986,
-8.40164026751963));
#36412=CARTESIAN_POINT('Ctrl Pts',(-4.85068927010199,-62.0545179709986,
-8.4016402675109));
#36413=CARTESIAN_POINT('Ctrl Pts',(-7.27603390513785,-61.8795179709986,
-4.20082013374671));
#36414=CARTESIAN_POINT('Ctrl Pts',(-9.70137854017372,-61.7045179709986,
1.74701493417668E-11));
#36415=CARTESIAN_POINT('Ctrl Pts',(-7.27603390512272,-61.5295179709986,
4.20082013377292));
#36416=CARTESIAN_POINT('Ctrl Pts',(-4.85068927007173,-61.3545179709986,
8.40164026752836));
#36417=CARTESIAN_POINT('Ctrl Pts',(1.5129078685785E-11,-61.1795179709986,
8.40164026751963));
#36418=CARTESIAN_POINT('Ctrl Pts',(4.85068927010198,-61.0045179709986,8.4016402675109));
#36419=CARTESIAN_POINT('Ctrl Pts',(7.27603390513785,-60.8295179709986,4.20082013374672));
#36420=CARTESIAN_POINT('Ctrl Pts',(9.70137854017372,-60.6545179709986,-1.74689612655491E-11));
#36421=CARTESIAN_POINT('Ctrl Pts',(7.27603390512273,-60.4795179709986,-4.20082013377291));
#36422=CARTESIAN_POINT('Ctrl Pts',(4.85068927007173,-60.3045179709986,-8.40164026752836));
#36423=CARTESIAN_POINT('Ctrl Pts',(-1.51301075899711E-11,-60.1295179709986,
-8.40164026751963));
#36424=CARTESIAN_POINT('Ctrl Pts',(-4.85068927010199,-59.9545179709986,
-8.4016402675109));
#36425=CARTESIAN_POINT('Ctrl Pts',(-7.27603390513785,-59.7795179709986,
-4.20082013374671));
#36426=CARTESIAN_POINT('Ctrl Pts',(-9.70137854017372,-59.6045179709986,
1.74701493417668E-11));
#36427=CARTESIAN_POINT('Ctrl Pts',(-7.27603390512272,-59.4295179709986,
4.20082013377292));
#36428=CARTESIAN_POINT('Ctrl Pts',(-4.85068927007173,-59.2545179709986,
8.40164026752836));
#36429=CARTESIAN_POINT('Ctrl Pts',(1.5129078685785E-11,-59.0795179709986,
8.40164026751963));
#36430=CARTESIAN_POINT('Ctrl Pts',(4.85068927010198,-58.9045179709986,8.4016402675109));
#36431=CARTESIAN_POINT('Ctrl Pts',(7.27603390513785,-58.7295179709986,4.20082013374672));
#36432=CARTESIAN_POINT('Ctrl Pts',(9.70137854017372,-58.5545179709986,-1.74689612655491E-11));
#36433=CARTESIAN_POINT('Ctrl Pts',(7.27603390512273,-58.3795179709986,-4.20082013377291));
#36434=CARTESIAN_POINT('Ctrl Pts',(4.85068927007173,-58.2045179709986,-8.40164026752836));
#36435=CARTESIAN_POINT('Ctrl Pts',(-1.51301075899711E-11,-58.0295179709986,
-8.40164026751963));
#36436=CARTESIAN_POINT('Ctrl Pts',(-4.85068927010199,-57.8545179709986,
-8.4016402675109));
#36437=CARTESIAN_POINT('Ctrl Pts',(-7.27603390513785,-57.6795179709986,
-4.20082013374671));
#36438=CARTESIAN_POINT('Ctrl Pts',(-9.70137854017372,-57.5045179709986,
1.74701493417668E-11));
#36439=CARTESIAN_POINT('Ctrl Pts',(-7.27603390512272,-57.3295179709986,
4.20082013377292));
#36440=CARTESIAN_POINT('Ctrl Pts',(-4.85068927007173,-57.1545179709986,
8.40164026752836));
#36441=CARTESIAN_POINT('Ctrl Pts',(1.5129078685785E-11,-56.9795179709986,
8.40164026751963));
#36442=CARTESIAN_POINT('Ctrl Pts',(4.85068927010198,-56.8045179709986,8.4016402675109));
#36443=CARTESIAN_POINT('Ctrl Pts',(7.27603390513785,-56.6295179709986,4.20082013374672));
#36444=CARTESIAN_POINT('Ctrl Pts',(9.70137854017372,-56.4545179709986,-1.74689612655491E-11));
#36445=CARTESIAN_POINT('Ctrl Pts',(7.27603390512273,-56.2795179709986,-4.20082013377291));
#36446=CARTESIAN_POINT('Ctrl Pts',(4.85068927007173,-56.1045179709986,-8.40164026752836));
#36447=CARTESIAN_POINT('Ctrl Pts',(-1.51301075899711E-11,-55.9295179709986,
-8.40164026751963));
#36448=CARTESIAN_POINT('Ctrl Pts',(-4.85068927010199,-55.7545179709987,
-8.4016402675109));
#36449=CARTESIAN_POINT('Ctrl Pts',(-7.27603390513785,-55.5795179709986,
-4.20082013374671));
#36450=CARTESIAN_POINT('Ctrl Pts',(-9.70137854017372,-55.4045179709986,
1.74701493417668E-11));
#36451=CARTESIAN_POINT('Ctrl Pts',(-7.27603390512272,-55.2295179709986,
4.20082013377292));
#36452=CARTESIAN_POINT('Ctrl Pts',(-4.85068927007173,-55.0545179709987,
8.40164026752836));
#36453=CARTESIAN_POINT('Ctrl Pts',(1.5129078685785E-11,-54.8795179709986,
8.40164026751963));
#36454=CARTESIAN_POINT('Ctrl Pts',(4.85068927010198,-54.7045179709987,8.4016402675109));
#36455=CARTESIAN_POINT('Ctrl Pts',(7.27603390513785,-54.5295179709986,4.20082013374672));
#36456=CARTESIAN_POINT('Ctrl Pts',(9.70137854017372,-54.3545179709986,-1.74689612655491E-11));
#36457=CARTESIAN_POINT('Ctrl Pts',(7.27603390512273,-54.1795179709986,-4.20082013377291));
#36458=CARTESIAN_POINT('Ctrl Pts',(4.85068927007173,-54.0045179709987,-8.40164026752836));
#36459=CARTESIAN_POINT('Ctrl Pts',(-1.51301075899711E-11,-53.8295179709986,
-8.40164026751963));
#36460=CARTESIAN_POINT('Ctrl Pts',(-4.85068927010199,-53.6545179709986,
-8.4016402675109));
#36461=CARTESIAN_POINT('Ctrl Pts',(-7.27603390513785,-53.4795179709987,
-4.20082013374671));
#36462=CARTESIAN_POINT('Ctrl Pts',(-9.70137854017372,-53.3045179709987,
1.74701493417668E-11));
#36463=CARTESIAN_POINT('Ctrl Pts',(-7.27603390512272,-53.1295179709986,
4.20082013377292));
#36464=CARTESIAN_POINT('Ctrl Pts',(-4.85068927007173,-52.9545179709987,
8.40164026752836));
#36465=CARTESIAN_POINT('Ctrl Pts',(1.5129078685785E-11,-52.7795179709986,
8.40164026751963));
#36466=CARTESIAN_POINT('Ctrl Pts',(4.85068927010198,-52.6045179709986,8.4016402675109));
#36467=CARTESIAN_POINT('Ctrl Pts',(7.27603390513785,-52.4295179709987,4.20082013374672));
#36468=CARTESIAN_POINT('Ctrl Pts',(9.70137854017372,-52.2545179709986,-1.74689612655491E-11));
#36469=CARTESIAN_POINT('Ctrl Pts',(7.27603390512273,-52.0795179709986,-4.20082013377291));
#36470=CARTESIAN_POINT('Ctrl Pts',(4.85068927007173,-51.9045179709987,-8.40164026752836));
#36471=CARTESIAN_POINT('Ctrl Pts',(-1.51301075899711E-11,-51.7295179709986,
-8.40164026751963));
#36472=CARTESIAN_POINT('Ctrl Pts',(-4.85068927010199,-51.5545179709986,
-8.4016402675109));
#36473=CARTESIAN_POINT('Ctrl Pts',(-7.27603390513785,-51.3795179709987,
-4.20082013374671));
#36474=CARTESIAN_POINT('Ctrl Pts',(-9.70137854017372,-51.2045179709987,
1.74701493417668E-11));
#36475=CARTESIAN_POINT('Ctrl Pts',(-7.27603390512272,-51.0295179709986,
4.20082013377292));
#36476=CARTESIAN_POINT('Ctrl Pts',(-4.85068927007173,-50.8545179709987,
8.40164026752836));
#36477=CARTESIAN_POINT('Ctrl Pts',(1.5129078685785E-11,-50.6795179709987,
8.40164026751963));
#36478=CARTESIAN_POINT('Ctrl Pts',(4.85068927010198,-50.5045179709986,8.4016402675109));
#36479=CARTESIAN_POINT('Ctrl Pts',(7.27603390513785,-50.3295179709987,4.20082013374672));
#36480=CARTESIAN_POINT('Ctrl Pts',(9.70137854017372,-50.1545179709987,-1.74689612655491E-11));
#36481=CARTESIAN_POINT('Ctrl Pts',(7.27603390512273,-49.9795179709986,-4.20082013377291));
#36482=CARTESIAN_POINT('Ctrl Pts',(4.85068927007173,-49.8045179709986,-8.40164026752836));
#36483=CARTESIAN_POINT('Ctrl Pts',(-1.51301075899711E-11,-49.6295179709987,
-8.40164026751963));
#36484=CARTESIAN_POINT('Ctrl Pts',(-4.85068927010199,-49.4545179709986,
-8.4016402675109));
#36485=CARTESIAN_POINT('Ctrl Pts',(-7.27603390513785,-49.2795179709986,
-4.20082013374671));
#36486=CARTESIAN_POINT('Ctrl Pts',(-9.70137854017372,-49.1045179709987,
1.74701493417668E-11));
#36487=CARTESIAN_POINT('Ctrl Pts',(-7.27603390512272,-48.9295179709987,
4.20082013377292));
#36488=CARTESIAN_POINT('Ctrl Pts',(-4.85068927007173,-48.7545179709986,
8.40164026752836));
#36489=CARTESIAN_POINT('Ctrl Pts',(1.5129078685785E-11,-48.5795179709987,
8.40164026751963));
#36490=CARTESIAN_POINT('Ctrl Pts',(4.85068927010198,-48.4045179709987,8.4016402675109));
#36491=CARTESIAN_POINT('Ctrl Pts',(7.27603390513785,-48.2295179709986,4.20082013374672));
#36492=CARTESIAN_POINT('Ctrl Pts',(9.70137854017372,-48.0545179709987,-1.74689612655491E-11));
#36493=CARTESIAN_POINT('Ctrl Pts',(7.27603390512273,-47.8795179709987,-4.20082013377291));
#36494=CARTESIAN_POINT('Ctrl Pts',(4.85068927007173,-47.7045179709986,-8.40164026752836));
#36495=CARTESIAN_POINT('Ctrl Pts',(-1.51301075899711E-11,-47.5295179709987,
-8.40164026751963));
#36496=CARTESIAN_POINT('Ctrl Pts',(-4.85068927010199,-47.3545179709987,
-8.4016402675109));
#36497=CARTESIAN_POINT('Ctrl Pts',(-7.27603390513785,-47.1795179709986,
-4.20082013374671));
#36498=CARTESIAN_POINT('Ctrl Pts',(-9.70137854017372,-47.0045179709987,
1.74701493417668E-11));
#36499=CARTESIAN_POINT('Ctrl Pts',(-7.27603390512272,-46.8295179709987,
4.20082013377292));
#36500=CARTESIAN_POINT('Ctrl Pts',(-4.85068927007173,-46.6545179709987,
8.40164026752836));
#36501=CARTESIAN_POINT('Ctrl Pts',(1.5129078685785E-11,-46.4795179709987,
8.40164026751963));
#36502=CARTESIAN_POINT('Ctrl Pts',(4.85068927010198,-46.3045179709987,8.4016402675109));
#36503=CARTESIAN_POINT('Ctrl Pts',(7.27603390513785,-46.1295179709986,4.20082013374672));
#36504=CARTESIAN_POINT('Ctrl Pts',(9.70137854017372,-45.9545179709987,-1.74689612655491E-11));
#36505=CARTESIAN_POINT('Ctrl Pts',(7.27603390512273,-45.7795179709987,-4.20082013377291));
#36506=CARTESIAN_POINT('Ctrl Pts',(4.85068927007173,-45.6045179709986,-8.40164026752836));
#36507=CARTESIAN_POINT('Ctrl Pts',(-1.51301075899711E-11,-45.4295179709987,
-8.40164026751963));
#36508=CARTESIAN_POINT('Ctrl Pts',(-4.85068927010199,-45.2545179709987,
-8.4016402675109));
#36509=CARTESIAN_POINT('Ctrl Pts',(-7.27603390513785,-45.0795179709987,
-4.20082013374671));
#36510=CARTESIAN_POINT('Ctrl Pts',(-9.70137854017372,-44.9045179709986,
1.74701493417668E-11));
#36511=CARTESIAN_POINT('Ctrl Pts',(-7.27603390512272,-44.7295179709987,
4.20082013377292));
#36512=CARTESIAN_POINT('Ctrl Pts',(-4.85068927007173,-44.5545179709987,
8.40164026752836));
#36513=CARTESIAN_POINT('Ctrl Pts',(1.5129078685785E-11,-44.3795179709986,
8.40164026751963));
#36514=CARTESIAN_POINT('Ctrl Pts',(4.85068927010198,-44.2045179709987,8.4016402675109));
#36515=CARTESIAN_POINT('Ctrl Pts',(7.27603390513785,-44.0295179709987,4.20082013374672));
#36516=CARTESIAN_POINT('Ctrl Pts',(9.70137854017372,-43.8545179709986,-1.74689612655491E-11));
#36517=CARTESIAN_POINT('Ctrl Pts',(7.27603390512273,-43.6795179709987,-4.20082013377291));
#36518=CARTESIAN_POINT('Ctrl Pts',(4.85068927007173,-43.5045179709987,-8.40164026752836));
#36519=CARTESIAN_POINT('Ctrl Pts',(-1.51301075899711E-11,-43.3295179709987,
-8.40164026751963));
#36520=CARTESIAN_POINT('',(-5.67113674141202,-212.63,6.19885209091279));
#36521=CARTESIAN_POINT('Ctrl Pts',(-5.67113674141202,-212.63,6.19885209091279));
#36522=CARTESIAN_POINT('Ctrl Pts',(-3.26337288082243,-212.49725180682,8.40164026752551));
#36523=CARTESIAN_POINT('Ctrl Pts',(1.5129078685785E-11,-212.379517970998,
8.40164026751963));
#36524=CARTESIAN_POINT('Ctrl Pts',(4.85068927010198,-212.204517970998,8.4016402675109));
#36525=CARTESIAN_POINT('Ctrl Pts',(7.27603390513785,-212.029517970998,4.20082013374672));
#36526=CARTESIAN_POINT('Ctrl Pts',(9.70137854017372,-211.854517970998,-1.74689612655491E-11));
#36527=CARTESIAN_POINT('Ctrl Pts',(7.27603390512273,-211.679517970998,-4.20082013377291));
#36528=CARTESIAN_POINT('Ctrl Pts',(4.85068927007173,-211.504517970998,-8.40164026752836));
#36529=CARTESIAN_POINT('Ctrl Pts',(-1.51280497815988E-11,-211.329517970998,
-8.40164026751963));
#36530=CARTESIAN_POINT('Ctrl Pts',(-4.85068927010198,-211.154517970998,
-8.4016402675109));
#36531=CARTESIAN_POINT('Ctrl Pts',(-7.27603390513785,-210.979517970998,
-4.20082013374672));
#36532=CARTESIAN_POINT('Ctrl Pts',(-9.70137854017372,-210.804517970998,
1.74591566342707E-11));
#36533=CARTESIAN_POINT('Ctrl Pts',(-7.27603390512273,-210.629517970998,
4.20082013377291));
#36534=CARTESIAN_POINT('Ctrl Pts',(-4.85068927007174,-210.454517970998,
8.40164026752836));
#36535=CARTESIAN_POINT('Ctrl Pts',(1.51270208774127E-11,-210.279517970998,
8.40164026751963));
#36536=CARTESIAN_POINT('Ctrl Pts',(4.85068927010198,-210.104517970998,8.4016402675109));
#36537=CARTESIAN_POINT('Ctrl Pts',(7.27603390513785,-209.929517970998,4.20082013374672));
#36538=CARTESIAN_POINT('Ctrl Pts',(9.70137854017372,-209.754517970998,-1.74665851131138E-11));
#36539=CARTESIAN_POINT('Ctrl Pts',(7.27603390512273,-209.579517970998,-4.20082013377291));
#36540=CARTESIAN_POINT('Ctrl Pts',(4.85068927007174,-209.404517970998,-8.40164026752836));
#36541=CARTESIAN_POINT('Ctrl Pts',(-1.51259919732266E-11,-209.229517970998,
-8.40164026751963));
#36542=CARTESIAN_POINT('Ctrl Pts',(-4.85068927010198,-209.054517970998,
-8.4016402675109));
#36543=CARTESIAN_POINT('Ctrl Pts',(-7.27603390513785,-208.879517970998,
-4.20082013374672));
#36544=CARTESIAN_POINT('Ctrl Pts',(-9.70137854017372,-208.704517970998,
1.74481639267747E-11));
#36545=CARTESIAN_POINT('Ctrl Pts',(-7.27603390512273,-208.529517970998,
4.20082013377291));
#36546=CARTESIAN_POINT('Ctrl Pts',(-4.85068927007174,-208.354517970998,
8.40164026752836));
#36547=CARTESIAN_POINT('Ctrl Pts',(1.51100387578891E-11,-208.179517970998,
8.40164026751963));
#36548=CARTESIAN_POINT('Ctrl Pts',(4.85068927010198,-208.004517970998,8.4016402675109));
#36549=CARTESIAN_POINT('Ctrl Pts',(7.27603390513784,-207.829517970998,4.20082013374673));
#36550=CARTESIAN_POINT('Ctrl Pts',(9.70137854017372,-207.654517970998,-1.74469758505571E-11));
#36551=CARTESIAN_POINT('Ctrl Pts',(7.27603390512273,-207.479517970998,-4.2008201337729));
#36552=CARTESIAN_POINT('Ctrl Pts',(4.85068927007176,-207.304517970998,-8.40164026752835));
#36553=CARTESIAN_POINT('Ctrl Pts',(-1.51239341648544E-11,-207.129517970998,
-8.40164026751963));
#36554=CARTESIAN_POINT('Ctrl Pts',(-4.85068927010198,-206.954517970998,
-8.4016402675109));
#36555=CARTESIAN_POINT('Ctrl Pts',(-7.27603390513784,-206.779517970998,
-4.20082013374673));
#36556=CARTESIAN_POINT('Ctrl Pts',(-9.70137854017372,-206.604517970998,
1.74457877743394E-11));
#36557=CARTESIAN_POINT('Ctrl Pts',(-7.27603390512273,-206.429517970998,
4.20082013377289));
#36558=CARTESIAN_POINT('Ctrl Pts',(-4.85068927007176,-206.254517970998,
8.40164026752835));
#36559=CARTESIAN_POINT('Ctrl Pts',(1.51229052606682E-11,-206.079517970998,
8.40164026751963));
#36560=CARTESIAN_POINT('Ctrl Pts',(4.85068927010198,-205.904517970998,8.4016402675109));
#36561=CARTESIAN_POINT('Ctrl Pts',(7.27603390513784,-205.729517970998,4.20082013374673));
#36562=CARTESIAN_POINT('Ctrl Pts',(9.70137854017372,-205.554517970998,-1.74445996981217E-11));
#36563=CARTESIAN_POINT('Ctrl Pts',(7.27603390512273,-205.379517970998,-4.20082013377289));
#36564=CARTESIAN_POINT('Ctrl Pts',(4.85068927007176,-205.204517970998,-8.40164026752835));
#36565=CARTESIAN_POINT('Ctrl Pts',(-1.51218763564821E-11,-205.029517970998,
-8.40164026751963));
#36566=CARTESIAN_POINT('Ctrl Pts',(-4.85068927010197,-204.854517970998,
-8.4016402675109));
#36567=CARTESIAN_POINT('Ctrl Pts',(-7.27603390513784,-204.679517970998,
-4.20082013374673));
#36568=CARTESIAN_POINT('Ctrl Pts',(-9.70137854017372,-204.504517970998,
1.74434116219041E-11));
#36569=CARTESIAN_POINT('Ctrl Pts',(-7.27603390512274,-204.329517970998,
4.20082013377289));
#36570=CARTESIAN_POINT('Ctrl Pts',(-4.85068927007176,-204.154517970998,
8.40164026752834));
#36571=CARTESIAN_POINT('Ctrl Pts',(1.50909988299932E-11,-203.979517970998,
8.40164026751963));
#36572=CARTESIAN_POINT('Ctrl Pts',(4.85068927010197,-203.804517970998,8.4016402675109));
#36573=CARTESIAN_POINT('Ctrl Pts',(7.27603390513784,-203.629517970998,4.20082013374673));
#36574=CARTESIAN_POINT('Ctrl Pts',(9.70137854017372,-203.454517970998,-1.74422235456864E-11));
#36575=CARTESIAN_POINT('Ctrl Pts',(7.27603390512274,-203.279517970998,-4.20082013377289));
#36576=CARTESIAN_POINT('Ctrl Pts',(4.85068927007176,-203.104517970998,-8.40164026752834));
#36577=CARTESIAN_POINT('Ctrl Pts',(-1.50899699258071E-11,-202.929517970998,
-8.40164026751963));
#36578=CARTESIAN_POINT('Ctrl Pts',(-4.85068927010197,-202.754517970998,
-8.4016402675109));
#36579=CARTESIAN_POINT('Ctrl Pts',(-7.27603390513784,-202.579517970998,
-4.20082013374673));
#36580=CARTESIAN_POINT('Ctrl Pts',(-9.70137854017372,-202.404517970998,
1.74065692492259E-11));
#36581=CARTESIAN_POINT('Ctrl Pts',(-7.27603390512274,-202.229517970998,
4.20082013377289));
#36582=CARTESIAN_POINT('Ctrl Pts',(-4.85068927007173,-202.054517970998,
8.40164026752836));
#36583=CARTESIAN_POINT('Ctrl Pts',(1.5088941021621E-11,-201.879517970998,
8.40164026751963));
#36584=CARTESIAN_POINT('Ctrl Pts',(4.85068927010197,-201.704517970998,8.4016402675109));
#36585=CARTESIAN_POINT('Ctrl Pts',(7.27603390513783,-201.529517970998,4.20082013374676));
#36586=CARTESIAN_POINT('Ctrl Pts',(9.70137854017372,-201.354517970998,-1.74398473932511E-11));
#36587=CARTESIAN_POINT('Ctrl Pts',(7.27603390512275,-201.179517970998,-4.20082013377287));
#36588=CARTESIAN_POINT('Ctrl Pts',(4.85068927007176,-201.004517970998,-8.40164026752834));
#36589=CARTESIAN_POINT('Ctrl Pts',(-1.51177607397376E-11,-200.829517970998,
-8.40164026751963));
#36590=CARTESIAN_POINT('Ctrl Pts',(-4.85068927010194,-200.654517970998,
-8.40164026751092));
#36591=CARTESIAN_POINT('Ctrl Pts',(-7.27603390513784,-200.479517970998,
-4.20082013374673));
#36592=CARTESIAN_POINT('Ctrl Pts',(-9.70137854017372,-200.304517970998,
1.74041930967906E-11));
#36593=CARTESIAN_POINT('Ctrl Pts',(-7.27603390512274,-200.129517970998,
4.20082013377289));
#36594=CARTESIAN_POINT('Ctrl Pts',(-4.85068927007174,-199.954517970998,
8.40164026752836));
#36595=CARTESIAN_POINT('Ctrl Pts',(1.50868832132487E-11,-199.779517970998,
8.40164026751963));
#36596=CARTESIAN_POINT('Ctrl Pts',(4.85068927010197,-199.604517970998,8.4016402675109));
#36597=CARTESIAN_POINT('Ctrl Pts',(7.27603390513783,-199.429517970998,4.20082013374676));
#36598=CARTESIAN_POINT('Ctrl Pts',(9.70137854017372,-199.254517970998,-1.74374712408158E-11));
#36599=CARTESIAN_POINT('Ctrl Pts',(7.27603390512275,-199.079517970998,-4.20082013377286));
#36600=CARTESIAN_POINT('Ctrl Pts',(4.85068927007177,-198.904517970998,-8.40164026752834));
#36601=CARTESIAN_POINT('Ctrl Pts',(-1.51157029313654E-11,-198.729517970998,
-8.40164026751963));
#36602=CARTESIAN_POINT('Ctrl Pts',(-4.85068927010194,-198.554517970998,
-8.40164026751092));
#36603=CARTESIAN_POINT('Ctrl Pts',(-7.27603390513784,-198.379517970998,
-4.20082013374673));
#36604=CARTESIAN_POINT('Ctrl Pts',(-9.70137854017372,-198.204517970998,
1.74018169443553E-11));
#36605=CARTESIAN_POINT('Ctrl Pts',(-7.27603390512274,-198.029517970998,
4.20082013377289));
#36606=CARTESIAN_POINT('Ctrl Pts',(-4.8506892700718,-197.854517970998,8.40164026752832));
#36607=CARTESIAN_POINT('Ctrl Pts',(1.50848254048765E-11,-197.679517970998,
8.40164026751963));
#36608=CARTESIAN_POINT('Ctrl Pts',(4.85068927010197,-197.504517970998,8.4016402675109));
#36609=CARTESIAN_POINT('Ctrl Pts',(7.27603390513782,-197.329517970998,4.20082013374676));
#36610=CARTESIAN_POINT('Ctrl Pts',(9.70137854017372,-197.154517970998,-1.74350950883805E-11));
#36611=CARTESIAN_POINT('Ctrl Pts',(7.27603390512276,-196.979517970998,-4.20082013377286));
#36612=CARTESIAN_POINT('Ctrl Pts',(4.85068927007177,-196.804517970998,-8.40164026752834));
#36613=CARTESIAN_POINT('Ctrl Pts',(-1.51136451229931E-11,-196.629517970998,
-8.40164026751963));
#36614=CARTESIAN_POINT('Ctrl Pts',(-4.85068927010194,-196.454517970998,
-8.40164026751092));
#36615=CARTESIAN_POINT('Ctrl Pts',(-7.27603390513784,-196.279517970998,
-4.20082013374673));
#36616=CARTESIAN_POINT('Ctrl Pts',(-9.70137854017372,-196.104517970998,
1.739944079192E-11));
#36617=CARTESIAN_POINT('Ctrl Pts',(-7.27603390512274,-195.929517970998,
4.20082013377289));
#36618=CARTESIAN_POINT('Ctrl Pts',(-4.8506892700718,-195.754517970998,8.40164026752832));
#36619=CARTESIAN_POINT('Ctrl Pts',(1.50827675965043E-11,-195.579517970998,
8.40164026751963));
#36620=CARTESIAN_POINT('Ctrl Pts',(4.85068927010196,-195.404517970998,8.40164026751091));
#36621=CARTESIAN_POINT('Ctrl Pts',(7.27603390513782,-195.229517970998,4.20082013374676));
#36622=CARTESIAN_POINT('Ctrl Pts',(9.70137854017372,-195.054517970998,-1.74327189359452E-11));
#36623=CARTESIAN_POINT('Ctrl Pts',(7.27603390512276,-194.879517970998,-4.20082013377286));
#36624=CARTESIAN_POINT('Ctrl Pts',(4.85068927007177,-194.704517970998,-8.40164026752834));
#36625=CARTESIAN_POINT('Ctrl Pts',(-1.50518900700154E-11,-194.529517970998,
-8.40164026751963));
#36626=CARTESIAN_POINT('Ctrl Pts',(-4.85068927010193,-194.354517970998,
-8.40164026751092));
#36627=CARTESIAN_POINT('Ctrl Pts',(-7.27603390513784,-194.179517970998,
-4.20082013374674));
#36628=CARTESIAN_POINT('Ctrl Pts',(-9.70137854017372,-194.004517970998,
1.73970646394847E-11));
#36629=CARTESIAN_POINT('Ctrl Pts',(-7.27603390512274,-193.829517970998,
4.20082013377288));
#36630=CARTESIAN_POINT('Ctrl Pts',(-4.8506892700718,-193.654517970998,8.40164026752832));
#36631=CARTESIAN_POINT('Ctrl Pts',(1.5080709788132E-11,-193.479517970998,
8.40164026751963));
#36632=CARTESIAN_POINT('Ctrl Pts',(4.8506892701019,-193.304517970998,8.40164026751094));
#36633=CARTESIAN_POINT('Ctrl Pts',(7.27603390513782,-193.129517970998,4.20082013374676));
#36634=CARTESIAN_POINT('Ctrl Pts',(9.70137854017372,-192.954517970998,-1.74303427835099E-11));
#36635=CARTESIAN_POINT('Ctrl Pts',(7.27603390512276,-192.779517970998,-4.20082013377286));
#36636=CARTESIAN_POINT('Ctrl Pts',(4.85068927007177,-192.604517970998,-8.40164026752834));
#36637=CARTESIAN_POINT('Ctrl Pts',(-1.50498322616431E-11,-192.429517970998,
-8.40164026751963));
#36638=CARTESIAN_POINT('Ctrl Pts',(-4.85068927010193,-192.254517970998,
-8.40164026751093));
#36639=CARTESIAN_POINT('Ctrl Pts',(-7.27603390513784,-192.079517970998,
-4.20082013374674));
#36640=CARTESIAN_POINT('Ctrl Pts',(-9.70137854017372,-191.904517970998,
1.73946884870493E-11));
#36641=CARTESIAN_POINT('Ctrl Pts',(-7.27603390512274,-191.729517970998,
4.20082013377288));
#36642=CARTESIAN_POINT('Ctrl Pts',(-4.85068927007174,-191.554517970998,
8.40164026752836));
#36643=CARTESIAN_POINT('Ctrl Pts',(1.50189547351542E-11,-191.379517970998,
8.40164026751963));
#36644=CARTESIAN_POINT('Ctrl Pts',(4.8506892701019,-191.204517970998,8.40164026751094));
#36645=CARTESIAN_POINT('Ctrl Pts',(7.27603390513782,-191.029517970998,4.20082013374676));
#36646=CARTESIAN_POINT('Ctrl Pts',(9.70137854017372,-190.854517970998,-1.74279666310746E-11));
#36647=CARTESIAN_POINT('Ctrl Pts',(7.27603390512273,-190.679517970998,-4.20082013377291));
#36648=CARTESIAN_POINT('Ctrl Pts',(4.85068927007184,-190.504517970998,-8.4016402675283));
#36649=CARTESIAN_POINT('Ctrl Pts',(-1.50477744532709E-11,-190.329517970998,
-8.40164026751963));
#36650=CARTESIAN_POINT('Ctrl Pts',(-4.85068927010193,-190.154517970998,
-8.40164026751093));
#36651=CARTESIAN_POINT('Ctrl Pts',(-7.27603390513784,-189.979517970998,
-4.20082013374674));
#36652=CARTESIAN_POINT('Ctrl Pts',(-9.70137854017372,-189.804517970998,
1.74612447750998E-11));
#36653=CARTESIAN_POINT('Ctrl Pts',(-7.27603390512277,-189.629517970998,
4.20082013377283));
#36654=CARTESIAN_POINT('Ctrl Pts',(-4.8506892700718,-189.454517970998,8.40164026752832));
#36655=CARTESIAN_POINT('Ctrl Pts',(1.50765941713875E-11,-189.279517970998,
8.40164026751963));
#36656=CARTESIAN_POINT('Ctrl Pts',(4.85068927010196,-189.104517970998,8.40164026751091));
#36657=CARTESIAN_POINT('Ctrl Pts',(7.27603390513779,-188.929517970998,4.20082013374682));
#36658=CARTESIAN_POINT('Ctrl Pts',(9.70137854017372,-188.754517970998,-1.73566580381535E-11));
#36659=CARTESIAN_POINT('Ctrl Pts',(7.27603390512276,-188.579517970998,-4.20082013377285));
#36660=CARTESIAN_POINT('Ctrl Pts',(4.85068927007178,-188.404517970998,-8.40164026752834));
#36661=CARTESIAN_POINT('Ctrl Pts',(-1.51054138895042E-11,-188.229517970998,
-8.40164026751963));
#36662=CARTESIAN_POINT('Ctrl Pts',(-4.85068927010187,-188.054517970998,
-8.40164026751096));
#36663=CARTESIAN_POINT('Ctrl Pts',(-7.27603390513781,-187.879517970998,
-4.20082013374679));
#36664=CARTESIAN_POINT('Ctrl Pts',(-9.70137854017372,-187.704517970998,
1.73899361821787E-11));
#36665=CARTESIAN_POINT('Ctrl Pts',(-7.27603390512274,-187.529517970998,
4.20082013377288));
#36666=CARTESIAN_POINT('Ctrl Pts',(-4.85068927007175,-187.354517970998,
8.40164026752835));
#36667=CARTESIAN_POINT('Ctrl Pts',(1.50148391184097E-11,-187.179517970998,
8.40164026751963));
#36668=CARTESIAN_POINT('Ctrl Pts',(4.8506892701019,-187.004517970998,8.40164026751095));
#36669=CARTESIAN_POINT('Ctrl Pts',(7.27603390513782,-186.829517970998,4.20082013374677));
#36670=CARTESIAN_POINT('Ctrl Pts',(9.70137854017372,-186.654517970998,-1.7423214326204E-11));
#36671=CARTESIAN_POINT('Ctrl Pts',(7.27603390512273,-186.479517970998,-4.2008201337729));
#36672=CARTESIAN_POINT('Ctrl Pts',(4.85068927007184,-186.304517970998,-8.4016402675283));
#36673=CARTESIAN_POINT('Ctrl Pts',(-1.50436588365264E-11,-186.129517970998,
-8.40164026751963));
#36674=CARTESIAN_POINT('Ctrl Pts',(-4.85068927010193,-185.954517970998,
-8.40164026751093));
#36675=CARTESIAN_POINT('Ctrl Pts',(-7.27603390513783,-185.779517970998,
-4.20082013374674));
#36676=CARTESIAN_POINT('Ctrl Pts',(-9.70137854017372,-185.604517970998,
1.73186275892576E-11));
#36677=CARTESIAN_POINT('Ctrl Pts',(-7.27603390512277,-185.429517970998,
4.20082013377283));
#36678=CARTESIAN_POINT('Ctrl Pts',(-4.85068927007181,-185.254517970998,
8.40164026752832));
#36679=CARTESIAN_POINT('Ctrl Pts',(1.5072478554643E-11,-185.079517970998,
8.40164026751963));
#36680=CARTESIAN_POINT('Ctrl Pts',(4.85068927010196,-184.904517970998,8.40164026751091));
#36681=CARTESIAN_POINT('Ctrl Pts',(7.27603390513779,-184.729517970998,4.20082013374682));
#36682=CARTESIAN_POINT('Ctrl Pts',(9.70137854017372,-184.554517970998,-1.73519057332829E-11));
#36683=CARTESIAN_POINT('Ctrl Pts',(7.27603390512276,-184.379517970998,-4.20082013377285));
#36684=CARTESIAN_POINT('Ctrl Pts',(4.85068927007178,-184.204517970998,-8.40164026752833));
#36685=CARTESIAN_POINT('Ctrl Pts',(-1.51012982727597E-11,-184.029517970998,
-8.40164026751963));
#36686=CARTESIAN_POINT('Ctrl Pts',(-4.85068927010186,-183.854517970998,
-8.40164026751097));
#36687=CARTESIAN_POINT('Ctrl Pts',(-7.2760339051378,-183.679517970998,-4.2008201337468));
#36688=CARTESIAN_POINT('Ctrl Pts',(-9.70137854017372,-183.504517970998,
1.73851838773081E-11));
#36689=CARTESIAN_POINT('Ctrl Pts',(-7.27603390512275,-183.329517970998,
4.20082013377288));
#36690=CARTESIAN_POINT('Ctrl Pts',(-4.85068927007175,-183.154517970998,
8.40164026752835));
#36691=CARTESIAN_POINT('Ctrl Pts',(1.50107235016652E-11,-182.979517970998,
8.40164026751963));
#36692=CARTESIAN_POINT('Ctrl Pts',(4.85068927010189,-182.804517970998,8.40164026751095));
#36693=CARTESIAN_POINT('Ctrl Pts',(7.27603390513782,-182.629517970998,4.20082013374677));
#36694=CARTESIAN_POINT('Ctrl Pts',(9.70137854017372,-182.454517970998,-1.74184620213334E-11));
#36695=CARTESIAN_POINT('Ctrl Pts',(7.27603390512279,-182.279517970998,-4.2008201337728));
#36696=CARTESIAN_POINT('Ctrl Pts',(4.85068927007184,-182.104517970998,-8.4016402675283));
#36697=CARTESIAN_POINT('Ctrl Pts',(-1.50395432197819E-11,-181.929517970998,
-8.40164026751963));
#36698=CARTESIAN_POINT('Ctrl Pts',(-4.85068927010192,-181.754517970998,
-8.40164026751093));
#36699=CARTESIAN_POINT('Ctrl Pts',(-7.27603390513783,-181.579517970998,
-4.20082013374675));
#36700=CARTESIAN_POINT('Ctrl Pts',(-9.70137854017372,-181.404517970998,
1.7313875284387E-11));
#36701=CARTESIAN_POINT('Ctrl Pts',(-7.27603390512278,-181.229517970998,
4.20082013377282));
#36702=CARTESIAN_POINT('Ctrl Pts',(-4.85068927007181,-181.054517970998,
8.40164026752832));
#36703=CARTESIAN_POINT('Ctrl Pts',(1.50683629378986E-11,-180.879517970998,
8.40164026751963));
#36704=CARTESIAN_POINT('Ctrl Pts',(4.85068927010195,-180.704517970998,8.40164026751092));
#36705=CARTESIAN_POINT('Ctrl Pts',(7.27603390513779,-180.529517970998,4.20082013374683));
#36706=CARTESIAN_POINT('Ctrl Pts',(9.70137854017372,-180.354517970998,-1.73471534284123E-11));
#36707=CARTESIAN_POINT('Ctrl Pts',(7.27603390512276,-180.179517970998,-4.20082013377285));
#36708=CARTESIAN_POINT('Ctrl Pts',(4.85068927007178,-180.004517970998,-8.40164026752833));
#36709=CARTESIAN_POINT('Ctrl Pts',(-1.50971826560152E-11,-179.829517970998,
-8.40164026751963));
#36710=CARTESIAN_POINT('Ctrl Pts',(-4.85068927010186,-179.654517970998,
-8.40164026751097));
#36711=CARTESIAN_POINT('Ctrl Pts',(-7.2760339051378,-179.479517970998,-4.2008201337468));
#36712=CARTESIAN_POINT('Ctrl Pts',(-9.70137854017372,-179.304517970998,
1.73804315724375E-11));
#36713=CARTESIAN_POINT('Ctrl Pts',(-7.27603390512275,-179.129517970998,
4.20082013377287));
#36714=CARTESIAN_POINT('Ctrl Pts',(-4.85068927007188,-178.954517970998,
8.40164026752828));
#36715=CARTESIAN_POINT('Ctrl Pts',(1.50066078849208E-11,-178.779517970998,
8.40164026751963));
#36716=CARTESIAN_POINT('Ctrl Pts',(4.85068927010189,-178.604517970998,8.40164026751095));
#36717=CARTESIAN_POINT('Ctrl Pts',(7.27603390513782,-178.429517970998,4.20082013374678));
#36718=CARTESIAN_POINT('Ctrl Pts',(9.70137854017372,-178.254517970998,-1.74137097164627E-11));
#36719=CARTESIAN_POINT('Ctrl Pts',(7.27603390512279,-178.079517970998,-4.20082013377279));
#36720=CARTESIAN_POINT('Ctrl Pts',(4.85068927007185,-177.904517970998,-8.4016402675283));
#36721=CARTESIAN_POINT('Ctrl Pts',(-1.50354276030374E-11,-177.729517970998,
-8.40164026751963));
#36722=CARTESIAN_POINT('Ctrl Pts',(-4.85068927010192,-177.554517970998,
-8.40164026751093));
#36723=CARTESIAN_POINT('Ctrl Pts',(-7.27603390513783,-177.379517970998,
-4.20082013374675));
#36724=CARTESIAN_POINT('Ctrl Pts',(-9.70137854017372,-177.204517970998,
1.73091229795164E-11));
#36725=CARTESIAN_POINT('Ctrl Pts',(-7.27603390512278,-177.029517970998,
4.20082013377282));
#36726=CARTESIAN_POINT('Ctrl Pts',(-4.85068927007182,-176.854517970998,
8.40164026752831));
#36727=CARTESIAN_POINT('Ctrl Pts',(1.50642473211541E-11,-176.679517970998,
8.40164026751963));
#36728=CARTESIAN_POINT('Ctrl Pts',(4.85068927010183,-176.504517970998,8.40164026751099));
#36729=CARTESIAN_POINT('Ctrl Pts',(7.27603390513778,-176.329517970998,4.20082013374683));
#36730=CARTESIAN_POINT('Ctrl Pts',(9.70137854017372,-176.154517970998,-1.73424011235416E-11));
#36731=CARTESIAN_POINT('Ctrl Pts',(7.27603390512277,-175.979517970998,-4.20082013377284));
#36732=CARTESIAN_POINT('Ctrl Pts',(4.85068927007179,-175.804517970998,-8.40164026752833));
#36733=CARTESIAN_POINT('Ctrl Pts',(-1.49736725500596E-11,-175.629517970998,
-8.40164026751963));
#36734=CARTESIAN_POINT('Ctrl Pts',(-4.85068927010185,-175.454517970998,
-8.40164026751097));
#36735=CARTESIAN_POINT('Ctrl Pts',(-7.2760339051378,-175.279517970998,-4.2008201337468));
#36736=CARTESIAN_POINT('Ctrl Pts',(-9.70137854017372,-175.104517970998,
1.73756792675669E-11));
#36737=CARTESIAN_POINT('Ctrl Pts',(-7.27603390512275,-174.929517970998,
4.20082013377287));
#36738=CARTESIAN_POINT('Ctrl Pts',(-4.85068927007188,-174.754517970998,
8.40164026752828));
#36739=CARTESIAN_POINT('Ctrl Pts',(1.50024922681763E-11,-174.579517970998,
8.40164026751963));
#36740=CARTESIAN_POINT('Ctrl Pts',(4.85068927010188,-174.404517970998,8.40164026751095));
#36741=CARTESIAN_POINT('Ctrl Pts',(7.27603390513781,-174.229517970998,4.20082013374678));
#36742=CARTESIAN_POINT('Ctrl Pts',(9.70137854017372,-174.054517970998,-1.74089574115921E-11));
#36743=CARTESIAN_POINT('Ctrl Pts',(7.2760339051228,-173.879517970998,-4.20082013377279));
#36744=CARTESIAN_POINT('Ctrl Pts',(4.85068927007185,-173.704517970998,-8.4016402675283));
#36745=CARTESIAN_POINT('Ctrl Pts',(-1.50313119862929E-11,-173.529517970998,
-8.40164026751963));
#36746=CARTESIAN_POINT('Ctrl Pts',(-4.85068927010191,-173.354517970998,
-8.40164026751094));
#36747=CARTESIAN_POINT('Ctrl Pts',(-7.27603390513777,-173.179517970998,
-4.20082013374686));
#36748=CARTESIAN_POINT('Ctrl Pts',(-9.70137854017372,-173.004517970998,
1.73043706746458E-11));
#36749=CARTESIAN_POINT('Ctrl Pts',(-7.27603390512278,-172.829517970998,
4.20082013377282));
#36750=CARTESIAN_POINT('Ctrl Pts',(-4.85068927007182,-172.654517970998,
8.40164026752831));
#36751=CARTESIAN_POINT('Ctrl Pts',(1.50601317044096E-11,-172.479517970998,
8.40164026751963));
#36752=CARTESIAN_POINT('Ctrl Pts',(4.85068927010182,-172.304517970998,8.40164026751099));
#36753=CARTESIAN_POINT('Ctrl Pts',(7.27603390513778,-172.129517970998,4.20082013374683));
#36754=CARTESIAN_POINT('Ctrl Pts',(9.70137854017372,-171.954517970998,-1.7337648818671E-11));
#36755=CARTESIAN_POINT('Ctrl Pts',(7.27603390512277,-171.779517970998,-4.20082013377284));
#36756=CARTESIAN_POINT('Ctrl Pts',(4.85068927007179,-171.604517970998,-8.40164026752833));
#36757=CARTESIAN_POINT('Ctrl Pts',(-1.49695569333151E-11,-171.429517970998,
-8.40164026751963));
#36758=CARTESIAN_POINT('Ctrl Pts',(-4.85068927010185,-171.254517970998,
-8.40164026751097));
#36759=CARTESIAN_POINT('Ctrl Pts',(-7.2760339051378,-171.079517970998,-4.20082013374681));
#36760=CARTESIAN_POINT('Ctrl Pts',(-9.70137854017372,-170.904517970998,
1.73709269626963E-11));
#36761=CARTESIAN_POINT('Ctrl Pts',(-7.27603390512275,-170.729517970998,
4.20082013377287));
#36762=CARTESIAN_POINT('Ctrl Pts',(-4.85068927007176,-170.554517970998,
8.40164026752834));
#36763=CARTESIAN_POINT('Ctrl Pts',(1.49983766514318E-11,-170.379517970998,
8.40164026751963));
#36764=CARTESIAN_POINT('Ctrl Pts',(4.85068927010176,-170.204517970998,8.40164026751102));
#36765=CARTESIAN_POINT('Ctrl Pts',(7.27603390513781,-170.029517970998,4.20082013374678));
#36766=CARTESIAN_POINT('Ctrl Pts',(9.70137854017372,-169.854517970998,-1.72663402257499E-11));
#36767=CARTESIAN_POINT('Ctrl Pts',(7.27603390512274,-169.679517970998,-4.20082013377289));
#36768=CARTESIAN_POINT('Ctrl Pts',(4.85068927007186,-169.504517970998,-8.40164026752829));
#36769=CARTESIAN_POINT('Ctrl Pts',(-1.49078018803373E-11,-169.329517970998,
-8.40164026751963));
#36770=CARTESIAN_POINT('Ctrl Pts',(-4.85068927010191,-169.154517970998,
-8.40164026751094));
#36771=CARTESIAN_POINT('Ctrl Pts',(-7.27603390513777,-168.979517970998,
-4.20082013374686));
#36772=CARTESIAN_POINT('Ctrl Pts',(-9.70137854017372,-168.804517970998,
1.74374832507468E-11));
#36773=CARTESIAN_POINT('Ctrl Pts',(-7.27603390512278,-168.629517970998,
4.20082013377281));
#36774=CARTESIAN_POINT('Ctrl Pts',(-4.85068927007195,-168.454517970998,
8.40164026752824));
#36775=CARTESIAN_POINT('Ctrl Pts',(1.50560160876651E-11,-168.279517970998,
8.40164026751963));
#36776=CARTESIAN_POINT('Ctrl Pts',(4.85068927010182,-168.104517970998,8.40164026751099));
#36777=CARTESIAN_POINT('Ctrl Pts',(7.27603390513784,-167.929517970998,4.20082013374673));
#36778=CARTESIAN_POINT('Ctrl Pts',(9.70137854017372,-167.754517970998,-1.73328965138004E-11));
#36779=CARTESIAN_POINT('Ctrl Pts',(7.27603390512283,-167.579517970998,-4.20082013377273));
#36780=CARTESIAN_POINT('Ctrl Pts',(4.8506892700718,-167.404517970998,-8.40164026752832));
#36781=CARTESIAN_POINT('Ctrl Pts',(-1.49654413165707E-11,-167.229517970998,
-8.40164026751963));
#36782=CARTESIAN_POINT('Ctrl Pts',(-4.85068927010197,-167.054517970998,
-8.4016402675109));
#36783=CARTESIAN_POINT('Ctrl Pts',(-7.27603390513779,-166.879517970998,
-4.20082013374681));
#36784=CARTESIAN_POINT('Ctrl Pts',(-9.70137854017372,-166.704517970998,
1.72283097768541E-11));
#36785=CARTESIAN_POINT('Ctrl Pts',(-7.27603390512276,-166.529517970998,
4.20082013377286));
#36786=CARTESIAN_POINT('Ctrl Pts',(-4.85068927007189,-166.354517970998,
8.40164026752827));
#36787=CARTESIAN_POINT('Ctrl Pts',(1.51136555238984E-11,-166.179517970998,
8.40164026751963));
#36788=CARTESIAN_POINT('Ctrl Pts',(4.85068927010188,-166.004517970998,8.40164026751096));
#36789=CARTESIAN_POINT('Ctrl Pts',(7.27603390513775,-165.829517970998,4.20082013374689));
#36790=CARTESIAN_POINT('Ctrl Pts',(9.70137854017372,-165.654517970998,-1.73994528018509E-11));
#36791=CARTESIAN_POINT('Ctrl Pts',(7.2760339051228,-165.479517970998,-4.20082013377278));
#36792=CARTESIAN_POINT('Ctrl Pts',(4.85068927007198,-165.304517970998,-8.40164026752822));
#36793=CARTESIAN_POINT('Ctrl Pts',(-1.5023080752804E-11,-165.129517970998,
-8.40164026751963));
#36794=CARTESIAN_POINT('Ctrl Pts',(-4.85068927010179,-164.954517970998,
-8.40164026751101));
#36795=CARTESIAN_POINT('Ctrl Pts',(-7.27603390513782,-164.779517970998,
-4.20082013374676));
#36796=CARTESIAN_POINT('Ctrl Pts',(-9.70137854017372,-164.604517970998,
1.72948660649045E-11));
#36797=CARTESIAN_POINT('Ctrl Pts',(-7.27603390512285,-164.429517970998,
4.20082013377271));
#36798=CARTESIAN_POINT('Ctrl Pts',(-4.85068927007183,-164.254517970998,
8.40164026752831));
#36799=CARTESIAN_POINT('Ctrl Pts',(1.49325059817095E-11,-164.079517970998,
8.40164026751963));
#36800=CARTESIAN_POINT('Ctrl Pts',(4.85068927010193,-163.904517970998,8.40164026751092));
#36801=CARTESIAN_POINT('Ctrl Pts',(7.27603390513778,-163.729517970998,4.20082013374684));
#36802=CARTESIAN_POINT('Ctrl Pts',(9.70137854017372,-163.554517970998,-1.71902793279582E-11));
#36803=CARTESIAN_POINT('Ctrl Pts',(7.27603390512277,-163.379517970998,-4.20082013377283));
#36804=CARTESIAN_POINT('Ctrl Pts',(4.85068927007192,-163.204517970998,-8.40164026752825));
#36805=CARTESIAN_POINT('Ctrl Pts',(-1.50807201890373E-11,-163.029517970998,
-8.40164026751963));
#36806=CARTESIAN_POINT('Ctrl Pts',(-4.85068927010184,-162.854517970998,
-8.40164026751098));
#36807=CARTESIAN_POINT('Ctrl Pts',(-7.27603390513773,-162.679517970998,
-4.20082013374692));
#36808=CARTESIAN_POINT('Ctrl Pts',(-9.70137854017372,-162.504517970998,
1.7361422352955E-11));
#36809=CARTESIAN_POINT('Ctrl Pts',(-7.27603390512282,-162.329517970998,
4.20082013377275));
#36810=CARTESIAN_POINT('Ctrl Pts',(-4.85068927007177,-162.154517970998,
8.40164026752834));
#36811=CARTESIAN_POINT('Ctrl Pts',(1.49901454179428E-11,-161.979517970998,
8.40164026751963));
#36812=CARTESIAN_POINT('Ctrl Pts',(4.85068927010175,-161.804517970998,8.40164026751103));
#36813=CARTESIAN_POINT('Ctrl Pts',(7.27603390513781,-161.629517970998,4.20082013374679));
#36814=CARTESIAN_POINT('Ctrl Pts',(9.70137854017372,-161.454517970998,-1.72568356160087E-11));
#36815=CARTESIAN_POINT('Ctrl Pts',(7.27603390512274,-161.279517970998,-4.20082013377288));
#36816=CARTESIAN_POINT('Ctrl Pts',(4.85068927007186,-161.104517970998,-8.40164026752829));
#36817=CARTESIAN_POINT('Ctrl Pts',(-1.48995706468484E-11,-160.929517970998,
-8.40164026751963));
#36818=CARTESIAN_POINT('Ctrl Pts',(-4.8506892701019,-160.754517970998,-8.40164026751094));
#36819=CARTESIAN_POINT('Ctrl Pts',(-7.27603390513776,-160.579517970998,
-4.20082013374687));
#36820=CARTESIAN_POINT('Ctrl Pts',(-9.70137854017372,-160.404517970998,
1.74279786410055E-11));
#36821=CARTESIAN_POINT('Ctrl Pts',(-7.27603390512279,-160.229517970998,
4.2008201337728));
#36822=CARTESIAN_POINT('Ctrl Pts',(-4.85068927007195,-160.054517970998,
8.40164026752823));
#36823=CARTESIAN_POINT('Ctrl Pts',(1.50477848541761E-11,-159.879517970998,
8.40164026751963));
#36824=CARTESIAN_POINT('Ctrl Pts',(4.85068927010181,-159.704517970998,8.401640267511));
#36825=CARTESIAN_POINT('Ctrl Pts',(7.27603390513784,-159.529517970998,4.20082013374674));
#36826=CARTESIAN_POINT('Ctrl Pts',(9.70137854017372,-159.354517970998,-1.73233919040592E-11));
#36827=CARTESIAN_POINT('Ctrl Pts',(7.27603390512283,-159.179517970998,-4.20082013377273));
#36828=CARTESIAN_POINT('Ctrl Pts',(4.8506892700718,-159.004517970998,-8.40164026752832));
#36829=CARTESIAN_POINT('Ctrl Pts',(-1.49572100830817E-11,-158.829517970998,
-8.40164026751963));
#36830=CARTESIAN_POINT('Ctrl Pts',(-4.85068927010172,-158.654517970998,
-8.40164026751105));
#36831=CARTESIAN_POINT('Ctrl Pts',(-7.27603390513779,-158.479517970998,
-4.20082013374682));
#36832=CARTESIAN_POINT('Ctrl Pts',(-9.70137854017372,-158.304517970998,
1.72188051671128E-11));
#36833=CARTESIAN_POINT('Ctrl Pts',(-7.27603390512276,-158.129517970998,
4.20082013377285));
#36834=CARTESIAN_POINT('Ctrl Pts',(-4.8506892700719,-157.954517970998,8.40164026752827));
#36835=CARTESIAN_POINT('Ctrl Pts',(1.48666353119872E-11,-157.779517970998,
8.40164026751963));
#36836=CARTESIAN_POINT('Ctrl Pts',(4.85068927010187,-157.604517970998,8.40164026751096));
#36837=CARTESIAN_POINT('Ctrl Pts',(7.27603390513774,-157.429517970998,4.2008201337469));
#36838=CARTESIAN_POINT('Ctrl Pts',(9.70137854017372,-157.254517970998,-1.73899481921097E-11));
#36839=CARTESIAN_POINT('Ctrl Pts',(7.27603390512281,-157.079517970998,-4.20082013377278));
#36840=CARTESIAN_POINT('Ctrl Pts',(4.85068927007199,-156.904517970998,-8.40164026752822));
#36841=CARTESIAN_POINT('Ctrl Pts',(-1.5014849519315E-11,-156.729517970998,
-8.40164026751963));
#36842=CARTESIAN_POINT('Ctrl Pts',(-4.85068927010178,-156.554517970998,
-8.40164026751101));
#36843=CARTESIAN_POINT('Ctrl Pts',(-7.27603390513782,-156.379517970998,
-4.20082013374677));
#36844=CARTESIAN_POINT('Ctrl Pts',(-9.70137854017372,-156.204517970998,
1.72853614551633E-11));
#36845=CARTESIAN_POINT('Ctrl Pts',(-7.27603390512285,-156.029517970998,
4.2008201337727));
#36846=CARTESIAN_POINT('Ctrl Pts',(-4.85068927007184,-155.854517970998,
8.4016402675283));
#36847=CARTESIAN_POINT('Ctrl Pts',(1.49242747482206E-11,-155.679517970998,
8.40164026751963));
#36848=CARTESIAN_POINT('Ctrl Pts',(4.85068927010193,-155.504517970998,8.40164026751093));
#36849=CARTESIAN_POINT('Ctrl Pts',(7.27603390513778,-155.329517970998,4.20082013374685));
#36850=CARTESIAN_POINT('Ctrl Pts',(9.70137854017372,-155.154517970998,-1.7180774718217E-11));
#36851=CARTESIAN_POINT('Ctrl Pts',(7.27603390512277,-154.979517970998,-4.20082013377283));
#36852=CARTESIAN_POINT('Ctrl Pts',(4.85068927007193,-154.804517970998,-8.40164026752825));
#36853=CARTESIAN_POINT('Ctrl Pts',(-1.50724889555483E-11,-154.629517970998,
-8.40164026751963));
#36854=CARTESIAN_POINT('Ctrl Pts',(-4.85068927010184,-154.454517970998,
-8.40164026751098));
#36855=CARTESIAN_POINT('Ctrl Pts',(-7.27603390513773,-154.279517970998,
-4.20082013374692));
#36856=CARTESIAN_POINT('Ctrl Pts',(-9.70137854017372,-154.104517970998,
1.73519177432138E-11));
#36857=CARTESIAN_POINT('Ctrl Pts',(-7.27603390512282,-153.929517970998,
4.20082013377275));
#36858=CARTESIAN_POINT('Ctrl Pts',(-4.85068927007178,-153.754517970998,
8.40164026752833));
#36859=CARTESIAN_POINT('Ctrl Pts',(1.49819141844539E-11,-153.579517970998,
8.40164026751963));
#36860=CARTESIAN_POINT('Ctrl Pts',(4.85068927010175,-153.404517970998,8.40164026751103));
#36861=CARTESIAN_POINT('Ctrl Pts',(7.2760339051378,-153.229517970998,4.2008201337468));
#36862=CARTESIAN_POINT('Ctrl Pts',(9.70137854017372,-153.054517970998,-1.72473310062675E-11));
#36863=CARTESIAN_POINT('Ctrl Pts',(7.27603390512275,-152.879517970998,-4.20082013377288));
#36864=CARTESIAN_POINT('Ctrl Pts',(4.85068927007187,-152.704517970998,-8.40164026752828));
#36865=CARTESIAN_POINT('Ctrl Pts',(-1.48913394133594E-11,-152.529517970998,
-8.40164026751963));
#36866=CARTESIAN_POINT('Ctrl Pts',(-4.85068927010189,-152.354517970998,
-8.40164026751095));
#36867=CARTESIAN_POINT('Ctrl Pts',(-7.27603390513776,-152.179517970998,
-4.20082013374688));
#36868=CARTESIAN_POINT('Ctrl Pts',(-9.70137854017372,-152.004517970998,
1.71427442693211E-11));
#36869=CARTESIAN_POINT('Ctrl Pts',(-7.27603390512279,-151.829517970998,
4.2008201337728));
#36870=CARTESIAN_POINT('Ctrl Pts',(-4.85068927007196,-151.654517970998,
8.40164026752823));
#36871=CARTESIAN_POINT('Ctrl Pts',(1.50395536206872E-11,-151.479517970998,
8.40164026751963));
#36872=CARTESIAN_POINT('Ctrl Pts',(4.8506892701018,-151.304517970998,8.401640267511));
#36873=CARTESIAN_POINT('Ctrl Pts',(7.27603390513771,-151.129517970998,4.20082013374695));
#36874=CARTESIAN_POINT('Ctrl Pts',(9.70137854017372,-150.954517970998,-1.73138872943179E-11));
#36875=CARTESIAN_POINT('Ctrl Pts',(7.27603390512284,-150.779517970998,-4.20082013377272));
#36876=CARTESIAN_POINT('Ctrl Pts',(4.85068927007181,-150.604517970998,-8.40164026752832));
#36877=CARTESIAN_POINT('Ctrl Pts',(-1.49489788495927E-11,-150.429517970998,
-8.40164026751963));
#36878=CARTESIAN_POINT('Ctrl Pts',(-4.85068927010171,-150.254517970998,
-8.40164026751105));
#36879=CARTESIAN_POINT('Ctrl Pts',(-7.27603390513779,-150.079517970998,
-4.20082013374683));
#36880=CARTESIAN_POINT('Ctrl Pts',(-9.70137854017372,-149.904517970998,
1.72093005573716E-11));
#36881=CARTESIAN_POINT('Ctrl Pts',(-7.27603390512276,-149.729517970998,
4.20082013377285));
#36882=CARTESIAN_POINT('Ctrl Pts',(-4.8506892700719,-149.554517970998,8.40164026752826));
#36883=CARTESIAN_POINT('Ctrl Pts',(1.48584040784983E-11,-149.379517970998,
8.40164026751963));
#36884=CARTESIAN_POINT('Ctrl Pts',(4.85068927010186,-149.204517970998,8.40164026751097));
#36885=CARTESIAN_POINT('Ctrl Pts',(7.27603390513774,-149.029517970998,4.2008201337469));
#36886=CARTESIAN_POINT('Ctrl Pts',(9.70137854017372,-148.854517970998,-1.73804435823684E-11));
#36887=CARTESIAN_POINT('Ctrl Pts',(7.27603390512281,-148.679517970998,-4.20082013377277));
#36888=CARTESIAN_POINT('Ctrl Pts',(4.85068927007199,-148.504517970998,-8.40164026752821));
#36889=CARTESIAN_POINT('Ctrl Pts',(-1.5006618285826E-11,-148.329517970998,
-8.40164026751963));
#36890=CARTESIAN_POINT('Ctrl Pts',(-4.85068927010177,-148.154517970998,
-8.40164026751102));
#36891=CARTESIAN_POINT('Ctrl Pts',(-7.27603390513782,-147.979517970998,
-4.20082013374678));
#36892=CARTESIAN_POINT('Ctrl Pts',(-9.70137854017372,-147.804517970998,
1.72758568454221E-11));
#36893=CARTESIAN_POINT('Ctrl Pts',(-7.27603390512285,-147.629517970998,
4.20082013377269));
#36894=CARTESIAN_POINT('Ctrl Pts',(-4.85068927007185,-147.454517970998,
8.4016402675283));
#36895=CARTESIAN_POINT('Ctrl Pts',(1.49160435147316E-11,-147.279517970998,
8.40164026751963));
#36896=CARTESIAN_POINT('Ctrl Pts',(4.85068927010192,-147.104517970998,8.40164026751093));
#36897=CARTESIAN_POINT('Ctrl Pts',(7.27603390513777,-146.929517970998,4.20082013374685));
#36898=CARTESIAN_POINT('Ctrl Pts',(9.70137854017372,-146.754517970998,-1.71712701084757E-11));
#36899=CARTESIAN_POINT('Ctrl Pts',(7.27603390512278,-146.579517970998,-4.20082013377282));
#36900=CARTESIAN_POINT('Ctrl Pts',(4.85068927007194,-146.404517970998,-8.40164026752825));
#36901=CARTESIAN_POINT('Ctrl Pts',(-1.50642577220594E-11,-146.229517970998,
-8.40164026751963));
#36902=CARTESIAN_POINT('Ctrl Pts',(-4.85068927010183,-146.054517970998,
-8.40164026751099));
#36903=CARTESIAN_POINT('Ctrl Pts',(-7.27603390513773,-145.879517970998,
-4.20082013374693));
#36904=CARTESIAN_POINT('Ctrl Pts',(-9.70137854017372,-145.704517970998,
1.73424131334726E-11));
#36905=CARTESIAN_POINT('Ctrl Pts',(-7.27603390512282,-145.529517970998,
4.20082013377274));
#36906=CARTESIAN_POINT('Ctrl Pts',(-4.85068927007203,-145.354517970998,
8.40164026752819));
#36907=CARTESIAN_POINT('Ctrl Pts',(1.49736829509649E-11,-145.179517970998,
8.40164026751963));
#36908=CARTESIAN_POINT('Ctrl Pts',(4.85068927010174,-145.004517970998,8.40164026751104));
#36909=CARTESIAN_POINT('Ctrl Pts',(7.2760339051378,-144.829517970998,4.2008201337468));
#36910=CARTESIAN_POINT('Ctrl Pts',(9.70137854017372,-144.654517970998,-1.72378263965262E-11));
#36911=CARTESIAN_POINT('Ctrl Pts',(7.27603390512287,-144.479517970998,-4.20082013377266));
#36912=CARTESIAN_POINT('Ctrl Pts',(4.85068927007188,-144.304517970998,-8.40164026752828));
#36913=CARTESIAN_POINT('Ctrl Pts',(-1.48831081798705E-11,-144.129517970998,
-8.40164026751963));
#36914=CARTESIAN_POINT('Ctrl Pts',(-4.85068927010188,-143.954517970998,
-8.40164026751095));
#36915=CARTESIAN_POINT('Ctrl Pts',(-7.27603390513775,-143.779517970998,
-4.20082013374688));
#36916=CARTESIAN_POINT('Ctrl Pts',(-9.70137854017372,-143.604517970998,
1.71332396595799E-11));
#36917=CARTESIAN_POINT('Ctrl Pts',(-7.2760339051228,-143.429517970998,4.20082013377279));
#36918=CARTESIAN_POINT('Ctrl Pts',(-4.85068927007197,-143.254517970998,
8.40164026752823));
#36919=CARTESIAN_POINT('Ctrl Pts',(1.50313223871982E-11,-143.079517970998,
8.40164026751963));
#36920=CARTESIAN_POINT('Ctrl Pts',(4.85068927010179,-142.904517970998,8.401640267511));
#36921=CARTESIAN_POINT('Ctrl Pts',(7.27603390513771,-142.729517970998,4.20082013374696));
#36922=CARTESIAN_POINT('Ctrl Pts',(9.70137854017372,-142.554517970998,-1.73043826845767E-11));
#36923=CARTESIAN_POINT('Ctrl Pts',(7.27603390512284,-142.379517970998,-4.20082013377271));
#36924=CARTESIAN_POINT('Ctrl Pts',(4.85068927007182,-142.204517970998,-8.40164026752831));
#36925=CARTESIAN_POINT('Ctrl Pts',(-1.49407476161038E-11,-142.029517970998,
-8.40164026751963));
#36926=CARTESIAN_POINT('Ctrl Pts',(-4.8506892701017,-141.854517970998,-8.40164026751106));
#36927=CARTESIAN_POINT('Ctrl Pts',(-7.27603390513778,-141.679517970998,
-4.20082013374683));
#36928=CARTESIAN_POINT('Ctrl Pts',(-9.70137854017372,-141.504517970998,
1.71997959476304E-11));
#36929=CARTESIAN_POINT('Ctrl Pts',(-7.27603390512277,-141.329517970998,
4.20082013377284));
#36930=CARTESIAN_POINT('Ctrl Pts',(-4.85068927007191,-141.154517970998,
8.40164026752826));
#36931=CARTESIAN_POINT('Ctrl Pts',(1.48501728450093E-11,-140.979517970998,
8.40164026751963));
#36932=CARTESIAN_POINT('Ctrl Pts',(4.85068927010185,-140.804517970998,8.40164026751097));
#36933=CARTESIAN_POINT('Ctrl Pts',(7.27603390513774,-140.629517970998,4.20082013374691));
#36934=CARTESIAN_POINT('Ctrl Pts',(9.70137854017372,-140.454517970998,-1.73709389726272E-11));
#36935=CARTESIAN_POINT('Ctrl Pts',(7.27603390512281,-140.279517970998,-4.20082013377276));
#36936=CARTESIAN_POINT('Ctrl Pts',(4.850689270072,-140.104517970998,-8.40164026752821));
#36937=CARTESIAN_POINT('Ctrl Pts',(-1.49983870523371E-11,-139.929517970998,
-8.40164026751963));
#36938=CARTESIAN_POINT('Ctrl Pts',(-4.85068927010176,-139.754517970998,
-8.40164026751102));
#36939=CARTESIAN_POINT('Ctrl Pts',(-7.27603390513769,-139.579517970998,
-4.20082013374699));
#36940=CARTESIAN_POINT('Ctrl Pts',(-9.70137854017372,-139.404517970998,
1.72663522356809E-11));
#36941=CARTESIAN_POINT('Ctrl Pts',(-7.27603390512286,-139.229517970998,
4.20082013377268));
#36942=CARTESIAN_POINT('Ctrl Pts',(-4.85068927007186,-139.054517970998,
8.40164026752829));
#36943=CARTESIAN_POINT('Ctrl Pts',(1.49078122812426E-11,-138.879517970998,
8.40164026751963));
#36944=CARTESIAN_POINT('Ctrl Pts',(4.85068927010167,-138.704517970998,8.40164026751108));
#36945=CARTESIAN_POINT('Ctrl Pts',(7.27603390513777,-138.529517970998,4.20082013374686));
#36946=CARTESIAN_POINT('Ctrl Pts',(9.70137854017372,-138.354517970998,-1.71617654987345E-11));
#36947=CARTESIAN_POINT('Ctrl Pts',(7.27603390512278,-138.179517970998,-4.20082013377281));
#36948=CARTESIAN_POINT('Ctrl Pts',(4.85068927007195,-138.004517970998,-8.40164026752824));
#36949=CARTESIAN_POINT('Ctrl Pts',(-1.48172375101482E-11,-137.829517970998,
-8.40164026751963));
#36950=CARTESIAN_POINT('Ctrl Pts',(-4.85068927010182,-137.654517970998,
-8.40164026751099));
#36951=CARTESIAN_POINT('Ctrl Pts',(-7.27603390513772,-137.479517970998,
-4.20082013374694));
#36952=CARTESIAN_POINT('Ctrl Pts',(-9.70137854017372,-137.304517970998,
1.73329085237313E-11));
#36953=CARTESIAN_POINT('Ctrl Pts',(-7.27603390512283,-137.129517970998,
4.20082013377273));
#36954=CARTESIAN_POINT('Ctrl Pts',(-4.85068927007204,-136.954517970998,
8.40164026752819));
#36955=CARTESIAN_POINT('Ctrl Pts',(1.49654517174759E-11,-136.779517970998,
8.40164026751963));
#36956=CARTESIAN_POINT('Ctrl Pts',(4.85068927010173,-136.604517970998,8.40164026751104));
#36957=CARTESIAN_POINT('Ctrl Pts',(7.27603390513779,-136.429517970998,4.20082013374681));
#36958=CARTESIAN_POINT('Ctrl Pts',(9.70137854017372,-136.254517970999,-1.7228321786785E-11));
#36959=CARTESIAN_POINT('Ctrl Pts',(7.27603390512287,-136.079517970998,-4.20082013377265));
#36960=CARTESIAN_POINT('Ctrl Pts',(4.85068927007189,-135.904517970998,-8.40164026752827));
#36961=CARTESIAN_POINT('Ctrl Pts',(-1.48748769463815E-11,-135.729517970998,
-8.40164026751963));
#36962=CARTESIAN_POINT('Ctrl Pts',(-4.85068927010188,-135.554517970998,
-8.40164026751096));
#36963=CARTESIAN_POINT('Ctrl Pts',(-7.27603390513775,-135.379517970998,
-4.20082013374689));
#36964=CARTESIAN_POINT('Ctrl Pts',(-9.70137854017372,-135.204517970998,
1.71237350498386E-11));
#36965=CARTESIAN_POINT('Ctrl Pts',(-7.2760339051228,-135.029517970998,4.20082013377278));
#36966=CARTESIAN_POINT('Ctrl Pts',(-4.85068927007198,-134.854517970998,
8.40164026752822));
#36967=CARTESIAN_POINT('Ctrl Pts',(1.50230911537093E-11,-134.679517970998,
8.40164026751963));
#36968=CARTESIAN_POINT('Ctrl Pts',(4.85068927010179,-134.504517970998,8.40164026751101));
#36969=CARTESIAN_POINT('Ctrl Pts',(7.2760339051377,-134.329517970998,4.20082013374697));
#36970=CARTESIAN_POINT('Ctrl Pts',(9.70137854017372,-134.154517970998,-1.72948780748355E-11));
#36971=CARTESIAN_POINT('Ctrl Pts',(7.27603390512285,-133.979517970998,-4.20082013377271));
#36972=CARTESIAN_POINT('Ctrl Pts',(4.85068927007183,-133.804517970998,-8.40164026752831));
#36973=CARTESIAN_POINT('Ctrl Pts',(-1.49325163826148E-11,-133.629517970998,
-8.40164026751963));
#36974=CARTESIAN_POINT('Ctrl Pts',(-4.85068927010169,-133.454517970998,
-8.40164026751106));
#36975=CARTESIAN_POINT('Ctrl Pts',(-7.27603390513778,-133.279517970998,
-4.20082013374684));
#36976=CARTESIAN_POINT('Ctrl Pts',(-9.70137854017372,-133.104517970998,
1.71902913378891E-11));
#36977=CARTESIAN_POINT('Ctrl Pts',(-7.27603390512289,-132.929517970998,
4.20082013377263));
#36978=CARTESIAN_POINT('Ctrl Pts',(-4.85068927007192,-132.754517970998,
8.40164026752825));
#36979=CARTESIAN_POINT('Ctrl Pts',(1.48419416115203E-11,-132.579517970998,
8.40164026751963));
#36980=CARTESIAN_POINT('Ctrl Pts',(4.85068927010184,-132.404517970998,8.40164026751098));
#36981=CARTESIAN_POINT('Ctrl Pts',(7.27603390513773,-132.229517970998,4.20082013374692));
#36982=CARTESIAN_POINT('Ctrl Pts',(9.70137854017372,-132.054517970998,-1.70857046009428E-11));
#36983=CARTESIAN_POINT('Ctrl Pts',(7.27603390512282,-131.879517970998,-4.20082013377275));
#36984=CARTESIAN_POINT('Ctrl Pts',(4.85068927007201,-131.704517970998,-8.4016402675282));
#36985=CARTESIAN_POINT('Ctrl Pts',(-1.49901558188481E-11,-131.529517970998,
-8.40164026751963));
#36986=CARTESIAN_POINT('Ctrl Pts',(-4.85068927010175,-131.354517970998,
-8.40164026751103));
#36987=CARTESIAN_POINT('Ctrl Pts',(-7.27603390513769,-131.179517970998,
-4.200820133747));
#36988=CARTESIAN_POINT('Ctrl Pts',(-9.70137854017372,-131.004517970998,
1.72568476259396E-11));
#36989=CARTESIAN_POINT('Ctrl Pts',(-7.27603390512286,-130.829517970998,
4.20082013377267));
#36990=CARTESIAN_POINT('Ctrl Pts',(-4.85068927007186,-130.654517970998,
8.40164026752829));
#36991=CARTESIAN_POINT('Ctrl Pts',(1.48995810477537E-11,-130.479517970998,
8.40164026751963));
#36992=CARTESIAN_POINT('Ctrl Pts',(4.85068927010166,-130.304517970998,8.40164026751108));
#36993=CARTESIAN_POINT('Ctrl Pts',(7.27603390513776,-130.129517970998,4.20082013374687));
#36994=CARTESIAN_POINT('Ctrl Pts',(9.70137854017372,-129.954517970998,-1.71522608889933E-11));
#36995=CARTESIAN_POINT('Ctrl Pts',(7.27603390512279,-129.779517970998,-4.2008201337728));
#36996=CARTESIAN_POINT('Ctrl Pts',(4.85068927007195,-129.604517970998,-8.40164026752823));
#36997=CARTESIAN_POINT('Ctrl Pts',(-1.48090062766592E-11,-129.429517970998,
-8.40164026751963));
#36998=CARTESIAN_POINT('Ctrl Pts',(-4.85068927010181,-129.254517970998,
-8.401640267511));
#36999=CARTESIAN_POINT('Ctrl Pts',(-7.27603390513772,-129.079517970998,
-4.20082013374695));
#37000=CARTESIAN_POINT('Ctrl Pts',(-9.70137854017372,-128.904517970998,
1.73234039139901E-11));
#37001=CARTESIAN_POINT('Ctrl Pts',(-7.27603390512283,-128.729517970998,
4.20082013377273));
#37002=CARTESIAN_POINT('Ctrl Pts',(-4.85068927007204,-128.554517970998,
8.40164026752818));
#37003=CARTESIAN_POINT('Ctrl Pts',(1.4957220483987E-11,-128.379517970998,
8.40164026751963));
#37004=CARTESIAN_POINT('Ctrl Pts',(4.85068927010172,-128.204517970998,8.40164026751105));
#37005=CARTESIAN_POINT('Ctrl Pts',(7.27603390513779,-128.029517970998,4.20082013374682));
#37006=CARTESIAN_POINT('Ctrl Pts',(9.70137854017372,-127.854517970998,-1.72188171770438E-11));
#37007=CARTESIAN_POINT('Ctrl Pts',(7.27603390512276,-127.679517970998,-4.20082013377285));
#37008=CARTESIAN_POINT('Ctrl Pts',(4.85068927007213,-127.504517970998,-8.40164026752813));
#37009=CARTESIAN_POINT('Ctrl Pts',(-1.48666457128925E-11,-127.329517970998,
-8.40164026751963));
#37010=CARTESIAN_POINT('Ctrl Pts',(-4.85068927010187,-127.154517970998,
-8.40164026751096));
#37011=CARTESIAN_POINT('Ctrl Pts',(-7.27603390513763,-126.979517970998,
-4.2008201337471));
#37012=CARTESIAN_POINT('Ctrl Pts',(-9.70137854017372,-126.804517970998,
1.71142304400974E-11));
#37013=CARTESIAN_POINT('Ctrl Pts',(-7.27603390512281,-126.629517970998,
4.20082013377278));
#37014=CARTESIAN_POINT('Ctrl Pts',(-4.85068927007175,-126.454517970998,
8.40164026752835));
#37015=CARTESIAN_POINT('Ctrl Pts',(1.47760709417981E-11,-126.279517970998,
8.40164026751963));
#37016=CARTESIAN_POINT('Ctrl Pts',(4.85068927010178,-126.104517970998,8.40164026751101));
#37017=CARTESIAN_POINT('Ctrl Pts',(7.27603390513782,-125.929517970998,4.20082013374677));
#37018=CARTESIAN_POINT('Ctrl Pts',(9.70137854017372,-125.754517970998,-1.70096437031511E-11));
#37019=CARTESIAN_POINT('Ctrl Pts',(7.27603390512285,-125.579517970998,-4.2008201337727));
#37020=CARTESIAN_POINT('Ctrl Pts',(4.85068927007184,-125.404517970998,-8.4016402675283));
#37021=CARTESIAN_POINT('Ctrl Pts',(-1.46854961707036E-11,-125.229517970998,
-8.40164026751963));
#37022=CARTESIAN_POINT('Ctrl Pts',(-4.85068927010169,-125.054517970998,
-8.40164026751107));
#37023=CARTESIAN_POINT('Ctrl Pts',(-7.27603390513778,-124.879517970998,
-4.20082013374685));
#37024=CARTESIAN_POINT('Ctrl Pts',(-9.70137854017372,-124.704517970998,
1.74565164900911E-11));
#37025=CARTESIAN_POINT('Ctrl Pts',(-7.27603390512289,-124.529517970998,
4.20082013377262));
#37026=CARTESIAN_POINT('Ctrl Pts',(-4.85068927007193,-124.354517970998,
8.40164026752825));
#37027=CARTESIAN_POINT('Ctrl Pts',(1.50724993564536E-11,-124.179517970998,
8.40164026751963));
#37028=CARTESIAN_POINT('Ctrl Pts',(4.8506892701016,-124.004517970998,8.40164026751112));
#37029=CARTESIAN_POINT('Ctrl Pts',(7.27603390513773,-123.829517970998,4.20082013374692));
#37030=CARTESIAN_POINT('Ctrl Pts',(9.70137854017372,-123.654517970998,-1.73519297531447E-11));
#37031=CARTESIAN_POINT('Ctrl Pts',(7.27603390512294,-123.479517970998,-4.20082013377254));
#37032=CARTESIAN_POINT('Ctrl Pts',(4.85068927007202,-123.304517970998,-8.4016402675282));
#37033=CARTESIAN_POINT('Ctrl Pts',(-1.49819245853592E-11,-123.129517970998,
-8.40164026751963));
#37034=CARTESIAN_POINT('Ctrl Pts',(-4.85068927010151,-122.954517970998,
-8.40164026751117));
#37035=CARTESIAN_POINT('Ctrl Pts',(-7.27603390513768,-122.779517970998,
-4.200820133747));
#37036=CARTESIAN_POINT('Ctrl Pts',(-9.70137854017372,-122.604517970998,
1.72473430161984E-11));
#37037=CARTESIAN_POINT('Ctrl Pts',(-7.27603390512275,-122.429517970998,
4.20082013377288));
#37038=CARTESIAN_POINT('Ctrl Pts',(-4.85068927007211,-122.254517970998,
8.40164026752814));
#37039=CARTESIAN_POINT('Ctrl Pts',(1.48913498142647E-11,-122.079517970998,
8.40164026751963));
#37040=CARTESIAN_POINT('Ctrl Pts',(4.85068927010189,-121.904517970998,8.40164026751095));
#37041=CARTESIAN_POINT('Ctrl Pts',(7.27603390513764,-121.729517970998,4.20082013374708));
#37042=CARTESIAN_POINT('Ctrl Pts',(9.70137854017372,-121.554517970999,-1.7142756279252E-11));
#37043=CARTESIAN_POINT('Ctrl Pts',(7.27603390512279,-121.379517970998,-4.2008201337728));
#37044=CARTESIAN_POINT('Ctrl Pts',(4.8506892700722,-121.204517970998,-8.40164026752809));
#37045=CARTESIAN_POINT('Ctrl Pts',(-1.48007750431702E-11,-121.029517970998,
-8.40164026751963));
#37046=CARTESIAN_POINT('Ctrl Pts',(-4.8506892701018,-120.854517970999,-8.401640267511));
#37047=CARTESIAN_POINT('Ctrl Pts',(-7.27603390513783,-120.679517970999,
-4.20082013374675));
#37048=CARTESIAN_POINT('Ctrl Pts',(-9.70137854017372,-120.504517970999,
1.70381695423057E-11));
#37049=CARTESIAN_POINT('Ctrl Pts',(-7.27603390512284,-120.329517970998,
4.20082013377272));
#37050=CARTESIAN_POINT('Ctrl Pts',(-4.85068927007181,-120.154517970998,
8.40164026752832));
#37051=CARTESIAN_POINT('Ctrl Pts',(1.47102002720758E-11,-119.979517970999,
8.40164026751963));
#37052=CARTESIAN_POINT('Ctrl Pts',(4.85068927010171,-119.804517970999,8.40164026751105));
#37053=CARTESIAN_POINT('Ctrl Pts',(7.27603390513779,-119.629517970998,4.20082013374683));
#37054=CARTESIAN_POINT('Ctrl Pts',(9.70137854017372,-119.454517970998,-1.69335828053594E-11));
#37055=CARTESIAN_POINT('Ctrl Pts',(7.27603390512288,-119.279517970999,-4.20082013377264));
#37056=CARTESIAN_POINT('Ctrl Pts',(4.8506892700719,-119.104517970999,-8.40164026752826));
#37057=CARTESIAN_POINT('Ctrl Pts',(-1.50972034578258E-11,-118.929517970998,
-8.40164026751963));
#37058=CARTESIAN_POINT('Ctrl Pts',(-4.85068927010162,-118.754517970998,
-8.40164026751111));
#37059=CARTESIAN_POINT('Ctrl Pts',(-7.27603390513774,-118.579517970998,
-4.2008201337469));
#37060=CARTESIAN_POINT('Ctrl Pts',(-9.70137854017372,-118.404517970999,
1.73804555922994E-11));
#37061=CARTESIAN_POINT('Ctrl Pts',(-7.27603390512293,-118.229517970998,
4.20082013377256));
#37062=CARTESIAN_POINT('Ctrl Pts',(-4.85068927007199,-118.054517970998,
8.40164026752821));
#37063=CARTESIAN_POINT('Ctrl Pts',(1.50066286867313E-11,-117.879517970999,
8.40164026751963));
#37064=CARTESIAN_POINT('Ctrl Pts',(4.85068927010153,-117.704517970998,8.40164026751116));
#37065=CARTESIAN_POINT('Ctrl Pts',(7.2760339051377,-117.529517970998,4.20082013374698));
#37066=CARTESIAN_POINT('Ctrl Pts',(9.70137854017372,-117.354517970999,-1.7275868855353E-11));
#37067=CARTESIAN_POINT('Ctrl Pts',(7.27603390512297,-117.179517970999,-4.20082013377248));
#37068=CARTESIAN_POINT('Ctrl Pts',(4.85068927007208,-117.004517970999,-8.40164026752816));
#37069=CARTESIAN_POINT('Ctrl Pts',(-1.49160539156369E-11,-116.829517970998,
-8.40164026751963));
#37070=CARTESIAN_POINT('Ctrl Pts',(-4.85068927010192,-116.654517970998,
-8.40164026751093));
#37071=CARTESIAN_POINT('Ctrl Pts',(-7.27603390513765,-116.479517970999,
-4.20082013374706));
#37072=CARTESIAN_POINT('Ctrl Pts',(-9.70137854017372,-116.304517970999,
1.71712821184067E-11));
#37073=CARTESIAN_POINT('Ctrl Pts',(-7.27603390512278,-116.129517970999,
4.20082013377282));
#37074=CARTESIAN_POINT('Ctrl Pts',(-4.85068927007218,-115.954517970998,
8.40164026752811));
#37075=CARTESIAN_POINT('Ctrl Pts',(1.48254791445424E-11,-115.779517970998,
8.40164026751963));
#37076=CARTESIAN_POINT('Ctrl Pts',(4.85068927010183,-115.604517970999,8.40164026751099));
#37077=CARTESIAN_POINT('Ctrl Pts',(7.27603390513761,-115.429517970999,4.20082013374714));
#37078=CARTESIAN_POINT('Ctrl Pts',(9.70137854017372,-115.254517970999,-1.70666953814603E-11));
#37079=CARTESIAN_POINT('Ctrl Pts',(7.27603390512282,-115.079517970998,-4.20082013377274));
#37080=CARTESIAN_POINT('Ctrl Pts',(4.85068927007179,-114.904517970999,-8.40164026752833));
#37081=CARTESIAN_POINT('Ctrl Pts',(-1.4734904373448E-11,-114.729517970999,
-8.40164026751963));
#37082=CARTESIAN_POINT('Ctrl Pts',(-4.85068927010174,-114.554517970999,
-8.40164026751104));
#37083=CARTESIAN_POINT('Ctrl Pts',(-7.2760339051378,-114.379517970999,-4.2008201337468));
#37084=CARTESIAN_POINT('Ctrl Pts',(-9.70137854017372,-114.204517970999,
1.6962108644514E-11));
#37085=CARTESIAN_POINT('Ctrl Pts',(-7.27603390512287,-114.029517970999,
4.20082013377266));
#37086=CARTESIAN_POINT('Ctrl Pts',(-4.85068927007188,-113.854517970998,
8.40164026752828));
#37087=CARTESIAN_POINT('Ctrl Pts',(1.46443296023535E-11,-113.679517970999,
8.40164026751963));
#37088=CARTESIAN_POINT('Ctrl Pts',(4.85068927010165,-113.504517970999,8.40164026751109));
#37089=CARTESIAN_POINT('Ctrl Pts',(7.27603390513775,-113.329517970999,4.20082013374688));
#37090=CARTESIAN_POINT('Ctrl Pts',(9.70137854017372,-113.154517970999,-1.7408981431454E-11));
#37091=CARTESIAN_POINT('Ctrl Pts',(7.27603390512292,-112.979517970999,-4.20082013377258));
#37092=CARTESIAN_POINT('Ctrl Pts',(4.85068927007197,-112.804517970999,-8.40164026752823));
#37093=CARTESIAN_POINT('Ctrl Pts',(-1.50313327881035E-11,-112.629517970999,
-8.40164026751963));
#37094=CARTESIAN_POINT('Ctrl Pts',(-4.85068927010155,-112.454517970999,
-8.40164026751114));
#37095=CARTESIAN_POINT('Ctrl Pts',(-7.27603390513771,-112.279517970998,
-4.20082013374696));
#37096=CARTESIAN_POINT('Ctrl Pts',(-9.70137854017372,-112.104517970999,
1.73043946945076E-11));
#37097=CARTESIAN_POINT('Ctrl Pts',(-7.27603390512296,-111.929517970999,
4.2008201337725));
#37098=CARTESIAN_POINT('Ctrl Pts',(-4.85068927007206,-111.754517970999,
8.40164026752817));
#37099=CARTESIAN_POINT('Ctrl Pts',(1.49407580170091E-11,-111.579517970999,
8.40164026751963));
#37100=CARTESIAN_POINT('Ctrl Pts',(4.85068927010194,-111.404517970998,8.40164026751092));
#37101=CARTESIAN_POINT('Ctrl Pts',(7.27603390513766,-111.229517970999,4.20082013374704));
#37102=CARTESIAN_POINT('Ctrl Pts',(9.70137854017372,-111.054517970999,-1.71998079575613E-11));
#37103=CARTESIAN_POINT('Ctrl Pts',(7.27603390512277,-110.879517970999,-4.20082013377284));
#37104=CARTESIAN_POINT('Ctrl Pts',(4.85068927007215,-110.704517970999,-8.40164026752812));
#37105=CARTESIAN_POINT('Ctrl Pts',(-1.48501832459146E-11,-110.529517970999,
-8.40164026751963));
#37106=CARTESIAN_POINT('Ctrl Pts',(-4.85068927010185,-110.354517970999,
-8.40164026751097));
#37107=CARTESIAN_POINT('Ctrl Pts',(-7.27603390513762,-110.179517970999,
-4.20082013374712));
#37108=CARTESIAN_POINT('Ctrl Pts',(-9.70137854017372,-110.004517970999,
1.7095221220615E-11));
#37109=CARTESIAN_POINT('Ctrl Pts',(-7.27603390512281,-109.829517970999,
4.20082013377276));
#37110=CARTESIAN_POINT('Ctrl Pts',(-4.85068927007224,-109.654517970999,
8.40164026752807));
#37111=CARTESIAN_POINT('Ctrl Pts',(1.47596084748201E-11,-109.479517970999,
8.40164026751963));
#37112=CARTESIAN_POINT('Ctrl Pts',(4.85068927010176,-109.304517970999,8.40164026751102));
#37113=CARTESIAN_POINT('Ctrl Pts',(7.27603390513781,-109.129517970999,4.20082013374678));
#37114=CARTESIAN_POINT('Ctrl Pts',(9.70137854017372,-108.954517970999,-1.69906344836686E-11));
#37115=CARTESIAN_POINT('Ctrl Pts',(7.27603390512286,-108.779517970999,-4.20082013377268));
#37116=CARTESIAN_POINT('Ctrl Pts',(4.85068927007186,-108.604517970999,-8.40164026752829));
#37117=CARTESIAN_POINT('Ctrl Pts',(-1.46690337037257E-11,-108.429517970999,
-8.40164026751963));
#37118=CARTESIAN_POINT('Ctrl Pts',(-4.85068927010167,-108.254517970999,
-8.40164026751108));
#37119=CARTESIAN_POINT('Ctrl Pts',(-7.27603390513777,-108.079517970999,
-4.20082013374686));
#37120=CARTESIAN_POINT('Ctrl Pts',(-9.70137854017372,-107.904517970999,
1.68860477467223E-11));
#37121=CARTESIAN_POINT('Ctrl Pts',(-7.2760339051229,-107.729517970999,4.2008201337726));
#37122=CARTESIAN_POINT('Ctrl Pts',(-4.85068927007195,-107.554517970999,
8.40164026752824));
#37123=CARTESIAN_POINT('Ctrl Pts',(1.50560368894757E-11,-107.379517970999,
8.40164026751963));
#37124=CARTESIAN_POINT('Ctrl Pts',(4.85068927010158,-107.204517970999,8.40164026751113));
#37125=CARTESIAN_POINT('Ctrl Pts',(7.27603390513772,-107.029517970999,4.20082013374694));
#37126=CARTESIAN_POINT('Ctrl Pts',(9.70137854017372,-106.854517970999,-1.73329205336623E-11));
#37127=CARTESIAN_POINT('Ctrl Pts',(7.27603390512295,-106.679517970999,-4.20082013377253));
#37128=CARTESIAN_POINT('Ctrl Pts',(4.85068927007204,-106.504517970998,-8.40164026752819));
#37129=CARTESIAN_POINT('Ctrl Pts',(-1.49654621183812E-11,-106.329517970999,
-8.40164026751963));
#37130=CARTESIAN_POINT('Ctrl Pts',(-4.85068927010149,-106.154517970999,
-8.40164026751118));
#37131=CARTESIAN_POINT('Ctrl Pts',(-7.27603390513768,-105.979517970999,
-4.20082013374702));
#37132=CARTESIAN_POINT('Ctrl Pts',(-9.70137854017372,-105.804517970999,
1.72283337967159E-11));
#37133=CARTESIAN_POINT('Ctrl Pts',(-7.27603390512276,-105.629517970999,
4.20082013377286));
#37134=CARTESIAN_POINT('Ctrl Pts',(-4.85068927007213,-105.454517970999,
8.40164026752814));
#37135=CARTESIAN_POINT('Ctrl Pts',(1.48748873472868E-11,-105.279517970999,
8.40164026751963));
#37136=CARTESIAN_POINT('Ctrl Pts',(4.85068927010188,-105.104517970999,8.40164026751096));
#37137=CARTESIAN_POINT('Ctrl Pts',(7.27603390513763,-104.929517970999,4.2008201337471));
#37138=CARTESIAN_POINT('Ctrl Pts',(9.70137854017372,-104.754517970999,-1.71237470597696E-11));
#37139=CARTESIAN_POINT('Ctrl Pts',(7.2760339051228,-104.579517970999,-4.20082013377278));
#37140=CARTESIAN_POINT('Ctrl Pts',(4.85068927007222,-104.404517970999,-8.40164026752808));
#37141=CARTESIAN_POINT('Ctrl Pts',(-1.47843125761923E-11,-104.229517970999,
-8.40164026751963));
#37142=CARTESIAN_POINT('Ctrl Pts',(-4.85068927010179,-104.054517970999,
-8.40164026751101));
#37143=CARTESIAN_POINT('Ctrl Pts',(-7.27603390513758,-103.879517970999,
-4.20082013374717));
#37144=CARTESIAN_POINT('Ctrl Pts',(-9.70137854017372,-103.704517970999,
1.70191603228232E-11));
#37145=CARTESIAN_POINT('Ctrl Pts',(-7.27603390512285,-103.529517970999,
4.20082013377271));
#37146=CARTESIAN_POINT('Ctrl Pts',(-4.85068927007183,-103.354517970999,
8.40164026752831));
#37147=CARTESIAN_POINT('Ctrl Pts',(1.46937378050979E-11,-103.179517970999,
8.40164026751963));
#37148=CARTESIAN_POINT('Ctrl Pts',(4.85068927010169,-103.004517970999,8.40164026751106));
#37149=CARTESIAN_POINT('Ctrl Pts',(7.27603390513778,-102.829517970999,4.20082013374684));
#37150=CARTESIAN_POINT('Ctrl Pts',(9.70137854017372,-102.654517970999,-1.69145735858769E-11));
#37151=CARTESIAN_POINT('Ctrl Pts',(7.27603390512289,-102.479517970999,-4.20082013377263));
#37152=CARTESIAN_POINT('Ctrl Pts',(4.85068927007192,-102.304517970999,-8.40164026752825));
#37153=CARTESIAN_POINT('Ctrl Pts',(-1.46031630340034E-11,-102.129517970999,
-8.40164026751963));
#37154=CARTESIAN_POINT('Ctrl Pts',(-4.8506892701016,-101.954517970999,-8.40164026751111));
#37155=CARTESIAN_POINT('Ctrl Pts',(-7.27603390513773,-101.779517970999,
-4.20082013374692));
#37156=CARTESIAN_POINT('Ctrl Pts',(-9.70137854017372,-101.604517970999,
1.73614463728169E-11));
#37157=CARTESIAN_POINT('Ctrl Pts',(-7.27603390512294,-101.429517970999,
4.20082013377255));
#37158=CARTESIAN_POINT('Ctrl Pts',(-4.85068927007201,-101.254517970999,
8.4016402675282));
#37159=CARTESIAN_POINT('Ctrl Pts',(1.49901662197534E-11,-101.079517970999,
8.40164026751963));
#37160=CARTESIAN_POINT('Ctrl Pts',(4.85068927010151,-100.904517970999,8.40164026751117));
#37161=CARTESIAN_POINT('Ctrl Pts',(7.27603390513769,-100.729517970999,4.200820133747));
#37162=CARTESIAN_POINT('Ctrl Pts',(9.70137854017372,-100.554517970999,-1.72568596358705E-11));
#37163=CARTESIAN_POINT('Ctrl Pts',(7.27603390512298,-100.379517970999,-4.20082013377247));
#37164=CARTESIAN_POINT('Ctrl Pts',(4.8506892700721,-100.204517970999,-8.40164026752815));
#37165=CARTESIAN_POINT('Ctrl Pts',(-1.48995914486589E-11,-100.029517970999,
-8.40164026751963));
#37166=CARTESIAN_POINT('Ctrl Pts',(-4.8506892701019,-99.8545179709985,-8.40164026751094));
#37167=CARTESIAN_POINT('Ctrl Pts',(-7.27603390513764,-99.6795179709985,
-4.20082013374707));
#37168=CARTESIAN_POINT('Ctrl Pts',(-9.70137854017372,-99.5045179709985,
1.71522728989242E-11));
#37169=CARTESIAN_POINT('Ctrl Pts',(-7.27603390512279,-99.3295179709985,
4.2008201337728));
#37170=CARTESIAN_POINT('Ctrl Pts',(-4.85068927007219,-99.1545179709985,
8.4016402675281));
#37171=CARTESIAN_POINT('Ctrl Pts',(1.48090166775645E-11,-98.9795179709985,
8.40164026751963));
#37172=CARTESIAN_POINT('Ctrl Pts',(4.85068927010181,-98.8045179709985,8.401640267511));
#37173=CARTESIAN_POINT('Ctrl Pts',(7.2760339051376,-98.6295179709985,4.20082013374715));
#37174=CARTESIAN_POINT('Ctrl Pts',(9.70137854017372,-98.4545179709986,-1.70476861619779E-11));
#37175=CARTESIAN_POINT('Ctrl Pts',(7.27603390512283,-98.2795179709986,-4.20082013377273));
#37176=CARTESIAN_POINT('Ctrl Pts',(4.85068927007228,-98.1045179709985,-8.40164026752804));
#37177=CARTESIAN_POINT('Ctrl Pts',(-1.471844190647E-11,-97.9295179709985,
-8.40164026751963));
#37178=CARTESIAN_POINT('Ctrl Pts',(-4.85068927010172,-97.7545179709985,
-8.40164026751105));
#37179=CARTESIAN_POINT('Ctrl Pts',(-7.27603390513779,-97.5795179709986,
-4.20082013374682));
#37180=CARTESIAN_POINT('Ctrl Pts',(-9.70137854017372,-97.4045179709985,
1.69430994250315E-11));
#37181=CARTESIAN_POINT('Ctrl Pts',(-7.27603390512288,-97.2295179709985,
4.20082013377265));
#37182=CARTESIAN_POINT('Ctrl Pts',(-4.8506892700719,-97.0545179709985,8.40164026752827));
#37183=CARTESIAN_POINT('Ctrl Pts',(1.46278671353756E-11,-96.8795179709986,
8.40164026751963));
#37184=CARTESIAN_POINT('Ctrl Pts',(4.85068927010163,-96.7045179709986,8.4016402675111));
#37185=CARTESIAN_POINT('Ctrl Pts',(7.27603390513774,-96.5295179709985,4.2008201337469));
#37186=CARTESIAN_POINT('Ctrl Pts',(9.70137854017372,-96.3545179709985,-1.68385126880852E-11));
#37187=CARTESIAN_POINT('Ctrl Pts',(7.27603390512292,-96.1795179709985,-4.20082013377257));
#37188=CARTESIAN_POINT('Ctrl Pts',(4.85068927007199,-96.0045179709986,-8.40164026752822));
#37189=CARTESIAN_POINT('Ctrl Pts',(-1.50148703211256E-11,-95.8295179709985,
-8.40164026751963));
#37190=CARTESIAN_POINT('Ctrl Pts',(-4.85068927010154,-95.6545179709985,
-8.40164026751115));
#37191=CARTESIAN_POINT('Ctrl Pts',(-7.2760339051377,-95.4795179709985,-4.20082013374698));
#37192=CARTESIAN_POINT('Ctrl Pts',(-9.70137854017372,-95.3045179709985,
1.72853854750252E-11));
#37193=CARTESIAN_POINT('Ctrl Pts',(-7.27603390512297,-95.1295179709986,
4.20082013377249));
#37194=CARTESIAN_POINT('Ctrl Pts',(-4.85068927007208,-94.9545179709986,
8.40164026752816));
#37195=CARTESIAN_POINT('Ctrl Pts',(1.49242955500311E-11,-94.7795179709985,
8.40164026751963));
#37196=CARTESIAN_POINT('Ctrl Pts',(4.85068927010145,-94.6045179709986,8.40164026751121));
#37197=CARTESIAN_POINT('Ctrl Pts',(7.27603390513766,-94.4295179709985,4.20082013374705));
#37198=CARTESIAN_POINT('Ctrl Pts',(9.70137854017372,-94.2545179709985,-1.71807987380788E-11));
#37199=CARTESIAN_POINT('Ctrl Pts',(7.27603390512277,-94.0795179709986,-4.20082013377283));
#37200=CARTESIAN_POINT('Ctrl Pts',(4.85068927007217,-93.9045179709986,-8.40164026752811));
#37201=CARTESIAN_POINT('Ctrl Pts',(-1.48337207789367E-11,-93.7295179709986,
-8.40164026751963));
#37202=CARTESIAN_POINT('Ctrl Pts',(-4.85068927010184,-93.5545179709985,
-8.40164026751098));
#37203=CARTESIAN_POINT('Ctrl Pts',(-7.27603390513761,-93.3795179709985,
-4.20082013374713));
#37204=CARTESIAN_POINT('Ctrl Pts',(-9.70137854017372,-93.2045179709986,
1.70762120011325E-11));
#37205=CARTESIAN_POINT('Ctrl Pts',(-7.27603390512282,-93.0295179709986,
4.20082013377275));
#37206=CARTESIAN_POINT('Ctrl Pts',(-4.85068927007226,-92.8545179709985,
8.40164026752806));
#37207=CARTESIAN_POINT('Ctrl Pts',(1.47431460078422E-11,-92.6795179709985,
8.40164026751963));
#37208=CARTESIAN_POINT('Ctrl Pts',(4.85068927010175,-92.5045179709985,8.40164026751103));
#37209=CARTESIAN_POINT('Ctrl Pts',(7.2760339051378,-92.3295179709986,4.2008201337468));
#37210=CARTESIAN_POINT('Ctrl Pts',(9.70137854017372,-92.1545179709986,-1.69716252641861E-11));
#37211=CARTESIAN_POINT('Ctrl Pts',(7.27603390512287,-91.9795179709986,-4.20082013377267));
#37212=CARTESIAN_POINT('Ctrl Pts',(4.85068927007187,-91.8045179709985,-8.40164026752828));
#37213=CARTESIAN_POINT('Ctrl Pts',(-1.46525712367478E-11,-91.6295179709986,
-8.40164026751963));
#37214=CARTESIAN_POINT('Ctrl Pts',(-4.85068927010165,-91.4545179709986,
-8.40164026751109));
#37215=CARTESIAN_POINT('Ctrl Pts',(-7.27603390513776,-91.2795179709986,
-4.20082013374688));
#37216=CARTESIAN_POINT('Ctrl Pts',(-9.70137854017372,-91.1045179709986,
1.68670385272398E-11));
#37217=CARTESIAN_POINT('Ctrl Pts',(-7.27603390512291,-90.9295179709986,
4.20082013377259));
#37218=CARTESIAN_POINT('Ctrl Pts',(-4.85068927007196,-90.7545179709986,
8.40164026752823));
#37219=CARTESIAN_POINT('Ctrl Pts',(1.45619964656533E-11,-90.5795179709986,
8.40164026751963));
#37220=CARTESIAN_POINT('Ctrl Pts',(4.85068927010157,-90.4045179709985,8.40164026751114));
#37221=CARTESIAN_POINT('Ctrl Pts',(7.27603390513771,-90.2295179709986,4.20082013374695));
#37222=CARTESIAN_POINT('Ctrl Pts',(9.70137854017372,-90.0545179709986,-1.73139113141798E-11));
#37223=CARTESIAN_POINT('Ctrl Pts',(7.27603390512296,-89.8795179709985,-4.20082013377251));
#37224=CARTESIAN_POINT('Ctrl Pts',(4.85068927007205,-89.7045179709986,-8.40164026752818));
#37225=CARTESIAN_POINT('Ctrl Pts',(-1.49489996514033E-11,-89.5295179709986,
-8.40164026751963));
#37226=CARTESIAN_POINT('Ctrl Pts',(-4.85068927010147,-89.3545179709986,
-8.40164026751119));
#37227=CARTESIAN_POINT('Ctrl Pts',(-7.27603390513767,-89.1795179709986,
-4.20082013374703));
#37228=CARTESIAN_POINT('Ctrl Pts',(-9.70137854017372,-89.0045179709985,
1.72093245772335E-11));
#37229=CARTESIAN_POINT('Ctrl Pts',(-7.276033905123,-88.8295179709986,4.20082013377243));
#37230=CARTESIAN_POINT('Ctrl Pts',(-4.85068927007214,-88.6545179709986,
8.40164026752813));
#37231=CARTESIAN_POINT('Ctrl Pts',(1.48584248803088E-11,-88.4795179709986,
8.40164026751963));
#37232=CARTESIAN_POINT('Ctrl Pts',(4.85068927010186,-88.3045179709985,8.40164026751097));
#37233=CARTESIAN_POINT('Ctrl Pts',(7.27603390513762,-88.1295179709985,4.20082013374711));
#37234=CARTESIAN_POINT('Ctrl Pts',(9.70137854017372,-87.9545179709986,-1.71047378402871E-11));
#37235=CARTESIAN_POINT('Ctrl Pts',(7.27603390512281,-87.7795179709986,-4.20082013377277));
#37236=CARTESIAN_POINT('Ctrl Pts',(4.85068927007223,-87.6045179709986,-8.40164026752807));
#37237=CARTESIAN_POINT('Ctrl Pts',(-1.47678501092144E-11,-87.4295179709986,
-8.40164026751963));
#37238=CARTESIAN_POINT('Ctrl Pts',(-4.85068927010177,-87.2545179709985,
-8.40164026751102));
#37239=CARTESIAN_POINT('Ctrl Pts',(-7.27603390513758,-87.0795179709986,
-4.20082013374719));
#37240=CARTESIAN_POINT('Ctrl Pts',(-9.70137854017372,-86.9045179709986,
1.70001511033408E-11));
#37241=CARTESIAN_POINT('Ctrl Pts',(-7.27603390512285,-86.7295179709986,
4.20082013377269));
#37242=CARTESIAN_POINT('Ctrl Pts',(-4.85068927007185,-86.5545179709986,
8.4016402675283));
#37243=CARTESIAN_POINT('Ctrl Pts',(1.46772753381199E-11,-86.3795179709986,
8.40164026751963));
#37244=CARTESIAN_POINT('Ctrl Pts',(4.85068927010168,-86.2045179709986,8.40164026751107));
#37245=CARTESIAN_POINT('Ctrl Pts',(7.27603390513777,-86.0295179709986,4.20082013374685));
#37246=CARTESIAN_POINT('Ctrl Pts',(9.70137854017372,-85.8545179709986,-1.68955643663944E-11));
#37247=CARTESIAN_POINT('Ctrl Pts',(7.2760339051229,-85.6795179709986,-4.20082013377261));
#37248=CARTESIAN_POINT('Ctrl Pts',(4.85068927007194,-85.5045179709986,-8.40164026752825));
#37249=CARTESIAN_POINT('Ctrl Pts',(-1.45867005670255E-11,-85.3295179709986,
-8.40164026751963));
#37250=CARTESIAN_POINT('Ctrl Pts',(-4.85068927010159,-85.1545179709986,
-8.40164026751112));
#37251=CARTESIAN_POINT('Ctrl Pts',(-7.27603390513773,-84.9795179709986,
-4.20082013374693));
#37252=CARTESIAN_POINT('Ctrl Pts',(-9.70137854017372,-84.8045179709986,
1.67909776294481E-11));
#37253=CARTESIAN_POINT('Ctrl Pts',(-7.27603390512294,-84.6295179709986,
4.20082013377253));
#37254=CARTESIAN_POINT('Ctrl Pts',(-4.85068927007203,-84.4545179709986,
8.40164026752819));
#37255=CARTESIAN_POINT('Ctrl Pts',(1.49737037527755E-11,-84.2795179709986,
8.40164026751963));
#37256=CARTESIAN_POINT('Ctrl Pts',(4.8506892701015,-84.1045179709986,8.40164026751117));
#37257=CARTESIAN_POINT('Ctrl Pts',(7.27603390513768,-83.9295179709986,4.20082013374701));
#37258=CARTESIAN_POINT('Ctrl Pts',(9.70137854017372,-83.7545179709986,-1.72378504163881E-11));
#37259=CARTESIAN_POINT('Ctrl Pts',(7.27603390512299,-83.5795179709986,-4.20082013377245));
#37260=CARTESIAN_POINT('Ctrl Pts',(4.85068927007212,-83.4045179709986,-8.40164026752814));
#37261=CARTESIAN_POINT('Ctrl Pts',(-1.4883128981681E-11,-83.2295179709986,
-8.40164026751963));
#37262=CARTESIAN_POINT('Ctrl Pts',(-4.85068927010141,-83.0545179709986,
-8.40164026751123));
#37263=CARTESIAN_POINT('Ctrl Pts',(-7.27603390513763,-82.8795179709986,
-4.20082013374709));
#37264=CARTESIAN_POINT('Ctrl Pts',(-9.70137854017372,-82.7045179709986,
1.71332636794417E-11));
#37265=CARTESIAN_POINT('Ctrl Pts',(-7.2760339051228,-82.5295179709986,4.20082013377279));
#37266=CARTESIAN_POINT('Ctrl Pts',(-4.85068927007221,-82.3545179709986,
8.40164026752809));
#37267=CARTESIAN_POINT('Ctrl Pts',(1.47925542105866E-11,-82.1795179709986,
8.40164026751963));
#37268=CARTESIAN_POINT('Ctrl Pts',(4.85068927010179,-82.0045179709986,8.401640267511));
#37269=CARTESIAN_POINT('Ctrl Pts',(7.27603390513759,-81.8295179709986,4.20082013374717));
#37270=CARTESIAN_POINT('Ctrl Pts',(9.70137854017372,-81.6545179709986,-1.70286769424954E-11));
#37271=CARTESIAN_POINT('Ctrl Pts',(7.27603390512284,-81.4795179709986,-4.20082013377271));
#37272=CARTESIAN_POINT('Ctrl Pts',(4.8506892700723,-81.3045179709986,-8.40164026752804));
#37273=CARTESIAN_POINT('Ctrl Pts',(-1.47019794394921E-11,-81.1295179709986,
-8.40164026751963));
#37274=CARTESIAN_POINT('Ctrl Pts',(-4.8506892701017,-80.9545179709986,-8.40164026751106));
#37275=CARTESIAN_POINT('Ctrl Pts',(-7.27603390513778,-80.7795179709986,
-4.20082013374683));
#37276=CARTESIAN_POINT('Ctrl Pts',(-9.70137854017372,-80.6045179709986,
1.69240902055491E-11));
#37277=CARTESIAN_POINT('Ctrl Pts',(-7.27603390512289,-80.4295179709986,
4.20082013377263));
#37278=CARTESIAN_POINT('Ctrl Pts',(-4.85068927007191,-80.2545179709986,
8.40164026752826));
#37279=CARTESIAN_POINT('Ctrl Pts',(1.46114046683977E-11,-80.0795179709986,
8.40164026751963));
#37280=CARTESIAN_POINT('Ctrl Pts',(4.85068927010161,-79.9045179709986,8.40164026751111));
#37281=CARTESIAN_POINT('Ctrl Pts',(7.27603390513774,-79.7295179709986,4.20082013374691));
#37282=CARTESIAN_POINT('Ctrl Pts',(9.70137854017372,-79.5545179709986,-1.68195034686027E-11));
#37283=CARTESIAN_POINT('Ctrl Pts',(7.27603390512293,-79.3795179709986,-4.20082013377256));
#37284=CARTESIAN_POINT('Ctrl Pts',(4.850689270072,-79.2045179709986,-8.40164026752821));
#37285=CARTESIAN_POINT('Ctrl Pts',(-1.49984078541476E-11,-79.0295179709986,
-8.40164026751963));
#37286=CARTESIAN_POINT('Ctrl Pts',(-4.85068927010152,-78.8545179709986,
-8.40164026751116));
#37287=CARTESIAN_POINT('Ctrl Pts',(-7.27603390513769,-78.6795179709986,
-4.20082013374699));
#37288=CARTESIAN_POINT('Ctrl Pts',(-9.70137854017372,-78.5045179709986,
1.72663762555427E-11));
#37289=CARTESIAN_POINT('Ctrl Pts',(-7.27603390512298,-78.3295179709986,
4.20082013377248));
#37290=CARTESIAN_POINT('Ctrl Pts',(-4.85068927007209,-78.1545179709986,
8.40164026752815));
#37291=CARTESIAN_POINT('Ctrl Pts',(1.49078330830532E-11,-77.9795179709986,
8.40164026751963));
#37292=CARTESIAN_POINT('Ctrl Pts',(4.85068927010143,-77.8045179709986,8.40164026751122));
#37293=CARTESIAN_POINT('Ctrl Pts',(7.27603390513765,-77.6295179709986,4.20082013374707));
#37294=CARTESIAN_POINT('Ctrl Pts',(9.70137854017372,-77.4545179709986,-1.71617895185964E-11));
#37295=CARTESIAN_POINT('Ctrl Pts',(7.27603390512302,-77.2795179709986,-4.2008201337724));
#37296=CARTESIAN_POINT('Ctrl Pts',(4.85068927007219,-77.1045179709986,-8.4016402675281));
#37297=CARTESIAN_POINT('Ctrl Pts',(-1.48172583119587E-11,-76.9295179709986,
-8.40164026751963));
#37298=CARTESIAN_POINT('Ctrl Pts',(-4.85068927010182,-76.7545179709986,
-8.40164026751099));
#37299=CARTESIAN_POINT('Ctrl Pts',(-7.2760339051376,-76.5795179709986,-4.20082013374715));
#37300=CARTESIAN_POINT('Ctrl Pts',(-9.70137854017372,-76.4045179709986,
1.705720278165E-11));
#37301=CARTESIAN_POINT('Ctrl Pts',(-7.27603390512283,-76.2295179709986,
4.20082013377273));
#37302=CARTESIAN_POINT('Ctrl Pts',(-4.85068927007227,-76.0545179709986,
8.40164026752805));
#37303=CARTESIAN_POINT('Ctrl Pts',(1.47266835408643E-11,-75.8795179709986,
8.40164026751963));
#37304=CARTESIAN_POINT('Ctrl Pts',(4.85068927010173,-75.7045179709986,8.40164026751104));
#37305=CARTESIAN_POINT('Ctrl Pts',(7.27603390513756,-75.5295179709986,4.20082013374722));
#37306=CARTESIAN_POINT('Ctrl Pts',(9.70137854017372,-75.3545179709986,-1.69526160447037E-11));
#37307=CARTESIAN_POINT('Ctrl Pts',(7.27603390512287,-75.1795179709986,-4.20082013377265));
#37308=CARTESIAN_POINT('Ctrl Pts',(4.85068927007189,-75.0045179709986,-8.40164026752827));
#37309=CARTESIAN_POINT('Ctrl Pts',(-1.46361087697698E-11,-74.8295179709986,
-8.40164026751963));
#37310=CARTESIAN_POINT('Ctrl Pts',(-4.85068927010164,-74.6545179709986,
-8.40164026751109));
#37311=CARTESIAN_POINT('Ctrl Pts',(-7.27603390513775,-74.4795179709986,
-4.20082013374689));
#37312=CARTESIAN_POINT('Ctrl Pts',(-9.70137854017372,-74.3045179709986,
1.68480293077573E-11));
#37313=CARTESIAN_POINT('Ctrl Pts',(-7.27603390512292,-74.1295179709986,
4.20082013377258));
#37314=CARTESIAN_POINT('Ctrl Pts',(-4.85068927007198,-73.9545179709986,
8.40164026752822));
#37315=CARTESIAN_POINT('Ctrl Pts',(1.45455339986754E-11,-73.7795179709986,
8.40164026751963));
#37316=CARTESIAN_POINT('Ctrl Pts',(4.85068927010155,-73.6045179709986,8.40164026751115));
#37317=CARTESIAN_POINT('Ctrl Pts',(7.2760339051377,-73.4295179709986,4.20082013374697));
#37318=CARTESIAN_POINT('Ctrl Pts',(9.70137854017372,-73.2545179709986,-1.72949020946973E-11));
#37319=CARTESIAN_POINT('Ctrl Pts',(7.27603390512296,-73.0795179709986,-4.2008201337725));
#37320=CARTESIAN_POINT('Ctrl Pts',(4.85068927007207,-72.9045179709986,-8.40164026752817));
#37321=CARTESIAN_POINT('Ctrl Pts',(-1.49325371844254E-11,-72.7295179709986,
-8.40164026751963));
#37322=CARTESIAN_POINT('Ctrl Pts',(-4.85068927010146,-72.5545179709986,
-8.4016402675112));
#37323=CARTESIAN_POINT('Ctrl Pts',(-7.27603390513766,-72.3795179709986,
-4.20082013374705));
#37324=CARTESIAN_POINT('Ctrl Pts',(-9.70137854017372,-72.2045179709986,
1.7190315357751E-11));
#37325=CARTESIAN_POINT('Ctrl Pts',(-7.27603390512301,-72.0295179709986,
4.20082013377242));
#37326=CARTESIAN_POINT('Ctrl Pts',(-4.85068927007216,-71.8545179709986,
8.40164026752812));
#37327=CARTESIAN_POINT('Ctrl Pts',(1.48419624133309E-11,-71.6795179709986,
8.40164026751963));
#37328=CARTESIAN_POINT('Ctrl Pts',(4.85068927010137,-71.5045179709986,8.40164026751125));
#37329=CARTESIAN_POINT('Ctrl Pts',(7.27603390513761,-71.3295179709986,4.20082013374713));
#37330=CARTESIAN_POINT('Ctrl Pts',(9.70137854017372,-71.1545179709986,-1.70857286208046E-11));
#37331=CARTESIAN_POINT('Ctrl Pts',(7.27603390512282,-70.9795179709986,-4.20082013377275));
#37332=CARTESIAN_POINT('Ctrl Pts',(4.85068927007225,-70.8045179709986,-8.40164026752806));
#37333=CARTESIAN_POINT('Ctrl Pts',(-1.47513876422365E-11,-70.6295179709986,
-8.40164026751963));
#37334=CARTESIAN_POINT('Ctrl Pts',(-4.85068927010175,-70.4545179709986,
-8.40164026751103));
#37335=CARTESIAN_POINT('Ctrl Pts',(-7.27603390513757,-70.2795179709986,
-4.2008201337472));
#37336=CARTESIAN_POINT('Ctrl Pts',(-9.70137854017372,-70.1045179709986,
1.69811418838583E-11));
#37337=CARTESIAN_POINT('Ctrl Pts',(-7.27603390512286,-69.9295179709986,
4.20082013377267));
#37338=CARTESIAN_POINT('Ctrl Pts',(-4.85068927007234,-69.7545179709986,
8.40164026752801));
#37339=CARTESIAN_POINT('Ctrl Pts',(1.4660812871142E-11,-69.5795179709986,
8.40164026751963));
#37340=CARTESIAN_POINT('Ctrl Pts',(4.85068927010166,-69.4045179709986,8.40164026751108));
#37341=CARTESIAN_POINT('Ctrl Pts',(7.27603390513776,-69.2295179709986,4.20082013374687));
#37342=CARTESIAN_POINT('Ctrl Pts',(9.70137854017372,-69.0545179709986,-1.6876555146912E-11));
#37343=CARTESIAN_POINT('Ctrl Pts',(7.27603390512291,-68.8795179709986,-4.2008201337726));
#37344=CARTESIAN_POINT('Ctrl Pts',(4.85068927007195,-68.7045179709986,-8.40164026752823));
#37345=CARTESIAN_POINT('Ctrl Pts',(-1.45702381000475E-11,-68.5295179709986,
-8.40164026751963));
#37346=CARTESIAN_POINT('Ctrl Pts',(-4.85068927010157,-68.3545179709986,
-8.40164026751113));
#37347=CARTESIAN_POINT('Ctrl Pts',(-7.27603390513772,-68.1795179709986,
-4.20082013374695));
#37348=CARTESIAN_POINT('Ctrl Pts',(-9.70137854017372,-68.0045179709986,
1.67719684099656E-11));
#37349=CARTESIAN_POINT('Ctrl Pts',(-7.27603390512295,-67.8295179709986,
4.20082013377252));
#37350=CARTESIAN_POINT('Ctrl Pts',(-4.85068927007204,-67.6545179709986,
8.40164026752818));
#37351=CARTESIAN_POINT('Ctrl Pts',(1.49572412857975E-11,-67.4795179709986,
8.40164026751963));
#37352=CARTESIAN_POINT('Ctrl Pts',(4.85068927010148,-67.3045179709986,8.40164026751119));
#37353=CARTESIAN_POINT('Ctrl Pts',(7.27603390513767,-67.1295179709986,4.20082013374703));
#37354=CARTESIAN_POINT('Ctrl Pts',(9.70137854017372,-66.9545179709986,-1.72188411969056E-11));
#37355=CARTESIAN_POINT('Ctrl Pts',(7.276033905123,-66.7795179709986,-4.20082013377244));
#37356=CARTESIAN_POINT('Ctrl Pts',(4.85068927007213,-66.6045179709986,-8.40164026752813));
#37357=CARTESIAN_POINT('Ctrl Pts',(-1.48666665147031E-11,-66.4295179709986,
-8.40164026751963));
#37358=CARTESIAN_POINT('Ctrl Pts',(-4.85068927010139,-66.2545179709986,
-8.40164026751124));
#37359=CARTESIAN_POINT('Ctrl Pts',(-7.27603390513763,-66.0795179709986,
-4.2008201337471));
#37360=CARTESIAN_POINT('Ctrl Pts',(-9.70137854017372,-65.9045179709986,
1.71142544599593E-11));
#37361=CARTESIAN_POINT('Ctrl Pts',(-7.27603390512304,-65.7295179709986,
4.20082013377236));
#37362=CARTESIAN_POINT('Ctrl Pts',(-4.85068927007222,-65.5545179709986,
8.40164026752808));
#37363=CARTESIAN_POINT('Ctrl Pts',(1.47760917436086E-11,-65.3795179709986,
8.40164026751963));
#37364=CARTESIAN_POINT('Ctrl Pts',(4.85068927010178,-65.2045179709986,8.40164026751101));
#37365=CARTESIAN_POINT('Ctrl Pts',(7.27603390513758,-65.0295179709986,4.20082013374718));
#37366=CARTESIAN_POINT('Ctrl Pts',(9.70137854017372,-64.8545179709986,-1.70096677230129E-11));
#37367=CARTESIAN_POINT('Ctrl Pts',(7.27603390512285,-64.6795179709986,-4.2008201337727));
#37368=CARTESIAN_POINT('Ctrl Pts',(4.85068927007232,-64.5045179709986,-8.40164026752803));
#37369=CARTESIAN_POINT('Ctrl Pts',(-1.46855169725142E-11,-64.3295179709986,
-8.40164026751963));
#37370=CARTESIAN_POINT('Ctrl Pts',(-4.85068927010169,-64.1545179709986,
-8.40164026751107));
#37371=CARTESIAN_POINT('Ctrl Pts',(-7.27603390513754,-63.9795179709986,
-4.20082013374726));
#37372=CARTESIAN_POINT('Ctrl Pts',(-9.70137854017372,-63.8045179709986,
1.69050809860666E-11));
#37373=CARTESIAN_POINT('Ctrl Pts',(-7.27603390512289,-63.6295179709986,
4.20082013377262));
#37374=CARTESIAN_POINT('Ctrl Pts',(-4.85068927007193,-63.4545179709986,
8.40164026752825));
#37375=CARTESIAN_POINT('Ctrl Pts',(1.45949422014197E-11,-63.2795179709986,
8.40164026751963));
#37376=CARTESIAN_POINT('Ctrl Pts',(4.8506892701016,-63.1045179709986,8.40164026751112));
#37377=CARTESIAN_POINT('Ctrl Pts',(7.27603390513773,-62.9295179709986,4.20082013374692));
#37378=CARTESIAN_POINT('Ctrl Pts',(9.70137854017372,-62.7545179709986,-1.68004942491202E-11));
#37379=CARTESIAN_POINT('Ctrl Pts',(7.27603390512294,-62.5795179709986,-4.20082013377254));
#37380=CARTESIAN_POINT('Ctrl Pts',(4.85068927007202,-62.4045179709986,-8.4016402675282));
#37381=CARTESIAN_POINT('Ctrl Pts',(-1.45043674303253E-11,-62.2295179709986,
-8.40164026751963));
#37382=CARTESIAN_POINT('Ctrl Pts',(-4.85068927010151,-62.0545179709986,
-8.40164026751117));
#37383=CARTESIAN_POINT('Ctrl Pts',(-7.27603390513768,-61.8795179709986,
-4.200820133747));
#37384=CARTESIAN_POINT('Ctrl Pts',(-9.70137854017372,-61.7045179709986,
1.72473670360602E-11));
#37385=CARTESIAN_POINT('Ctrl Pts',(-7.27603390512298,-61.5295179709986,
4.20082013377246));
#37386=CARTESIAN_POINT('Ctrl Pts',(-4.85068927007211,-61.3545179709986,
8.40164026752814));
#37387=CARTESIAN_POINT('Ctrl Pts',(1.48913706160753E-11,-61.1795179709986,
8.40164026751963));
#37388=CARTESIAN_POINT('Ctrl Pts',(4.85068927010141,-61.0045179709986,8.40164026751122));
#37389=CARTESIAN_POINT('Ctrl Pts',(7.27603390513764,-60.8295179709986,4.20082013374708));
#37390=CARTESIAN_POINT('Ctrl Pts',(9.70137854017372,-60.6545179709986,-1.71427802991139E-11));
#37391=CARTESIAN_POINT('Ctrl Pts',(7.27603390512303,-60.4795179709986,-4.20082013377238));
#37392=CARTESIAN_POINT('Ctrl Pts',(4.8506892700722,-60.3045179709986,-8.40164026752809));
#37393=CARTESIAN_POINT('Ctrl Pts',(-1.48007958449808E-11,-60.1295179709986,
-8.40164026751963));
#37394=CARTESIAN_POINT('Ctrl Pts',(-4.8506892701018,-59.9545179709986,-8.401640267511));
#37395=CARTESIAN_POINT('Ctrl Pts',(-7.27603390513759,-59.7795179709986,
-4.20082013374716));
#37396=CARTESIAN_POINT('Ctrl Pts',(-9.70137854017372,-59.6045179709986,
1.70381935621676E-11));
#37397=CARTESIAN_POINT('Ctrl Pts',(-7.27603390512284,-59.4295179709986,
4.20082013377272));
#37398=CARTESIAN_POINT('Ctrl Pts',(-4.85068927007229,-59.2545179709986,
8.40164026752804));
#37399=CARTESIAN_POINT('Ctrl Pts',(1.47102210738864E-11,-59.0795179709986,
8.40164026751963));
#37400=CARTESIAN_POINT('Ctrl Pts',(4.85068927010171,-58.9045179709986,8.40164026751105));
#37401=CARTESIAN_POINT('Ctrl Pts',(7.27603390513755,-58.7295179709986,4.20082013374724));
#37402=CARTESIAN_POINT('Ctrl Pts',(9.70137854017372,-58.5545179709986,-1.69336068252212E-11));
#37403=CARTESIAN_POINT('Ctrl Pts',(7.27603390512288,-58.3795179709986,-4.20082013377264));
#37404=CARTESIAN_POINT('Ctrl Pts',(4.85068927007238,-58.2045179709986,-8.40164026752799));
#37405=CARTESIAN_POINT('Ctrl Pts',(-1.46196463027919E-11,-58.0295179709986,
-8.40164026751963));
#37406=CARTESIAN_POINT('Ctrl Pts',(-4.85068927010162,-57.8545179709986,
-8.40164026751111));
#37407=CARTESIAN_POINT('Ctrl Pts',(-7.27603390513774,-57.6795179709986,
-4.2008201337469));
#37408=CARTESIAN_POINT('Ctrl Pts',(-9.70137854017372,-57.5045179709986,
1.68290200882749E-11));
#37409=CARTESIAN_POINT('Ctrl Pts',(-7.27603390512293,-57.3295179709986,
4.20082013377256));
#37410=CARTESIAN_POINT('Ctrl Pts',(-4.85068927007199,-57.1545179709986,
8.40164026752821));
#37411=CARTESIAN_POINT('Ctrl Pts',(1.45290715316974E-11,-56.9795179709986,
8.40164026751963));
#37412=CARTESIAN_POINT('Ctrl Pts',(4.85068927010153,-56.8045179709986,8.40164026751116));
#37413=CARTESIAN_POINT('Ctrl Pts',(7.2760339051377,-56.6295179709986,4.20082013374698));
#37414=CARTESIAN_POINT('Ctrl Pts',(9.70137854017372,-56.4545179709986,-1.67244333513285E-11));
#37415=CARTESIAN_POINT('Ctrl Pts',(7.27603390512297,-56.2795179709986,-4.20082013377248));
#37416=CARTESIAN_POINT('Ctrl Pts',(4.85068927007208,-56.1045179709986,-8.40164026752816));
#37417=CARTESIAN_POINT('Ctrl Pts',(-1.49160747174474E-11,-55.9295179709986,
-8.40164026751963));
#37418=CARTESIAN_POINT('Ctrl Pts',(-4.85068927010144,-55.7545179709987,
-8.40164026751121));
#37419=CARTESIAN_POINT('Ctrl Pts',(-7.27603390513765,-55.5795179709986,
-4.20082013374706));
#37420=CARTESIAN_POINT('Ctrl Pts',(-9.70137854017372,-55.4045179709986,
1.71713061382685E-11));
#37421=CARTESIAN_POINT('Ctrl Pts',(-7.27603390512302,-55.2295179709986,
4.2008201337724));
#37422=CARTESIAN_POINT('Ctrl Pts',(-4.85068927007218,-55.0545179709986,
8.40164026752811));
#37423=CARTESIAN_POINT('Ctrl Pts',(1.4825499946353E-11,-54.8795179709986,
8.40164026751963));
#37424=CARTESIAN_POINT('Ctrl Pts',(4.85068927010135,-54.7045179709987,8.40164026751126));
#37425=CARTESIAN_POINT('Ctrl Pts',(7.27603390513761,-54.5295179709986,4.20082013374714));
#37426=CARTESIAN_POINT('Ctrl Pts',(9.70137854017372,-54.3545179709986,-1.70667194013222E-11));
#37427=CARTESIAN_POINT('Ctrl Pts',(7.27603390512282,-54.1795179709986,-4.20082013377274));
#37428=CARTESIAN_POINT('Ctrl Pts',(4.85068927007227,-54.0045179709986,-8.40164026752806));
#37429=CARTESIAN_POINT('Ctrl Pts',(-1.47349251752585E-11,-53.8295179709986,
-8.40164026751963));
#37430=CARTESIAN_POINT('Ctrl Pts',(-4.85068927010174,-53.6545179709986,
-8.40164026751104));
#37431=CARTESIAN_POINT('Ctrl Pts',(-7.27603390513756,-53.4795179709987,
-4.20082013374722));
#37432=CARTESIAN_POINT('Ctrl Pts',(-9.70137854017372,-53.3045179709987,
1.69621326643758E-11));
#37433=CARTESIAN_POINT('Ctrl Pts',(-7.27603390512287,-53.1295179709986,
4.20082013377266));
#37434=CARTESIAN_POINT('Ctrl Pts',(-4.85068927007236,-52.9545179709987,
8.401640267528));
#37435=CARTESIAN_POINT('Ctrl Pts',(1.46443504041641E-11,-52.7795179709986,
8.40164026751963));
#37436=CARTESIAN_POINT('Ctrl Pts',(4.85068927010165,-52.6045179709986,8.40164026751109));
#37437=CARTESIAN_POINT('Ctrl Pts',(7.27603390513752,-52.4295179709987,4.2008201337473));
#37438=CARTESIAN_POINT('Ctrl Pts',(9.70137854017372,-52.2545179709986,-1.68575459274295E-11));
#37439=CARTESIAN_POINT('Ctrl Pts',(7.27603390512292,-52.0795179709986,-4.20082013377258));
#37440=CARTESIAN_POINT('Ctrl Pts',(4.85068927007197,-51.9045179709987,-8.40164026752823));
#37441=CARTESIAN_POINT('Ctrl Pts',(-1.45537756330696E-11,-51.7295179709986,
-8.40164026751963));
#37442=CARTESIAN_POINT('Ctrl Pts',(-4.85068927010155,-51.5545179709986,
-8.40164026751114));
#37443=CARTESIAN_POINT('Ctrl Pts',(-7.27603390513771,-51.3795179709987,
-4.20082013374696));
#37444=CARTESIAN_POINT('Ctrl Pts',(-9.70137854017372,-51.2045179709986,
1.67529591904832E-11));
#37445=CARTESIAN_POINT('Ctrl Pts',(-7.27603390512296,-51.0295179709986,
4.2008201337725));
#37446=CARTESIAN_POINT('Ctrl Pts',(-4.85068927007206,-50.8545179709987,
8.40164026752817));
#37447=CARTESIAN_POINT('Ctrl Pts',(1.44632008619752E-11,-50.6795179709987,
8.40164026751963));
#37448=CARTESIAN_POINT('Ctrl Pts',(4.85068927010146,-50.5045179709986,8.4016402675112));
#37449=CARTESIAN_POINT('Ctrl Pts',(7.27603390513766,-50.3295179709987,4.20082013374704));
#37450=CARTESIAN_POINT('Ctrl Pts',(9.70137854017372,-50.1545179709987,-1.71998319774232E-11));
#37451=CARTESIAN_POINT('Ctrl Pts',(7.27603390512301,-49.9795179709986,-4.20082013377243));
#37452=CARTESIAN_POINT('Ctrl Pts',(4.85068927007215,-49.8045179709986,-8.40164026752812));
#37453=CARTESIAN_POINT('Ctrl Pts',(-1.48502040477252E-11,-49.6295179709987,
-8.40164026751963));
#37454=CARTESIAN_POINT('Ctrl Pts',(-4.85068927010137,-49.4545179709986,
-8.40164026751125));
#37455=CARTESIAN_POINT('Ctrl Pts',(-7.27603390513762,-49.2795179709986,
-4.20082013374712));
#37456=CARTESIAN_POINT('Ctrl Pts',(-9.70137854017372,-49.1045179709987,
1.70952452404768E-11));
#37457=CARTESIAN_POINT('Ctrl Pts',(-7.27603390512305,-48.9295179709987,
4.20082013377235));
#37458=CARTESIAN_POINT('Ctrl Pts',(-4.85068927007224,-48.7545179709986,
8.40164026752807));
#37459=CARTESIAN_POINT('Ctrl Pts',(1.47596292766307E-11,-48.5795179709987,
8.40164026751963));
#37460=CARTESIAN_POINT('Ctrl Pts',(4.85068927010176,-48.4045179709987,8.40164026751102));
#37461=CARTESIAN_POINT('Ctrl Pts',(7.27603390513757,-48.2295179709986,4.2008201337472));
#37462=CARTESIAN_POINT('Ctrl Pts',(9.70137854017372,-48.0545179709987,-1.69906585035305E-11));
#37463=CARTESIAN_POINT('Ctrl Pts',(7.27603390512286,-47.8795179709987,-4.20082013377268));
#37464=CARTESIAN_POINT('Ctrl Pts',(5.65116042235429,-47.7622757220518,-7.015183561788));
#37465=CARTESIAN_POINT('Ctrl Pts',(2.55537495509676,-47.63,-8.00360031633711));
#37466=CARTESIAN_POINT('Ctrl Pts',(-5.67113674141202,-212.63,6.1988520909128));
#37467=CARTESIAN_POINT('Ctrl Pts',(-5.09309959239855,-212.63,6.65024148625226));
#37468=CARTESIAN_POINT('Ctrl Pts',(-4.1369669254735,-212.630000000009,7.33153862293111));
#37469=CARTESIAN_POINT('Ctrl Pts',(-1.84049420638942,-212.630000000009,
8.10711214912164));
#37470=CARTESIAN_POINT('Ctrl Pts',(-0.84190354263217,-212.63,8.26396636048523));
#37471=CARTESIAN_POINT('Ctrl Pts',(1.15691725446766,-212.63,8.22412665653735));
#37472=CARTESIAN_POINT('Ctrl Pts',(2.13751792446255,-212.63,8.03230830225828));
#37473=CARTESIAN_POINT('Ctrl Pts',(4.40951680002617,-212.63,7.1736078615634));
#37474=CARTESIAN_POINT('Ctrl Pts',(5.3486773581226,-212.63,6.44726429217888));
#37475=CARTESIAN_POINT('Ctrl Pts',(5.91264939824166,-212.63,5.96893091585754));
#37476=CARTESIAN_POINT('Ctrl Pts',(-1.51301075899711E-11,-213.429517970998,
-8.40164026751963));
#37477=CARTESIAN_POINT('Ctrl Pts',(-4.85068927010199,-213.254517970998,
-8.4016402675109));
#37478=CARTESIAN_POINT('Ctrl Pts',(-7.27603390513785,-213.079517970998,
-4.20082013374671));
#37479=CARTESIAN_POINT('Ctrl Pts',(-9.70137854017372,-212.904517970998,
1.74701493417668E-11));
#37480=CARTESIAN_POINT('Ctrl Pts',(-7.27603390512272,-212.729517970998,
4.20082013377292));
#37481=CARTESIAN_POINT('Ctrl Pts',(-4.85068927007173,-212.554517970998,
8.40164026752836));
#37482=CARTESIAN_POINT('Ctrl Pts',(1.5129078685785E-11,-212.379517970998,
8.40164026751963));
#37483=CARTESIAN_POINT('Ctrl Pts',(4.85068927010198,-212.204517970998,8.4016402675109));
#37484=CARTESIAN_POINT('Ctrl Pts',(7.27603390513785,-212.029517970998,4.20082013374672));
#37485=CARTESIAN_POINT('Ctrl Pts',(9.70137854017372,-211.854517970998,-1.74689612655491E-11));
#37486=CARTESIAN_POINT('Ctrl Pts',(7.27603390512273,-211.679517970998,-4.20082013377291));
#37487=CARTESIAN_POINT('Ctrl Pts',(4.85068927007173,-211.504517970998,-8.40164026752836));
#37488=CARTESIAN_POINT('Ctrl Pts',(-1.51301075899711E-11,-211.329517970998,
-8.40164026751963));
#37489=CARTESIAN_POINT('Ctrl Pts',(-4.85068927010199,-211.154517970998,
-8.4016402675109));
#37490=CARTESIAN_POINT('Ctrl Pts',(-7.27603390513785,-210.979517970998,
-4.20082013374671));
#37491=CARTESIAN_POINT('Ctrl Pts',(-9.70137854017372,-210.804517970998,
1.74701493417668E-11));
#37492=CARTESIAN_POINT('Ctrl Pts',(-7.27603390512272,-210.629517970998,
4.20082013377292));
#37493=CARTESIAN_POINT('Ctrl Pts',(-4.85068927007173,-210.454517970998,
8.40164026752836));
#37494=CARTESIAN_POINT('Ctrl Pts',(1.5129078685785E-11,-210.279517970998,
8.40164026751963));
#37495=CARTESIAN_POINT('Ctrl Pts',(4.85068927010198,-210.104517970998,8.4016402675109));
#37496=CARTESIAN_POINT('Ctrl Pts',(7.27603390513785,-209.929517970998,4.20082013374672));
#37497=CARTESIAN_POINT('Ctrl Pts',(9.70137854017372,-209.754517970998,-1.74689612655491E-11));
#37498=CARTESIAN_POINT('Ctrl Pts',(7.27603390512273,-209.579517970998,-4.20082013377291));
#37499=CARTESIAN_POINT('Ctrl Pts',(4.85068927007173,-209.404517970998,-8.40164026752836));
#37500=CARTESIAN_POINT('Ctrl Pts',(-1.51301075899711E-11,-209.229517970998,
-8.40164026751963));
#37501=CARTESIAN_POINT('Ctrl Pts',(-4.85068927010199,-209.054517970998,
-8.4016402675109));
#37502=CARTESIAN_POINT('Ctrl Pts',(-7.27603390513785,-208.879517970998,
-4.20082013374671));
#37503=CARTESIAN_POINT('Ctrl Pts',(-9.70137854017372,-208.704517970998,
1.74701493417668E-11));
#37504=CARTESIAN_POINT('Ctrl Pts',(-7.27603390512272,-208.529517970998,
4.20082013377292));
#37505=CARTESIAN_POINT('Ctrl Pts',(-4.85068927007173,-208.354517970998,
8.40164026752836));
#37506=CARTESIAN_POINT('Ctrl Pts',(1.5129078685785E-11,-208.179517970998,
8.40164026751963));
#37507=CARTESIAN_POINT('Ctrl Pts',(4.85068927010198,-208.004517970998,8.4016402675109));
#37508=CARTESIAN_POINT('Ctrl Pts',(7.27603390513785,-207.829517970998,4.20082013374672));
#37509=CARTESIAN_POINT('Ctrl Pts',(9.70137854017372,-207.654517970998,-1.74689612655491E-11));
#37510=CARTESIAN_POINT('Ctrl Pts',(7.27603390512273,-207.479517970998,-4.20082013377291));
#37511=CARTESIAN_POINT('Ctrl Pts',(4.85068927007173,-207.304517970998,-8.40164026752836));
#37512=CARTESIAN_POINT('Ctrl Pts',(-1.51301075899711E-11,-207.129517970998,
-8.40164026751963));
#37513=CARTESIAN_POINT('Ctrl Pts',(-4.85068927010199,-206.954517970998,
-8.4016402675109));
#37514=CARTESIAN_POINT('Ctrl Pts',(-7.27603390513785,-206.779517970998,
-4.20082013374671));
#37515=CARTESIAN_POINT('Ctrl Pts',(-9.70137854017372,-206.604517970998,
1.74701493417668E-11));
#37516=CARTESIAN_POINT('Ctrl Pts',(-7.27603390512272,-206.429517970998,
4.20082013377292));
#37517=CARTESIAN_POINT('Ctrl Pts',(-4.85068927007173,-206.254517970998,
8.40164026752836));
#37518=CARTESIAN_POINT('Ctrl Pts',(1.5129078685785E-11,-206.079517970998,
8.40164026751963));
#37519=CARTESIAN_POINT('Ctrl Pts',(4.85068927010198,-205.904517970998,8.4016402675109));
#37520=CARTESIAN_POINT('Ctrl Pts',(7.27603390513785,-205.729517970998,4.20082013374672));
#37521=CARTESIAN_POINT('Ctrl Pts',(9.70137854017372,-205.554517970998,-1.74689612655491E-11));
#37522=CARTESIAN_POINT('Ctrl Pts',(7.27603390512273,-205.379517970998,-4.20082013377291));
#37523=CARTESIAN_POINT('Ctrl Pts',(4.85068927007173,-205.204517970998,-8.40164026752836));
#37524=CARTESIAN_POINT('Ctrl Pts',(-1.51301075899711E-11,-205.029517970998,
-8.40164026751963));
#37525=CARTESIAN_POINT('Ctrl Pts',(-4.85068927010199,-204.854517970998,
-8.4016402675109));
#37526=CARTESIAN_POINT('Ctrl Pts',(-7.27603390513785,-204.679517970998,
-4.20082013374671));
#37527=CARTESIAN_POINT('Ctrl Pts',(-9.70137854017372,-204.504517970998,
1.74701493417668E-11));
#37528=CARTESIAN_POINT('Ctrl Pts',(-7.27603390512272,-204.329517970998,
4.20082013377292));
#37529=CARTESIAN_POINT('Ctrl Pts',(-4.85068927007173,-204.154517970998,
8.40164026752836));
#37530=CARTESIAN_POINT('Ctrl Pts',(1.5129078685785E-11,-203.979517970998,
8.40164026751963));
#37531=CARTESIAN_POINT('Ctrl Pts',(4.85068927010198,-203.804517970998,8.4016402675109));
#37532=CARTESIAN_POINT('Ctrl Pts',(7.27603390513785,-203.629517970998,4.20082013374672));
#37533=CARTESIAN_POINT('Ctrl Pts',(9.70137854017372,-203.454517970998,-1.74689612655491E-11));
#37534=CARTESIAN_POINT('Ctrl Pts',(7.27603390512273,-203.279517970998,-4.20082013377291));
#37535=CARTESIAN_POINT('Ctrl Pts',(4.85068927007173,-203.104517970998,-8.40164026752836));
#37536=CARTESIAN_POINT('Ctrl Pts',(-1.51301075899711E-11,-202.929517970998,
-8.40164026751963));
#37537=CARTESIAN_POINT('Ctrl Pts',(-4.85068927010199,-202.754517970998,
-8.4016402675109));
#37538=CARTESIAN_POINT('Ctrl Pts',(-7.27603390513785,-202.579517970998,
-4.20082013374671));
#37539=CARTESIAN_POINT('Ctrl Pts',(-9.70137854017372,-202.404517970998,
1.74701493417668E-11));
#37540=CARTESIAN_POINT('Ctrl Pts',(-7.27603390512272,-202.229517970998,
4.20082013377292));
#37541=CARTESIAN_POINT('Ctrl Pts',(-4.85068927007173,-202.054517970998,
8.40164026752836));
#37542=CARTESIAN_POINT('Ctrl Pts',(1.5129078685785E-11,-201.879517970998,
8.40164026751963));
#37543=CARTESIAN_POINT('Ctrl Pts',(4.85068927010198,-201.704517970998,8.4016402675109));
#37544=CARTESIAN_POINT('Ctrl Pts',(7.27603390513785,-201.529517970998,4.20082013374672));
#37545=CARTESIAN_POINT('Ctrl Pts',(9.70137854017372,-201.354517970998,-1.74689612655491E-11));
#37546=CARTESIAN_POINT('Ctrl Pts',(7.27603390512273,-201.179517970998,-4.20082013377291));
#37547=CARTESIAN_POINT('Ctrl Pts',(4.85068927007173,-201.004517970998,-8.40164026752836));
#37548=CARTESIAN_POINT('Ctrl Pts',(-1.51301075899711E-11,-200.829517970998,
-8.40164026751963));
#37549=CARTESIAN_POINT('Ctrl Pts',(-4.85068927010199,-200.654517970998,
-8.4016402675109));
#37550=CARTESIAN_POINT('Ctrl Pts',(-7.27603390513785,-200.479517970998,
-4.20082013374671));
#37551=CARTESIAN_POINT('Ctrl Pts',(-9.70137854017372,-200.304517970998,
1.74701493417668E-11));
#37552=CARTESIAN_POINT('Ctrl Pts',(-7.27603390512272,-200.129517970998,
4.20082013377292));
#37553=CARTESIAN_POINT('Ctrl Pts',(-4.85068927007173,-199.954517970998,
8.40164026752836));
#37554=CARTESIAN_POINT('Ctrl Pts',(1.5129078685785E-11,-199.779517970998,
8.40164026751963));
#37555=CARTESIAN_POINT('Ctrl Pts',(4.85068927010198,-199.604517970998,8.4016402675109));
#37556=CARTESIAN_POINT('Ctrl Pts',(7.27603390513785,-199.429517970998,4.20082013374672));
#37557=CARTESIAN_POINT('Ctrl Pts',(9.70137854017372,-199.254517970998,-1.74689612655491E-11));
#37558=CARTESIAN_POINT('Ctrl Pts',(7.27603390512273,-199.079517970998,-4.20082013377291));
#37559=CARTESIAN_POINT('Ctrl Pts',(4.85068927007173,-198.904517970998,-8.40164026752836));
#37560=CARTESIAN_POINT('Ctrl Pts',(-1.51301075899711E-11,-198.729517970998,
-8.40164026751963));
#37561=CARTESIAN_POINT('Ctrl Pts',(-4.85068927010199,-198.554517970998,
-8.4016402675109));
#37562=CARTESIAN_POINT('Ctrl Pts',(-7.27603390513785,-198.379517970998,
-4.20082013374671));
#37563=CARTESIAN_POINT('Ctrl Pts',(-9.70137854017372,-198.204517970998,
1.74701493417668E-11));
#37564=CARTESIAN_POINT('Ctrl Pts',(-7.27603390512272,-198.029517970998,
4.20082013377292));
#37565=CARTESIAN_POINT('Ctrl Pts',(-4.85068927007173,-197.854517970998,
8.40164026752836));
#37566=CARTESIAN_POINT('Ctrl Pts',(1.5129078685785E-11,-197.679517970998,
8.40164026751963));
#37567=CARTESIAN_POINT('Ctrl Pts',(4.85068927010198,-197.504517970998,8.4016402675109));
#37568=CARTESIAN_POINT('Ctrl Pts',(7.27603390513785,-197.329517970998,4.20082013374672));
#37569=CARTESIAN_POINT('Ctrl Pts',(9.70137854017372,-197.154517970998,-1.74689612655491E-11));
#37570=CARTESIAN_POINT('Ctrl Pts',(7.27603390512273,-196.979517970998,-4.20082013377291));
#37571=CARTESIAN_POINT('Ctrl Pts',(4.85068927007173,-196.804517970998,-8.40164026752836));
#37572=CARTESIAN_POINT('Ctrl Pts',(-1.51301075899711E-11,-196.629517970998,
-8.40164026751963));
#37573=CARTESIAN_POINT('Ctrl Pts',(-4.85068927010199,-196.454517970998,
-8.4016402675109));
#37574=CARTESIAN_POINT('Ctrl Pts',(-7.27603390513785,-196.279517970998,
-4.20082013374671));
#37575=CARTESIAN_POINT('Ctrl Pts',(-9.70137854017372,-196.104517970998,
1.74701493417668E-11));
#37576=CARTESIAN_POINT('Ctrl Pts',(-7.27603390512272,-195.929517970998,
4.20082013377292));
#37577=CARTESIAN_POINT('Ctrl Pts',(-4.85068927007173,-195.754517970998,
8.40164026752836));
#37578=CARTESIAN_POINT('Ctrl Pts',(1.5129078685785E-11,-195.579517970998,
8.40164026751963));
#37579=CARTESIAN_POINT('Ctrl Pts',(4.85068927010198,-195.404517970998,8.4016402675109));
#37580=CARTESIAN_POINT('Ctrl Pts',(7.27603390513785,-195.229517970998,4.20082013374672));
#37581=CARTESIAN_POINT('Ctrl Pts',(9.70137854017372,-195.054517970998,-1.74689612655491E-11));
#37582=CARTESIAN_POINT('Ctrl Pts',(7.27603390512273,-194.879517970998,-4.20082013377291));
#37583=CARTESIAN_POINT('Ctrl Pts',(4.85068927007173,-194.704517970998,-8.40164026752836));
#37584=CARTESIAN_POINT('Ctrl Pts',(-1.51301075899711E-11,-194.529517970998,
-8.40164026751963));
#37585=CARTESIAN_POINT('Ctrl Pts',(-4.85068927010199,-194.354517970998,
-8.4016402675109));
#37586=CARTESIAN_POINT('Ctrl Pts',(-7.27603390513785,-194.179517970998,
-4.20082013374671));
#37587=CARTESIAN_POINT('Ctrl Pts',(-9.70137854017372,-194.004517970998,
1.74701493417668E-11));
#37588=CARTESIAN_POINT('Ctrl Pts',(-7.27603390512272,-193.829517970998,
4.20082013377292));
#37589=CARTESIAN_POINT('Ctrl Pts',(-4.85068927007173,-193.654517970998,
8.40164026752836));
#37590=CARTESIAN_POINT('Ctrl Pts',(1.5129078685785E-11,-193.479517970998,
8.40164026751963));
#37591=CARTESIAN_POINT('Ctrl Pts',(4.85068927010198,-193.304517970998,8.4016402675109));
#37592=CARTESIAN_POINT('Ctrl Pts',(7.27603390513785,-193.129517970998,4.20082013374672));
#37593=CARTESIAN_POINT('Ctrl Pts',(9.70137854017372,-192.954517970998,-1.74689612655491E-11));
#37594=CARTESIAN_POINT('Ctrl Pts',(7.27603390512273,-192.779517970998,-4.20082013377291));
#37595=CARTESIAN_POINT('Ctrl Pts',(4.85068927007173,-192.604517970998,-8.40164026752836));
#37596=CARTESIAN_POINT('Ctrl Pts',(-1.51301075899711E-11,-192.429517970998,
-8.40164026751963));
#37597=CARTESIAN_POINT('Ctrl Pts',(-4.85068927010199,-192.254517970998,
-8.4016402675109));
#37598=CARTESIAN_POINT('Ctrl Pts',(-7.27603390513785,-192.079517970998,
-4.20082013374671));
#37599=CARTESIAN_POINT('Ctrl Pts',(-9.70137854017372,-191.904517970998,
1.74701493417668E-11));
#37600=CARTESIAN_POINT('Ctrl Pts',(-7.27603390512272,-191.729517970998,
4.20082013377292));
#37601=CARTESIAN_POINT('Ctrl Pts',(-4.85068927007173,-191.554517970998,
8.40164026752836));
#37602=CARTESIAN_POINT('Ctrl Pts',(1.5129078685785E-11,-191.379517970998,
8.40164026751963));
#37603=CARTESIAN_POINT('Ctrl Pts',(4.85068927010198,-191.204517970998,8.4016402675109));
#37604=CARTESIAN_POINT('Ctrl Pts',(7.27603390513785,-191.029517970998,4.20082013374672));
#37605=CARTESIAN_POINT('Ctrl Pts',(9.70137854017372,-190.854517970998,-1.74689612655491E-11));
#37606=CARTESIAN_POINT('Ctrl Pts',(7.27603390512273,-190.679517970998,-4.20082013377291));
#37607=CARTESIAN_POINT('Ctrl Pts',(4.85068927007173,-190.504517970998,-8.40164026752836));
#37608=CARTESIAN_POINT('Ctrl Pts',(-1.51301075899711E-11,-190.329517970998,
-8.40164026751963));
#37609=CARTESIAN_POINT('Ctrl Pts',(-4.85068927010199,-190.154517970998,
-8.4016402675109));
#37610=CARTESIAN_POINT('Ctrl Pts',(-7.27603390513785,-189.979517970998,
-4.20082013374671));
#37611=CARTESIAN_POINT('Ctrl Pts',(-9.70137854017372,-189.804517970998,
1.74701493417668E-11));
#37612=CARTESIAN_POINT('Ctrl Pts',(-7.27603390512272,-189.629517970998,
4.20082013377292));
#37613=CARTESIAN_POINT('Ctrl Pts',(-4.85068927007173,-189.454517970998,
8.40164026752836));
#37614=CARTESIAN_POINT('Ctrl Pts',(1.5129078685785E-11,-189.279517970998,
8.40164026751963));
#37615=CARTESIAN_POINT('Ctrl Pts',(4.85068927010198,-189.104517970998,8.4016402675109));
#37616=CARTESIAN_POINT('Ctrl Pts',(7.27603390513785,-188.929517970998,4.20082013374672));
#37617=CARTESIAN_POINT('Ctrl Pts',(9.70137854017372,-188.754517970998,-1.74689612655491E-11));
#37618=CARTESIAN_POINT('Ctrl Pts',(7.27603390512273,-188.579517970998,-4.20082013377291));
#37619=CARTESIAN_POINT('Ctrl Pts',(4.85068927007173,-188.404517970998,-8.40164026752836));
#37620=CARTESIAN_POINT('Ctrl Pts',(-1.51301075899711E-11,-188.229517970998,
-8.40164026751963));
#37621=CARTESIAN_POINT('Ctrl Pts',(-4.85068927010199,-188.054517970998,
-8.4016402675109));
#37622=CARTESIAN_POINT('Ctrl Pts',(-7.27603390513785,-187.879517970998,
-4.20082013374671));
#37623=CARTESIAN_POINT('Ctrl Pts',(-9.70137854017372,-187.704517970998,
1.74701493417668E-11));
#37624=CARTESIAN_POINT('Ctrl Pts',(-7.27603390512272,-187.529517970998,
4.20082013377292));
#37625=CARTESIAN_POINT('Ctrl Pts',(-4.85068927007173,-187.354517970998,
8.40164026752836));
#37626=CARTESIAN_POINT('Ctrl Pts',(1.5129078685785E-11,-187.179517970998,
8.40164026751963));
#37627=CARTESIAN_POINT('Ctrl Pts',(4.85068927010198,-187.004517970998,8.4016402675109));
#37628=CARTESIAN_POINT('Ctrl Pts',(7.27603390513785,-186.829517970998,4.20082013374672));
#37629=CARTESIAN_POINT('Ctrl Pts',(9.70137854017372,-186.654517970998,-1.74689612655491E-11));
#37630=CARTESIAN_POINT('Ctrl Pts',(7.27603390512273,-186.479517970998,-4.20082013377291));
#37631=CARTESIAN_POINT('Ctrl Pts',(4.85068927007173,-186.304517970998,-8.40164026752836));
#37632=CARTESIAN_POINT('Ctrl Pts',(-1.51301075899711E-11,-186.129517970998,
-8.40164026751963));
#37633=CARTESIAN_POINT('Ctrl Pts',(-4.85068927010199,-185.954517970998,
-8.4016402675109));
#37634=CARTESIAN_POINT('Ctrl Pts',(-7.27603390513785,-185.779517970998,
-4.20082013374671));
#37635=CARTESIAN_POINT('Ctrl Pts',(-9.70137854017372,-185.604517970998,
1.74701493417668E-11));
#37636=CARTESIAN_POINT('Ctrl Pts',(-7.27603390512272,-185.429517970998,
4.20082013377292));
#37637=CARTESIAN_POINT('Ctrl Pts',(-4.85068927007173,-185.254517970998,
8.40164026752836));
#37638=CARTESIAN_POINT('Ctrl Pts',(1.5129078685785E-11,-185.079517970998,
8.40164026751963));
#37639=CARTESIAN_POINT('Ctrl Pts',(4.85068927010198,-184.904517970998,8.4016402675109));
#37640=CARTESIAN_POINT('Ctrl Pts',(7.27603390513785,-184.729517970998,4.20082013374672));
#37641=CARTESIAN_POINT('Ctrl Pts',(9.70137854017372,-184.554517970998,-1.74689612655491E-11));
#37642=CARTESIAN_POINT('Ctrl Pts',(7.27603390512273,-184.379517970998,-4.20082013377291));
#37643=CARTESIAN_POINT('Ctrl Pts',(4.85068927007173,-184.204517970998,-8.40164026752836));
#37644=CARTESIAN_POINT('Ctrl Pts',(-1.51301075899711E-11,-184.029517970998,
-8.40164026751963));
#37645=CARTESIAN_POINT('Ctrl Pts',(-4.85068927010199,-183.854517970998,
-8.4016402675109));
#37646=CARTESIAN_POINT('Ctrl Pts',(-7.27603390513785,-183.679517970998,
-4.20082013374671));
#37647=CARTESIAN_POINT('Ctrl Pts',(-9.70137854017372,-183.504517970998,
1.74701493417668E-11));
#37648=CARTESIAN_POINT('Ctrl Pts',(-7.27603390512272,-183.329517970998,
4.20082013377292));
#37649=CARTESIAN_POINT('Ctrl Pts',(-4.85068927007173,-183.154517970998,
8.40164026752836));
#37650=CARTESIAN_POINT('Ctrl Pts',(1.5129078685785E-11,-182.979517970998,
8.40164026751963));
#37651=CARTESIAN_POINT('Ctrl Pts',(4.85068927010198,-182.804517970998,8.4016402675109));
#37652=CARTESIAN_POINT('Ctrl Pts',(7.27603390513785,-182.629517970998,4.20082013374672));
#37653=CARTESIAN_POINT('Ctrl Pts',(9.70137854017372,-182.454517970998,-1.74689612655491E-11));
#37654=CARTESIAN_POINT('Ctrl Pts',(7.27603390512273,-182.279517970998,-4.20082013377291));
#37655=CARTESIAN_POINT('Ctrl Pts',(4.85068927007173,-182.104517970998,-8.40164026752836));
#37656=CARTESIAN_POINT('Ctrl Pts',(-1.51301075899711E-11,-181.929517970998,
-8.40164026751963));
#37657=CARTESIAN_POINT('Ctrl Pts',(-4.85068927010199,-181.754517970998,
-8.4016402675109));
#37658=CARTESIAN_POINT('Ctrl Pts',(-7.27603390513785,-181.579517970998,
-4.20082013374671));
#37659=CARTESIAN_POINT('Ctrl Pts',(-9.70137854017372,-181.404517970998,
1.74701493417668E-11));
#37660=CARTESIAN_POINT('Ctrl Pts',(-7.27603390512272,-181.229517970998,
4.20082013377292));
#37661=CARTESIAN_POINT('Ctrl Pts',(-4.85068927007173,-181.054517970998,
8.40164026752836));
#37662=CARTESIAN_POINT('Ctrl Pts',(1.5129078685785E-11,-180.879517970998,
8.40164026751963));
#37663=CARTESIAN_POINT('Ctrl Pts',(4.85068927010198,-180.704517970998,8.4016402675109));
#37664=CARTESIAN_POINT('Ctrl Pts',(7.27603390513785,-180.529517970998,4.20082013374672));
#37665=CARTESIAN_POINT('Ctrl Pts',(9.70137854017372,-180.354517970998,-1.74689612655491E-11));
#37666=CARTESIAN_POINT('Ctrl Pts',(7.27603390512273,-180.179517970998,-4.20082013377291));
#37667=CARTESIAN_POINT('Ctrl Pts',(4.85068927007173,-180.004517970998,-8.40164026752836));
#37668=CARTESIAN_POINT('Ctrl Pts',(-1.51301075899711E-11,-179.829517970998,
-8.40164026751963));
#37669=CARTESIAN_POINT('Ctrl Pts',(-4.85068927010199,-179.654517970998,
-8.4016402675109));
#37670=CARTESIAN_POINT('Ctrl Pts',(-7.27603390513785,-179.479517970998,
-4.20082013374671));
#37671=CARTESIAN_POINT('Ctrl Pts',(-9.70137854017372,-179.304517970998,
1.74701493417668E-11));
#37672=CARTESIAN_POINT('Ctrl Pts',(-7.27603390512272,-179.129517970998,
4.20082013377292));
#37673=CARTESIAN_POINT('Ctrl Pts',(-4.85068927007173,-178.954517970998,
8.40164026752836));
#37674=CARTESIAN_POINT('Ctrl Pts',(1.5129078685785E-11,-178.779517970998,
8.40164026751963));
#37675=CARTESIAN_POINT('Ctrl Pts',(4.85068927010198,-178.604517970998,8.4016402675109));
#37676=CARTESIAN_POINT('Ctrl Pts',(7.27603390513785,-178.429517970998,4.20082013374672));
#37677=CARTESIAN_POINT('Ctrl Pts',(9.70137854017372,-178.254517970998,-1.74689612655491E-11));
#37678=CARTESIAN_POINT('Ctrl Pts',(7.27603390512273,-178.079517970998,-4.20082013377291));
#37679=CARTESIAN_POINT('Ctrl Pts',(4.85068927007173,-177.904517970998,-8.40164026752836));
#37680=CARTESIAN_POINT('Ctrl Pts',(-1.51301075899711E-11,-177.729517970998,
-8.40164026751963));
#37681=CARTESIAN_POINT('Ctrl Pts',(-4.85068927010199,-177.554517970998,
-8.4016402675109));
#37682=CARTESIAN_POINT('Ctrl Pts',(-7.27603390513785,-177.379517970998,
-4.20082013374671));
#37683=CARTESIAN_POINT('Ctrl Pts',(-9.70137854017372,-177.204517970998,
1.74701493417668E-11));
#37684=CARTESIAN_POINT('Ctrl Pts',(-7.27603390512272,-177.029517970998,
4.20082013377292));
#37685=CARTESIAN_POINT('Ctrl Pts',(-4.85068927007173,-176.854517970998,
8.40164026752836));
#37686=CARTESIAN_POINT('Ctrl Pts',(1.5129078685785E-11,-176.679517970998,
8.40164026751963));
#37687=CARTESIAN_POINT('Ctrl Pts',(4.85068927010198,-176.504517970998,8.4016402675109));
#37688=CARTESIAN_POINT('Ctrl Pts',(7.27603390513785,-176.329517970998,4.20082013374672));
#37689=CARTESIAN_POINT('Ctrl Pts',(9.70137854017372,-176.154517970998,-1.74689612655491E-11));
#37690=CARTESIAN_POINT('Ctrl Pts',(7.27603390512273,-175.979517970998,-4.20082013377291));
#37691=CARTESIAN_POINT('Ctrl Pts',(4.85068927007173,-175.804517970998,-8.40164026752836));
#37692=CARTESIAN_POINT('Ctrl Pts',(-1.51301075899711E-11,-175.629517970998,
-8.40164026751963));
#37693=CARTESIAN_POINT('Ctrl Pts',(-4.85068927010199,-175.454517970998,
-8.4016402675109));
#37694=CARTESIAN_POINT('Ctrl Pts',(-7.27603390513785,-175.279517970998,
-4.20082013374671));
#37695=CARTESIAN_POINT('Ctrl Pts',(-9.70137854017372,-175.104517970998,
1.74701493417668E-11));
#37696=CARTESIAN_POINT('Ctrl Pts',(-7.27603390512272,-174.929517970998,
4.20082013377292));
#37697=CARTESIAN_POINT('Ctrl Pts',(-4.85068927007173,-174.754517970998,
8.40164026752836));
#37698=CARTESIAN_POINT('Ctrl Pts',(1.5129078685785E-11,-174.579517970998,
8.40164026751963));
#37699=CARTESIAN_POINT('Ctrl Pts',(4.85068927010198,-174.404517970998,8.4016402675109));
#37700=CARTESIAN_POINT('Ctrl Pts',(7.27603390513785,-174.229517970998,4.20082013374672));
#37701=CARTESIAN_POINT('Ctrl Pts',(9.70137854017372,-174.054517970998,-1.74689612655491E-11));
#37702=CARTESIAN_POINT('Ctrl Pts',(7.27603390512273,-173.879517970998,-4.20082013377291));
#37703=CARTESIAN_POINT('Ctrl Pts',(4.85068927007173,-173.704517970998,-8.40164026752836));
#37704=CARTESIAN_POINT('Ctrl Pts',(-1.51301075899711E-11,-173.529517970998,
-8.40164026751963));
#37705=CARTESIAN_POINT('Ctrl Pts',(-4.85068927010199,-173.354517970998,
-8.4016402675109));
#37706=CARTESIAN_POINT('Ctrl Pts',(-7.27603390513785,-173.179517970998,
-4.20082013374671));
#37707=CARTESIAN_POINT('Ctrl Pts',(-9.70137854017372,-173.004517970998,
1.74701493417668E-11));
#37708=CARTESIAN_POINT('Ctrl Pts',(-7.27603390512272,-172.829517970998,
4.20082013377292));
#37709=CARTESIAN_POINT('Ctrl Pts',(-4.85068927007173,-172.654517970998,
8.40164026752836));
#37710=CARTESIAN_POINT('Ctrl Pts',(1.5129078685785E-11,-172.479517970998,
8.40164026751963));
#37711=CARTESIAN_POINT('Ctrl Pts',(4.85068927010198,-172.304517970998,8.4016402675109));
#37712=CARTESIAN_POINT('Ctrl Pts',(7.27603390513785,-172.129517970998,4.20082013374672));
#37713=CARTESIAN_POINT('Ctrl Pts',(9.70137854017372,-171.954517970998,-1.74689612655491E-11));
#37714=CARTESIAN_POINT('Ctrl Pts',(7.27603390512273,-171.779517970998,-4.20082013377291));
#37715=CARTESIAN_POINT('Ctrl Pts',(4.85068927007173,-171.604517970998,-8.40164026752836));
#37716=CARTESIAN_POINT('Ctrl Pts',(-1.51301075899711E-11,-171.429517970998,
-8.40164026751963));
#37717=CARTESIAN_POINT('Ctrl Pts',(-4.85068927010199,-171.254517970998,
-8.4016402675109));
#37718=CARTESIAN_POINT('Ctrl Pts',(-7.27603390513785,-171.079517970998,
-4.20082013374671));
#37719=CARTESIAN_POINT('Ctrl Pts',(-9.70137854017372,-170.904517970998,
1.74701493417668E-11));
#37720=CARTESIAN_POINT('Ctrl Pts',(-7.27603390512272,-170.729517970998,
4.20082013377292));
#37721=CARTESIAN_POINT('Ctrl Pts',(-4.85068927007173,-170.554517970998,
8.40164026752836));
#37722=CARTESIAN_POINT('Ctrl Pts',(1.5129078685785E-11,-170.379517970998,
8.40164026751963));
#37723=CARTESIAN_POINT('Ctrl Pts',(4.85068927010198,-170.204517970998,8.4016402675109));
#37724=CARTESIAN_POINT('Ctrl Pts',(7.27603390513785,-170.029517970998,4.20082013374672));
#37725=CARTESIAN_POINT('Ctrl Pts',(9.70137854017372,-169.854517970998,-1.74689612655491E-11));
#37726=CARTESIAN_POINT('Ctrl Pts',(7.27603390512273,-169.679517970998,-4.20082013377291));
#37727=CARTESIAN_POINT('Ctrl Pts',(4.85068927007173,-169.504517970998,-8.40164026752836));
#37728=CARTESIAN_POINT('Ctrl Pts',(-1.51301075899711E-11,-169.329517970998,
-8.40164026751963));
#37729=CARTESIAN_POINT('Ctrl Pts',(-4.85068927010199,-169.154517970998,
-8.4016402675109));
#37730=CARTESIAN_POINT('Ctrl Pts',(-7.27603390513785,-168.979517970998,
-4.20082013374671));
#37731=CARTESIAN_POINT('Ctrl Pts',(-9.70137854017372,-168.804517970998,
1.74701493417668E-11));
#37732=CARTESIAN_POINT('Ctrl Pts',(-7.27603390512272,-168.629517970998,
4.20082013377292));
#37733=CARTESIAN_POINT('Ctrl Pts',(-4.85068927007173,-168.454517970998,
8.40164026752836));
#37734=CARTESIAN_POINT('Ctrl Pts',(1.5129078685785E-11,-168.279517970998,
8.40164026751963));
#37735=CARTESIAN_POINT('Ctrl Pts',(4.85068927010198,-168.104517970998,8.4016402675109));
#37736=CARTESIAN_POINT('Ctrl Pts',(7.27603390513785,-167.929517970998,4.20082013374672));
#37737=CARTESIAN_POINT('Ctrl Pts',(9.70137854017372,-167.754517970998,-1.74689612655491E-11));
#37738=CARTESIAN_POINT('Ctrl Pts',(7.27603390512273,-167.579517970998,-4.20082013377291));
#37739=CARTESIAN_POINT('Ctrl Pts',(4.85068927007173,-167.404517970998,-8.40164026752836));
#37740=CARTESIAN_POINT('Ctrl Pts',(-1.51301075899711E-11,-167.229517970998,
-8.40164026751963));
#37741=CARTESIAN_POINT('Ctrl Pts',(-4.85068927010199,-167.054517970998,
-8.4016402675109));
#37742=CARTESIAN_POINT('Ctrl Pts',(-7.27603390513785,-166.879517970998,
-4.20082013374671));
#37743=CARTESIAN_POINT('Ctrl Pts',(-9.70137854017372,-166.704517970998,
1.74701493417668E-11));
#37744=CARTESIAN_POINT('Ctrl Pts',(-7.27603390512272,-166.529517970998,
4.20082013377292));
#37745=CARTESIAN_POINT('Ctrl Pts',(-4.85068927007173,-166.354517970998,
8.40164026752836));
#37746=CARTESIAN_POINT('Ctrl Pts',(1.5129078685785E-11,-166.179517970998,
8.40164026751963));
#37747=CARTESIAN_POINT('Ctrl Pts',(4.85068927010198,-166.004517970998,8.4016402675109));
#37748=CARTESIAN_POINT('Ctrl Pts',(7.27603390513785,-165.829517970998,4.20082013374672));
#37749=CARTESIAN_POINT('Ctrl Pts',(9.70137854017372,-165.654517970998,-1.74689612655491E-11));
#37750=CARTESIAN_POINT('Ctrl Pts',(7.27603390512273,-165.479517970998,-4.20082013377291));
#37751=CARTESIAN_POINT('Ctrl Pts',(4.85068927007173,-165.304517970998,-8.40164026752836));
#37752=CARTESIAN_POINT('Ctrl Pts',(-1.51301075899711E-11,-165.129517970998,
-8.40164026751963));
#37753=CARTESIAN_POINT('Ctrl Pts',(-4.85068927010199,-164.954517970998,
-8.4016402675109));
#37754=CARTESIAN_POINT('Ctrl Pts',(-7.27603390513785,-164.779517970998,
-4.20082013374671));
#37755=CARTESIAN_POINT('Ctrl Pts',(-9.70137854017372,-164.604517970998,
1.74701493417668E-11));
#37756=CARTESIAN_POINT('Ctrl Pts',(-7.27603390512272,-164.429517970998,
4.20082013377292));
#37757=CARTESIAN_POINT('Ctrl Pts',(-4.85068927007173,-164.254517970998,
8.40164026752836));
#37758=CARTESIAN_POINT('Ctrl Pts',(1.5129078685785E-11,-164.079517970998,
8.40164026751963));
#37759=CARTESIAN_POINT('Ctrl Pts',(4.85068927010198,-163.904517970998,8.4016402675109));
#37760=CARTESIAN_POINT('Ctrl Pts',(7.27603390513785,-163.729517970998,4.20082013374672));
#37761=CARTESIAN_POINT('Ctrl Pts',(9.70137854017372,-163.554517970998,-1.74689612655491E-11));
#37762=CARTESIAN_POINT('Ctrl Pts',(7.27603390512273,-163.379517970998,-4.20082013377291));
#37763=CARTESIAN_POINT('Ctrl Pts',(4.85068927007173,-163.204517970998,-8.40164026752836));
#37764=CARTESIAN_POINT('Ctrl Pts',(-1.51301075899711E-11,-163.029517970998,
-8.40164026751963));
#37765=CARTESIAN_POINT('Ctrl Pts',(-4.85068927010199,-162.854517970998,
-8.4016402675109));
#37766=CARTESIAN_POINT('Ctrl Pts',(-7.27603390513785,-162.679517970998,
-4.20082013374671));
#37767=CARTESIAN_POINT('Ctrl Pts',(-9.70137854017372,-162.504517970998,
1.74701493417668E-11));
#37768=CARTESIAN_POINT('Ctrl Pts',(-7.27603390512272,-162.329517970998,
4.20082013377292));
#37769=CARTESIAN_POINT('Ctrl Pts',(-4.85068927007173,-162.154517970998,
8.40164026752836));
#37770=CARTESIAN_POINT('Ctrl Pts',(1.5129078685785E-11,-161.979517970998,
8.40164026751963));
#37771=CARTESIAN_POINT('Ctrl Pts',(4.85068927010198,-161.804517970998,8.4016402675109));
#37772=CARTESIAN_POINT('Ctrl Pts',(7.27603390513785,-161.629517970998,4.20082013374672));
#37773=CARTESIAN_POINT('Ctrl Pts',(9.70137854017372,-161.454517970998,-1.74689612655491E-11));
#37774=CARTESIAN_POINT('Ctrl Pts',(7.27603390512273,-161.279517970998,-4.20082013377291));
#37775=CARTESIAN_POINT('Ctrl Pts',(4.85068927007173,-161.104517970998,-8.40164026752836));
#37776=CARTESIAN_POINT('Ctrl Pts',(-1.51301075899711E-11,-160.929517970998,
-8.40164026751963));
#37777=CARTESIAN_POINT('Ctrl Pts',(-4.85068927010199,-160.754517970998,
-8.4016402675109));
#37778=CARTESIAN_POINT('Ctrl Pts',(-7.27603390513785,-160.579517970998,
-4.20082013374671));
#37779=CARTESIAN_POINT('Ctrl Pts',(-9.70137854017372,-160.404517970998,
1.74701493417668E-11));
#37780=CARTESIAN_POINT('Ctrl Pts',(-7.27603390512272,-160.229517970998,
4.20082013377292));
#37781=CARTESIAN_POINT('Ctrl Pts',(-4.85068927007173,-160.054517970998,
8.40164026752836));
#37782=CARTESIAN_POINT('Ctrl Pts',(1.5129078685785E-11,-159.879517970998,
8.40164026751963));
#37783=CARTESIAN_POINT('Ctrl Pts',(4.85068927010198,-159.704517970998,8.4016402675109));
#37784=CARTESIAN_POINT('Ctrl Pts',(7.27603390513785,-159.529517970998,4.20082013374672));
#37785=CARTESIAN_POINT('Ctrl Pts',(9.70137854017372,-159.354517970998,-1.74689612655491E-11));
#37786=CARTESIAN_POINT('Ctrl Pts',(7.27603390512273,-159.179517970998,-4.20082013377291));
#37787=CARTESIAN_POINT('Ctrl Pts',(4.85068927007173,-159.004517970998,-8.40164026752836));
#37788=CARTESIAN_POINT('Ctrl Pts',(-1.51301075899711E-11,-158.829517970998,
-8.40164026751963));
#37789=CARTESIAN_POINT('Ctrl Pts',(-4.85068927010199,-158.654517970998,
-8.4016402675109));
#37790=CARTESIAN_POINT('Ctrl Pts',(-7.27603390513785,-158.479517970998,
-4.20082013374671));
#37791=CARTESIAN_POINT('Ctrl Pts',(-9.70137854017372,-158.304517970998,
1.74701493417668E-11));
#37792=CARTESIAN_POINT('Ctrl Pts',(-7.27603390512272,-158.129517970998,
4.20082013377292));
#37793=CARTESIAN_POINT('Ctrl Pts',(-4.85068927007173,-157.954517970998,
8.40164026752836));
#37794=CARTESIAN_POINT('Ctrl Pts',(1.5129078685785E-11,-157.779517970998,
8.40164026751963));
#37795=CARTESIAN_POINT('Ctrl Pts',(4.85068927010198,-157.604517970998,8.4016402675109));
#37796=CARTESIAN_POINT('Ctrl Pts',(7.27603390513785,-157.429517970998,4.20082013374672));
#37797=CARTESIAN_POINT('Ctrl Pts',(9.70137854017372,-157.254517970998,-1.74689612655491E-11));
#37798=CARTESIAN_POINT('Ctrl Pts',(7.27603390512273,-157.079517970998,-4.20082013377291));
#37799=CARTESIAN_POINT('Ctrl Pts',(4.85068927007173,-156.904517970998,-8.40164026752836));
#37800=CARTESIAN_POINT('Ctrl Pts',(-1.51301075899711E-11,-156.729517970998,
-8.40164026751963));
#37801=CARTESIAN_POINT('Ctrl Pts',(-4.85068927010199,-156.554517970998,
-8.4016402675109));
#37802=CARTESIAN_POINT('Ctrl Pts',(-7.27603390513785,-156.379517970998,
-4.20082013374671));
#37803=CARTESIAN_POINT('Ctrl Pts',(-9.70137854017372,-156.204517970998,
1.74701493417668E-11));
#37804=CARTESIAN_POINT('Ctrl Pts',(-7.27603390512272,-156.029517970998,
4.20082013377292));
#37805=CARTESIAN_POINT('Ctrl Pts',(-4.85068927007173,-155.854517970998,
8.40164026752836));
#37806=CARTESIAN_POINT('Ctrl Pts',(1.5129078685785E-11,-155.679517970998,
8.40164026751963));
#37807=CARTESIAN_POINT('Ctrl Pts',(4.85068927010198,-155.504517970998,8.4016402675109));
#37808=CARTESIAN_POINT('Ctrl Pts',(7.27603390513785,-155.329517970998,4.20082013374672));
#37809=CARTESIAN_POINT('Ctrl Pts',(9.70137854017372,-155.154517970998,-1.74689612655491E-11));
#37810=CARTESIAN_POINT('Ctrl Pts',(7.27603390512273,-154.979517970998,-4.20082013377291));
#37811=CARTESIAN_POINT('Ctrl Pts',(4.85068927007173,-154.804517970998,-8.40164026752836));
#37812=CARTESIAN_POINT('Ctrl Pts',(-1.51301075899711E-11,-154.629517970998,
-8.40164026751963));
#37813=CARTESIAN_POINT('Ctrl Pts',(-4.85068927010199,-154.454517970998,
-8.4016402675109));
#37814=CARTESIAN_POINT('Ctrl Pts',(-7.27603390513785,-154.279517970998,
-4.20082013374671));
#37815=CARTESIAN_POINT('Ctrl Pts',(-9.70137854017372,-154.104517970998,
1.74701493417668E-11));
#37816=CARTESIAN_POINT('Ctrl Pts',(-7.27603390512272,-153.929517970998,
4.20082013377292));
#37817=CARTESIAN_POINT('Ctrl Pts',(-4.85068927007173,-153.754517970998,
8.40164026752836));
#37818=CARTESIAN_POINT('Ctrl Pts',(1.5129078685785E-11,-153.579517970998,
8.40164026751963));
#37819=CARTESIAN_POINT('Ctrl Pts',(4.85068927010198,-153.404517970998,8.4016402675109));
#37820=CARTESIAN_POINT('Ctrl Pts',(7.27603390513785,-153.229517970998,4.20082013374672));
#37821=CARTESIAN_POINT('Ctrl Pts',(9.70137854017372,-153.054517970998,-1.74689612655491E-11));
#37822=CARTESIAN_POINT('Ctrl Pts',(7.27603390512273,-152.879517970998,-4.20082013377291));
#37823=CARTESIAN_POINT('Ctrl Pts',(4.85068927007173,-152.704517970998,-8.40164026752836));
#37824=CARTESIAN_POINT('Ctrl Pts',(-1.51301075899711E-11,-152.529517970998,
-8.40164026751963));
#37825=CARTESIAN_POINT('Ctrl Pts',(-4.85068927010199,-152.354517970998,
-8.4016402675109));
#37826=CARTESIAN_POINT('Ctrl Pts',(-7.27603390513785,-152.179517970998,
-4.20082013374671));
#37827=CARTESIAN_POINT('Ctrl Pts',(-9.70137854017372,-152.004517970998,
1.74701493417668E-11));
#37828=CARTESIAN_POINT('Ctrl Pts',(-7.27603390512272,-151.829517970998,
4.20082013377292));
#37829=CARTESIAN_POINT('Ctrl Pts',(-4.85068927007173,-151.654517970998,
8.40164026752836));
#37830=CARTESIAN_POINT('Ctrl Pts',(1.5129078685785E-11,-151.479517970998,
8.40164026751963));
#37831=CARTESIAN_POINT('Ctrl Pts',(4.85068927010198,-151.304517970998,8.4016402675109));
#37832=CARTESIAN_POINT('Ctrl Pts',(7.27603390513785,-151.129517970998,4.20082013374672));
#37833=CARTESIAN_POINT('Ctrl Pts',(9.70137854017372,-150.954517970998,-1.74689612655491E-11));
#37834=CARTESIAN_POINT('Ctrl Pts',(7.27603390512273,-150.779517970998,-4.20082013377291));
#37835=CARTESIAN_POINT('Ctrl Pts',(4.85068927007173,-150.604517970998,-8.40164026752836));
#37836=CARTESIAN_POINT('Ctrl Pts',(-1.51301075899711E-11,-150.429517970998,
-8.40164026751963));
#37837=CARTESIAN_POINT('Ctrl Pts',(-4.85068927010199,-150.254517970998,
-8.4016402675109));
#37838=CARTESIAN_POINT('Ctrl Pts',(-7.27603390513785,-150.079517970998,
-4.20082013374671));
#37839=CARTESIAN_POINT('Ctrl Pts',(-9.70137854017372,-149.904517970998,
1.74701493417668E-11));
#37840=CARTESIAN_POINT('Ctrl Pts',(-7.27603390512272,-149.729517970998,
4.20082013377292));
#37841=CARTESIAN_POINT('Ctrl Pts',(-4.85068927007173,-149.554517970998,
8.40164026752836));
#37842=CARTESIAN_POINT('Ctrl Pts',(1.5129078685785E-11,-149.379517970998,
8.40164026751963));
#37843=CARTESIAN_POINT('Ctrl Pts',(4.85068927010198,-149.204517970998,8.4016402675109));
#37844=CARTESIAN_POINT('Ctrl Pts',(7.27603390513785,-149.029517970998,4.20082013374672));
#37845=CARTESIAN_POINT('Ctrl Pts',(9.70137854017372,-148.854517970998,-1.74689612655491E-11));
#37846=CARTESIAN_POINT('Ctrl Pts',(7.27603390512273,-148.679517970998,-4.20082013377291));
#37847=CARTESIAN_POINT('Ctrl Pts',(4.85068927007173,-148.504517970998,-8.40164026752836));
#37848=CARTESIAN_POINT('Ctrl Pts',(-1.51301075899711E-11,-148.329517970998,
-8.40164026751963));
#37849=CARTESIAN_POINT('Ctrl Pts',(-4.85068927010199,-148.154517970998,
-8.4016402675109));
#37850=CARTESIAN_POINT('Ctrl Pts',(-7.27603390513785,-147.979517970998,
-4.20082013374671));
#37851=CARTESIAN_POINT('Ctrl Pts',(-9.70137854017372,-147.804517970998,
1.74701493417668E-11));
#37852=CARTESIAN_POINT('Ctrl Pts',(-7.27603390512272,-147.629517970998,
4.20082013377292));
#37853=CARTESIAN_POINT('Ctrl Pts',(-4.85068927007173,-147.454517970998,
8.40164026752836));
#37854=CARTESIAN_POINT('Ctrl Pts',(1.5129078685785E-11,-147.279517970998,
8.40164026751963));
#37855=CARTESIAN_POINT('Ctrl Pts',(4.85068927010198,-147.104517970998,8.4016402675109));
#37856=CARTESIAN_POINT('Ctrl Pts',(7.27603390513785,-146.929517970998,4.20082013374672));
#37857=CARTESIAN_POINT('Ctrl Pts',(9.70137854017372,-146.754517970998,-1.74689612655491E-11));
#37858=CARTESIAN_POINT('Ctrl Pts',(7.27603390512273,-146.579517970998,-4.20082013377291));
#37859=CARTESIAN_POINT('Ctrl Pts',(4.85068927007173,-146.404517970998,-8.40164026752836));
#37860=CARTESIAN_POINT('Ctrl Pts',(-1.51301075899711E-11,-146.229517970998,
-8.40164026751963));
#37861=CARTESIAN_POINT('Ctrl Pts',(-4.85068927010199,-146.054517970998,
-8.4016402675109));
#37862=CARTESIAN_POINT('Ctrl Pts',(-7.27603390513785,-145.879517970998,
-4.20082013374671));
#37863=CARTESIAN_POINT('Ctrl Pts',(-9.70137854017372,-145.704517970998,
1.74701493417668E-11));
#37864=CARTESIAN_POINT('Ctrl Pts',(-7.27603390512272,-145.529517970998,
4.20082013377292));
#37865=CARTESIAN_POINT('Ctrl Pts',(-4.85068927007173,-145.354517970998,
8.40164026752836));
#37866=CARTESIAN_POINT('Ctrl Pts',(1.5129078685785E-11,-145.179517970998,
8.40164026751963));
#37867=CARTESIAN_POINT('Ctrl Pts',(4.85068927010198,-145.004517970998,8.4016402675109));
#37868=CARTESIAN_POINT('Ctrl Pts',(7.27603390513785,-144.829517970998,4.20082013374672));
#37869=CARTESIAN_POINT('Ctrl Pts',(9.70137854017372,-144.654517970998,-1.74689612655491E-11));
#37870=CARTESIAN_POINT('Ctrl Pts',(7.27603390512273,-144.479517970998,-4.20082013377291));
#37871=CARTESIAN_POINT('Ctrl Pts',(4.85068927007173,-144.304517970998,-8.40164026752836));
#37872=CARTESIAN_POINT('Ctrl Pts',(-1.51301075899711E-11,-144.129517970998,
-8.40164026751963));
#37873=CARTESIAN_POINT('Ctrl Pts',(-4.85068927010199,-143.954517970998,
-8.4016402675109));
#37874=CARTESIAN_POINT('Ctrl Pts',(-7.27603390513785,-143.779517970998,
-4.20082013374671));
#37875=CARTESIAN_POINT('Ctrl Pts',(-9.70137854017372,-143.604517970998,
1.74701493417668E-11));
#37876=CARTESIAN_POINT('Ctrl Pts',(-7.27603390512272,-143.429517970998,
4.20082013377292));
#37877=CARTESIAN_POINT('Ctrl Pts',(-4.85068927007173,-143.254517970998,
8.40164026752836));
#37878=CARTESIAN_POINT('Ctrl Pts',(1.5129078685785E-11,-143.079517970998,
8.40164026751963));
#37879=CARTESIAN_POINT('Ctrl Pts',(4.85068927010198,-142.904517970998,8.4016402675109));
#37880=CARTESIAN_POINT('Ctrl Pts',(7.27603390513785,-142.729517970998,4.20082013374672));
#37881=CARTESIAN_POINT('Ctrl Pts',(9.70137854017372,-142.554517970998,-1.74689612655491E-11));
#37882=CARTESIAN_POINT('Ctrl Pts',(7.27603390512273,-142.379517970998,-4.20082013377291));
#37883=CARTESIAN_POINT('Ctrl Pts',(4.85068927007173,-142.204517970998,-8.40164026752836));
#37884=CARTESIAN_POINT('Ctrl Pts',(-1.51301075899711E-11,-142.029517970998,
-8.40164026751963));
#37885=CARTESIAN_POINT('Ctrl Pts',(-4.85068927010199,-141.854517970998,
-8.4016402675109));
#37886=CARTESIAN_POINT('Ctrl Pts',(-7.27603390513785,-141.679517970998,
-4.20082013374671));
#37887=CARTESIAN_POINT('Ctrl Pts',(-9.70137854017372,-141.504517970998,
1.74701493417668E-11));
#37888=CARTESIAN_POINT('Ctrl Pts',(-7.27603390512272,-141.329517970998,
4.20082013377292));
#37889=CARTESIAN_POINT('Ctrl Pts',(-4.85068927007173,-141.154517970998,
8.40164026752836));
#37890=CARTESIAN_POINT('Ctrl Pts',(1.5129078685785E-11,-140.979517970998,
8.40164026751963));
#37891=CARTESIAN_POINT('Ctrl Pts',(4.85068927010198,-140.804517970998,8.4016402675109));
#37892=CARTESIAN_POINT('Ctrl Pts',(7.27603390513785,-140.629517970998,4.20082013374672));
#37893=CARTESIAN_POINT('Ctrl Pts',(9.70137854017372,-140.454517970998,-1.74689612655491E-11));
#37894=CARTESIAN_POINT('Ctrl Pts',(7.27603390512273,-140.279517970998,-4.20082013377291));
#37895=CARTESIAN_POINT('Ctrl Pts',(4.85068927007173,-140.104517970998,-8.40164026752836));
#37896=CARTESIAN_POINT('Ctrl Pts',(-1.51301075899711E-11,-139.929517970998,
-8.40164026751963));
#37897=CARTESIAN_POINT('Ctrl Pts',(-4.85068927010199,-139.754517970998,
-8.4016402675109));
#37898=CARTESIAN_POINT('Ctrl Pts',(-7.27603390513785,-139.579517970998,
-4.20082013374671));
#37899=CARTESIAN_POINT('Ctrl Pts',(-9.70137854017372,-139.404517970998,
1.74701493417668E-11));
#37900=CARTESIAN_POINT('Ctrl Pts',(-7.27603390512272,-139.229517970998,
4.20082013377292));
#37901=CARTESIAN_POINT('Ctrl Pts',(-4.85068927007173,-139.054517970998,
8.40164026752836));
#37902=CARTESIAN_POINT('Ctrl Pts',(1.5129078685785E-11,-138.879517970998,
8.40164026751963));
#37903=CARTESIAN_POINT('Ctrl Pts',(4.85068927010198,-138.704517970998,8.4016402675109));
#37904=CARTESIAN_POINT('Ctrl Pts',(7.27603390513785,-138.529517970998,4.20082013374672));
#37905=CARTESIAN_POINT('Ctrl Pts',(9.70137854017372,-138.354517970998,-1.74689612655491E-11));
#37906=CARTESIAN_POINT('Ctrl Pts',(7.27603390512273,-138.179517970998,-4.20082013377291));
#37907=CARTESIAN_POINT('Ctrl Pts',(4.85068927007173,-138.004517970998,-8.40164026752836));
#37908=CARTESIAN_POINT('Ctrl Pts',(-1.51301075899711E-11,-137.829517970998,
-8.40164026751963));
#37909=CARTESIAN_POINT('Ctrl Pts',(-4.85068927010199,-137.654517970998,
-8.4016402675109));
#37910=CARTESIAN_POINT('Ctrl Pts',(-7.27603390513785,-137.479517970998,
-4.20082013374671));
#37911=CARTESIAN_POINT('Ctrl Pts',(-9.70137854017372,-137.304517970998,
1.74701493417668E-11));
#37912=CARTESIAN_POINT('Ctrl Pts',(-7.27603390512272,-137.129517970998,
4.20082013377292));
#37913=CARTESIAN_POINT('Ctrl Pts',(-4.85068927007173,-136.954517970998,
8.40164026752836));
#37914=CARTESIAN_POINT('Ctrl Pts',(1.5129078685785E-11,-136.779517970998,
8.40164026751963));
#37915=CARTESIAN_POINT('Ctrl Pts',(4.85068927010198,-136.604517970998,8.4016402675109));
#37916=CARTESIAN_POINT('Ctrl Pts',(7.27603390513785,-136.429517970998,4.20082013374672));
#37917=CARTESIAN_POINT('Ctrl Pts',(9.70137854017372,-136.254517970999,-1.74689612655491E-11));
#37918=CARTESIAN_POINT('Ctrl Pts',(7.27603390512273,-136.079517970998,-4.20082013377291));
#37919=CARTESIAN_POINT('Ctrl Pts',(4.85068927007173,-135.904517970998,-8.40164026752836));
#37920=CARTESIAN_POINT('Ctrl Pts',(-1.51301075899711E-11,-135.729517970998,
-8.40164026751963));
#37921=CARTESIAN_POINT('Ctrl Pts',(-4.85068927010199,-135.554517970998,
-8.4016402675109));
#37922=CARTESIAN_POINT('Ctrl Pts',(-7.27603390513785,-135.379517970998,
-4.20082013374671));
#37923=CARTESIAN_POINT('Ctrl Pts',(-9.70137854017372,-135.204517970998,
1.74701493417668E-11));
#37924=CARTESIAN_POINT('Ctrl Pts',(-7.27603390512272,-135.029517970998,
4.20082013377292));
#37925=CARTESIAN_POINT('Ctrl Pts',(-4.85068927007173,-134.854517970998,
8.40164026752836));
#37926=CARTESIAN_POINT('Ctrl Pts',(1.5129078685785E-11,-134.679517970998,
8.40164026751963));
#37927=CARTESIAN_POINT('Ctrl Pts',(4.85068927010198,-134.504517970998,8.4016402675109));
#37928=CARTESIAN_POINT('Ctrl Pts',(7.27603390513785,-134.329517970998,4.20082013374672));
#37929=CARTESIAN_POINT('Ctrl Pts',(9.70137854017372,-134.154517970998,-1.74689612655491E-11));
#37930=CARTESIAN_POINT('Ctrl Pts',(7.27603390512273,-133.979517970998,-4.20082013377291));
#37931=CARTESIAN_POINT('Ctrl Pts',(4.85068927007173,-133.804517970998,-8.40164026752836));
#37932=CARTESIAN_POINT('Ctrl Pts',(-1.51301075899711E-11,-133.629517970998,
-8.40164026751963));
#37933=CARTESIAN_POINT('Ctrl Pts',(-4.85068927010199,-133.454517970998,
-8.4016402675109));
#37934=CARTESIAN_POINT('Ctrl Pts',(-7.27603390513785,-133.279517970998,
-4.20082013374671));
#37935=CARTESIAN_POINT('Ctrl Pts',(-9.70137854017372,-133.104517970998,
1.74701493417668E-11));
#37936=CARTESIAN_POINT('Ctrl Pts',(-7.27603390512272,-132.929517970998,
4.20082013377292));
#37937=CARTESIAN_POINT('Ctrl Pts',(-4.85068927007173,-132.754517970998,
8.40164026752836));
#37938=CARTESIAN_POINT('Ctrl Pts',(1.5129078685785E-11,-132.579517970998,
8.40164026751963));
#37939=CARTESIAN_POINT('Ctrl Pts',(4.85068927010198,-132.404517970998,8.4016402675109));
#37940=CARTESIAN_POINT('Ctrl Pts',(7.27603390513785,-132.229517970998,4.20082013374672));
#37941=CARTESIAN_POINT('Ctrl Pts',(9.70137854017372,-132.054517970998,-1.74689612655491E-11));
#37942=CARTESIAN_POINT('Ctrl Pts',(7.27603390512273,-131.879517970998,-4.20082013377291));
#37943=CARTESIAN_POINT('Ctrl Pts',(4.85068927007173,-131.704517970998,-8.40164026752836));
#37944=CARTESIAN_POINT('Ctrl Pts',(-1.51301075899711E-11,-131.529517970998,
-8.40164026751963));
#37945=CARTESIAN_POINT('Ctrl Pts',(-4.85068927010199,-131.354517970998,
-8.4016402675109));
#37946=CARTESIAN_POINT('Ctrl Pts',(-7.27603390513785,-131.179517970998,
-4.20082013374671));
#37947=CARTESIAN_POINT('Ctrl Pts',(-9.70137854017372,-131.004517970998,
1.74701493417668E-11));
#37948=CARTESIAN_POINT('Ctrl Pts',(-7.27603390512272,-130.829517970998,
4.20082013377292));
#37949=CARTESIAN_POINT('Ctrl Pts',(-4.85068927007173,-130.654517970998,
8.40164026752836));
#37950=CARTESIAN_POINT('Ctrl Pts',(1.5129078685785E-11,-130.479517970998,
8.40164026751963));
#37951=CARTESIAN_POINT('Ctrl Pts',(4.85068927010198,-130.304517970998,8.4016402675109));
#37952=CARTESIAN_POINT('Ctrl Pts',(7.27603390513785,-130.129517970998,4.20082013374672));
#37953=CARTESIAN_POINT('Ctrl Pts',(9.70137854017372,-129.954517970998,-1.74689612655491E-11));
#37954=CARTESIAN_POINT('Ctrl Pts',(7.27603390512273,-129.779517970998,-4.20082013377291));
#37955=CARTESIAN_POINT('Ctrl Pts',(4.85068927007173,-129.604517970998,-8.40164026752836));
#37956=CARTESIAN_POINT('Ctrl Pts',(-1.51301075899711E-11,-129.429517970998,
-8.40164026751963));
#37957=CARTESIAN_POINT('Ctrl Pts',(-4.85068927010199,-129.254517970998,
-8.4016402675109));
#37958=CARTESIAN_POINT('Ctrl Pts',(-7.27603390513785,-129.079517970998,
-4.20082013374671));
#37959=CARTESIAN_POINT('Ctrl Pts',(-9.70137854017372,-128.904517970998,
1.74701493417668E-11));
#37960=CARTESIAN_POINT('Ctrl Pts',(-7.27603390512272,-128.729517970998,
4.20082013377292));
#37961=CARTESIAN_POINT('Ctrl Pts',(-4.85068927007173,-128.554517970998,
8.40164026752836));
#37962=CARTESIAN_POINT('Ctrl Pts',(1.5129078685785E-11,-128.379517970998,
8.40164026751963));
#37963=CARTESIAN_POINT('Ctrl Pts',(4.85068927010198,-128.204517970998,8.4016402675109));
#37964=CARTESIAN_POINT('Ctrl Pts',(7.27603390513785,-128.029517970998,4.20082013374672));
#37965=CARTESIAN_POINT('Ctrl Pts',(9.70137854017372,-127.854517970998,-1.74689612655491E-11));
#37966=CARTESIAN_POINT('Ctrl Pts',(7.27603390512273,-127.679517970998,-4.20082013377291));
#37967=CARTESIAN_POINT('Ctrl Pts',(4.85068927007173,-127.504517970998,-8.40164026752836));
#37968=CARTESIAN_POINT('Ctrl Pts',(-1.51301075899711E-11,-127.329517970998,
-8.40164026751963));
#37969=CARTESIAN_POINT('Ctrl Pts',(-4.85068927010199,-127.154517970998,
-8.4016402675109));
#37970=CARTESIAN_POINT('Ctrl Pts',(-7.27603390513785,-126.979517970998,
-4.20082013374671));
#37971=CARTESIAN_POINT('Ctrl Pts',(-9.70137854017372,-126.804517970998,
1.74701493417668E-11));
#37972=CARTESIAN_POINT('Ctrl Pts',(-7.27603390512272,-126.629517970998,
4.20082013377292));
#37973=CARTESIAN_POINT('Ctrl Pts',(-4.85068927007173,-126.454517970998,
8.40164026752836));
#37974=CARTESIAN_POINT('Ctrl Pts',(1.5129078685785E-11,-126.279517970998,
8.40164026751963));
#37975=CARTESIAN_POINT('Ctrl Pts',(4.85068927010198,-126.104517970998,8.4016402675109));
#37976=CARTESIAN_POINT('Ctrl Pts',(7.27603390513785,-125.929517970998,4.20082013374672));
#37977=CARTESIAN_POINT('Ctrl Pts',(9.70137854017372,-125.754517970998,-1.74689612655491E-11));
#37978=CARTESIAN_POINT('Ctrl Pts',(7.27603390512273,-125.579517970998,-4.20082013377291));
#37979=CARTESIAN_POINT('Ctrl Pts',(4.85068927007173,-125.404517970998,-8.40164026752836));
#37980=CARTESIAN_POINT('Ctrl Pts',(-1.51301075899711E-11,-125.229517970998,
-8.40164026751963));
#37981=CARTESIAN_POINT('Ctrl Pts',(-4.85068927010199,-125.054517970998,
-8.4016402675109));
#37982=CARTESIAN_POINT('Ctrl Pts',(-7.27603390513785,-124.879517970998,
-4.20082013374671));
#37983=CARTESIAN_POINT('Ctrl Pts',(-9.70137854017372,-124.704517970998,
1.74701493417668E-11));
#37984=CARTESIAN_POINT('Ctrl Pts',(-7.27603390512272,-124.529517970998,
4.20082013377292));
#37985=CARTESIAN_POINT('Ctrl Pts',(-4.85068927007173,-124.354517970998,
8.40164026752836));
#37986=CARTESIAN_POINT('Ctrl Pts',(1.5129078685785E-11,-124.179517970998,
8.40164026751963));
#37987=CARTESIAN_POINT('Ctrl Pts',(4.85068927010198,-124.004517970998,8.4016402675109));
#37988=CARTESIAN_POINT('Ctrl Pts',(7.27603390513785,-123.829517970998,4.20082013374672));
#37989=CARTESIAN_POINT('Ctrl Pts',(9.70137854017372,-123.654517970998,-1.74689612655491E-11));
#37990=CARTESIAN_POINT('Ctrl Pts',(7.27603390512273,-123.479517970998,-4.20082013377291));
#37991=CARTESIAN_POINT('Ctrl Pts',(4.85068927007173,-123.304517970998,-8.40164026752836));
#37992=CARTESIAN_POINT('Ctrl Pts',(-1.51301075899711E-11,-123.129517970998,
-8.40164026751963));
#37993=CARTESIAN_POINT('Ctrl Pts',(-4.85068927010199,-122.954517970998,
-8.4016402675109));
#37994=CARTESIAN_POINT('Ctrl Pts',(-7.27603390513785,-122.779517970998,
-4.20082013374671));
#37995=CARTESIAN_POINT('Ctrl Pts',(-9.70137854017372,-122.604517970998,
1.74701493417668E-11));
#37996=CARTESIAN_POINT('Ctrl Pts',(-7.27603390512272,-122.429517970998,
4.20082013377292));
#37997=CARTESIAN_POINT('Ctrl Pts',(-4.85068927007173,-122.254517970998,
8.40164026752836));
#37998=CARTESIAN_POINT('Ctrl Pts',(1.5129078685785E-11,-122.079517970998,
8.40164026751963));
#37999=CARTESIAN_POINT('Ctrl Pts',(4.85068927010198,-121.904517970998,8.4016402675109));
#38000=CARTESIAN_POINT('Ctrl Pts',(7.27603390513785,-121.729517970998,4.20082013374672));
#38001=CARTESIAN_POINT('Ctrl Pts',(9.70137854017372,-121.554517970999,-1.74689612655491E-11));
#38002=CARTESIAN_POINT('Ctrl Pts',(7.27603390512273,-121.379517970998,-4.20082013377291));
#38003=CARTESIAN_POINT('Ctrl Pts',(4.85068927007173,-121.204517970998,-8.40164026752836));
#38004=CARTESIAN_POINT('Ctrl Pts',(-1.51301075899711E-11,-121.029517970998,
-8.40164026751963));
#38005=CARTESIAN_POINT('Ctrl Pts',(-4.85068927010199,-120.854517970999,
-8.4016402675109));
#38006=CARTESIAN_POINT('Ctrl Pts',(-7.27603390513785,-120.679517970999,
-4.20082013374671));
#38007=CARTESIAN_POINT('Ctrl Pts',(-9.70137854017372,-120.504517970999,
1.74701493417668E-11));
#38008=CARTESIAN_POINT('Ctrl Pts',(-7.27603390512272,-120.329517970998,
4.20082013377292));
#38009=CARTESIAN_POINT('Ctrl Pts',(-4.85068927007173,-120.154517970998,
8.40164026752836));
#38010=CARTESIAN_POINT('Ctrl Pts',(1.5129078685785E-11,-119.979517970999,
8.40164026751963));
#38011=CARTESIAN_POINT('Ctrl Pts',(4.85068927010198,-119.804517970999,8.4016402675109));
#38012=CARTESIAN_POINT('Ctrl Pts',(7.27603390513785,-119.629517970998,4.20082013374672));
#38013=CARTESIAN_POINT('Ctrl Pts',(9.70137854017372,-119.454517970998,-1.74689612655491E-11));
#38014=CARTESIAN_POINT('Ctrl Pts',(7.27603390512273,-119.279517970999,-4.20082013377291));
#38015=CARTESIAN_POINT('Ctrl Pts',(4.85068927007173,-119.104517970998,-8.40164026752836));
#38016=CARTESIAN_POINT('Ctrl Pts',(-1.51301075899711E-11,-118.929517970998,
-8.40164026751963));
#38017=CARTESIAN_POINT('Ctrl Pts',(-4.85068927010199,-118.754517970998,
-8.4016402675109));
#38018=CARTESIAN_POINT('Ctrl Pts',(-7.27603390513785,-118.579517970998,
-4.20082013374671));
#38019=CARTESIAN_POINT('Ctrl Pts',(-9.70137854017372,-118.404517970999,
1.74701493417668E-11));
#38020=CARTESIAN_POINT('Ctrl Pts',(-7.27603390512272,-118.229517970998,
4.20082013377292));
#38021=CARTESIAN_POINT('Ctrl Pts',(-4.85068927007173,-118.054517970998,
8.40164026752836));
#38022=CARTESIAN_POINT('Ctrl Pts',(1.5129078685785E-11,-117.879517970999,
8.40164026751963));
#38023=CARTESIAN_POINT('Ctrl Pts',(4.85068927010198,-117.704517970998,8.4016402675109));
#38024=CARTESIAN_POINT('Ctrl Pts',(7.27603390513785,-117.529517970998,4.20082013374672));
#38025=CARTESIAN_POINT('Ctrl Pts',(9.70137854017372,-117.354517970999,-1.74689612655491E-11));
#38026=CARTESIAN_POINT('Ctrl Pts',(7.27603390512273,-117.179517970999,-4.20082013377291));
#38027=CARTESIAN_POINT('Ctrl Pts',(4.85068927007173,-117.004517970999,-8.40164026752836));
#38028=CARTESIAN_POINT('Ctrl Pts',(-1.51301075899711E-11,-116.829517970998,
-8.40164026751963));
#38029=CARTESIAN_POINT('Ctrl Pts',(-4.85068927010199,-116.654517970998,
-8.4016402675109));
#38030=CARTESIAN_POINT('Ctrl Pts',(-7.27603390513785,-116.479517970999,
-4.20082013374671));
#38031=CARTESIAN_POINT('Ctrl Pts',(-9.70137854017372,-116.304517970999,
1.74701493417668E-11));
#38032=CARTESIAN_POINT('Ctrl Pts',(-7.27603390512272,-116.129517970999,
4.20082013377292));
#38033=CARTESIAN_POINT('Ctrl Pts',(-4.85068927007173,-115.954517970998,
8.40164026752836));
#38034=CARTESIAN_POINT('Ctrl Pts',(1.5129078685785E-11,-115.779517970998,
8.40164026751963));
#38035=CARTESIAN_POINT('Ctrl Pts',(4.85068927010198,-115.604517970999,8.4016402675109));
#38036=CARTESIAN_POINT('Ctrl Pts',(7.27603390513785,-115.429517970999,4.20082013374672));
#38037=CARTESIAN_POINT('Ctrl Pts',(9.70137854017372,-115.254517970999,-1.74689612655491E-11));
#38038=CARTESIAN_POINT('Ctrl Pts',(7.27603390512273,-115.079517970998,-4.20082013377291));
#38039=CARTESIAN_POINT('Ctrl Pts',(4.85068927007173,-114.904517970999,-8.40164026752836));
#38040=CARTESIAN_POINT('Ctrl Pts',(-1.51301075899711E-11,-114.729517970999,
-8.40164026751963));
#38041=CARTESIAN_POINT('Ctrl Pts',(-4.85068927010199,-114.554517970999,
-8.4016402675109));
#38042=CARTESIAN_POINT('Ctrl Pts',(-7.27603390513785,-114.379517970999,
-4.20082013374671));
#38043=CARTESIAN_POINT('Ctrl Pts',(-9.70137854017372,-114.204517970999,
1.74701493417668E-11));
#38044=CARTESIAN_POINT('Ctrl Pts',(-7.27603390512272,-114.029517970999,
4.20082013377292));
#38045=CARTESIAN_POINT('Ctrl Pts',(-4.85068927007173,-113.854517970999,
8.40164026752836));
#38046=CARTESIAN_POINT('Ctrl Pts',(1.5129078685785E-11,-113.679517970999,
8.40164026751963));
#38047=CARTESIAN_POINT('Ctrl Pts',(4.85068927010198,-113.504517970999,8.4016402675109));
#38048=CARTESIAN_POINT('Ctrl Pts',(7.27603390513785,-113.329517970999,4.20082013374672));
#38049=CARTESIAN_POINT('Ctrl Pts',(9.70137854017372,-113.154517970999,-1.74689612655491E-11));
#38050=CARTESIAN_POINT('Ctrl Pts',(7.27603390512273,-112.979517970999,-4.20082013377291));
#38051=CARTESIAN_POINT('Ctrl Pts',(4.85068927007173,-112.804517970999,-8.40164026752836));
#38052=CARTESIAN_POINT('Ctrl Pts',(-1.51301075899711E-11,-112.629517970999,
-8.40164026751963));
#38053=CARTESIAN_POINT('Ctrl Pts',(-4.85068927010199,-112.454517970998,
-8.4016402675109));
#38054=CARTESIAN_POINT('Ctrl Pts',(-7.27603390513785,-112.279517970998,
-4.20082013374671));
#38055=CARTESIAN_POINT('Ctrl Pts',(-9.70137854017372,-112.104517970999,
1.74701493417668E-11));
#38056=CARTESIAN_POINT('Ctrl Pts',(-7.27603390512272,-111.929517970999,
4.20082013377292));
#38057=CARTESIAN_POINT('Ctrl Pts',(-4.85068927007173,-111.754517970999,
8.40164026752836));
#38058=CARTESIAN_POINT('Ctrl Pts',(1.5129078685785E-11,-111.579517970999,
8.40164026751963));
#38059=CARTESIAN_POINT('Ctrl Pts',(4.85068927010198,-111.404517970998,8.4016402675109));
#38060=CARTESIAN_POINT('Ctrl Pts',(7.27603390513785,-111.229517970999,4.20082013374672));
#38061=CARTESIAN_POINT('Ctrl Pts',(9.70137854017372,-111.054517970999,-1.74689612655491E-11));
#38062=CARTESIAN_POINT('Ctrl Pts',(7.27603390512273,-110.879517970999,-4.20082013377291));
#38063=CARTESIAN_POINT('Ctrl Pts',(4.85068927007173,-110.704517970999,-8.40164026752836));
#38064=CARTESIAN_POINT('Ctrl Pts',(-1.51301075899711E-11,-110.529517970999,
-8.40164026751963));
#38065=CARTESIAN_POINT('Ctrl Pts',(-4.85068927010199,-110.354517970999,
-8.4016402675109));
#38066=CARTESIAN_POINT('Ctrl Pts',(-7.27603390513785,-110.179517970999,
-4.20082013374671));
#38067=CARTESIAN_POINT('Ctrl Pts',(-9.70137854017372,-110.004517970999,
1.74701493417668E-11));
#38068=CARTESIAN_POINT('Ctrl Pts',(-7.27603390512272,-109.829517970999,
4.20082013377292));
#38069=CARTESIAN_POINT('Ctrl Pts',(-4.85068927007173,-109.654517970999,
8.40164026752836));
#38070=CARTESIAN_POINT('Ctrl Pts',(1.5129078685785E-11,-109.479517970999,
8.40164026751963));
#38071=CARTESIAN_POINT('Ctrl Pts',(4.85068927010198,-109.304517970999,8.4016402675109));
#38072=CARTESIAN_POINT('Ctrl Pts',(7.27603390513785,-109.129517970999,4.20082013374672));
#38073=CARTESIAN_POINT('Ctrl Pts',(9.70137854017372,-108.954517970999,-1.74689612655491E-11));
#38074=CARTESIAN_POINT('Ctrl Pts',(7.27603390512273,-108.779517970999,-4.20082013377291));
#38075=CARTESIAN_POINT('Ctrl Pts',(4.85068927007173,-108.604517970999,-8.40164026752836));
#38076=CARTESIAN_POINT('Ctrl Pts',(-1.51301075899711E-11,-108.429517970999,
-8.40164026751963));
#38077=CARTESIAN_POINT('Ctrl Pts',(-4.85068927010199,-108.254517970999,
-8.4016402675109));
#38078=CARTESIAN_POINT('Ctrl Pts',(-7.27603390513785,-108.079517970999,
-4.20082013374671));
#38079=CARTESIAN_POINT('Ctrl Pts',(-9.70137854017372,-107.904517970999,
1.74701493417668E-11));
#38080=CARTESIAN_POINT('Ctrl Pts',(-7.27603390512272,-107.729517970999,
4.20082013377292));
#38081=CARTESIAN_POINT('Ctrl Pts',(-4.85068927007173,-107.554517970999,
8.40164026752836));
#38082=CARTESIAN_POINT('Ctrl Pts',(1.5129078685785E-11,-107.379517970999,
8.40164026751963));
#38083=CARTESIAN_POINT('Ctrl Pts',(4.85068927010198,-107.204517970999,8.4016402675109));
#38084=CARTESIAN_POINT('Ctrl Pts',(7.27603390513785,-107.029517970999,4.20082013374672));
#38085=CARTESIAN_POINT('Ctrl Pts',(9.70137854017372,-106.854517970999,-1.74689612655491E-11));
#38086=CARTESIAN_POINT('Ctrl Pts',(7.27603390512273,-106.679517970999,-4.20082013377291));
#38087=CARTESIAN_POINT('Ctrl Pts',(4.85068927007173,-106.504517970998,-8.40164026752836));
#38088=CARTESIAN_POINT('Ctrl Pts',(-1.51301075899711E-11,-106.329517970999,
-8.40164026751963));
#38089=CARTESIAN_POINT('Ctrl Pts',(-4.85068927010199,-106.154517970999,
-8.4016402675109));
#38090=CARTESIAN_POINT('Ctrl Pts',(-7.27603390513785,-105.979517970999,
-4.20082013374671));
#38091=CARTESIAN_POINT('Ctrl Pts',(-9.70137854017372,-105.804517970999,
1.74701493417668E-11));
#38092=CARTESIAN_POINT('Ctrl Pts',(-7.27603390512272,-105.629517970999,
4.20082013377292));
#38093=CARTESIAN_POINT('Ctrl Pts',(-4.85068927007173,-105.454517970999,
8.40164026752836));
#38094=CARTESIAN_POINT('Ctrl Pts',(1.5129078685785E-11,-105.279517970999,
8.40164026751963));
#38095=CARTESIAN_POINT('Ctrl Pts',(4.85068927010198,-105.104517970999,8.4016402675109));
#38096=CARTESIAN_POINT('Ctrl Pts',(7.27603390513785,-104.929517970999,4.20082013374672));
#38097=CARTESIAN_POINT('Ctrl Pts',(9.70137854017372,-104.754517970999,-1.74689612655491E-11));
#38098=CARTESIAN_POINT('Ctrl Pts',(7.27603390512273,-104.579517970999,-4.20082013377291));
#38099=CARTESIAN_POINT('Ctrl Pts',(4.85068927007173,-104.404517970999,-8.40164026752836));
#38100=CARTESIAN_POINT('Ctrl Pts',(-1.51301075899711E-11,-104.229517970999,
-8.40164026751963));
#38101=CARTESIAN_POINT('Ctrl Pts',(-4.85068927010199,-104.054517970999,
-8.4016402675109));
#38102=CARTESIAN_POINT('Ctrl Pts',(-7.27603390513785,-103.879517970999,
-4.20082013374671));
#38103=CARTESIAN_POINT('Ctrl Pts',(-9.70137854017372,-103.704517970999,
1.74701493417668E-11));
#38104=CARTESIAN_POINT('Ctrl Pts',(-7.27603390512272,-103.529517970999,
4.20082013377292));
#38105=CARTESIAN_POINT('Ctrl Pts',(-4.85068927007173,-103.354517970999,
8.40164026752836));
#38106=CARTESIAN_POINT('Ctrl Pts',(1.5129078685785E-11,-103.179517970999,
8.40164026751963));
#38107=CARTESIAN_POINT('Ctrl Pts',(4.85068927010198,-103.004517970999,8.4016402675109));
#38108=CARTESIAN_POINT('Ctrl Pts',(7.27603390513785,-102.829517970999,4.20082013374672));
#38109=CARTESIAN_POINT('Ctrl Pts',(9.70137854017372,-102.654517970999,-1.74689612655491E-11));
#38110=CARTESIAN_POINT('Ctrl Pts',(7.27603390512273,-102.479517970999,-4.20082013377291));
#38111=CARTESIAN_POINT('Ctrl Pts',(4.85068927007173,-102.304517970999,-8.40164026752836));
#38112=CARTESIAN_POINT('Ctrl Pts',(-1.51301075899711E-11,-102.129517970999,
-8.40164026751963));
#38113=CARTESIAN_POINT('Ctrl Pts',(-4.85068927010199,-101.954517970999,
-8.4016402675109));
#38114=CARTESIAN_POINT('Ctrl Pts',(-7.27603390513785,-101.779517970999,
-4.20082013374671));
#38115=CARTESIAN_POINT('Ctrl Pts',(-9.70137854017372,-101.604517970999,
1.74701493417668E-11));
#38116=CARTESIAN_POINT('Ctrl Pts',(-7.27603390512272,-101.429517970999,
4.20082013377292));
#38117=CARTESIAN_POINT('Ctrl Pts',(-4.85068927007173,-101.254517970999,
8.40164026752836));
#38118=CARTESIAN_POINT('Ctrl Pts',(1.5129078685785E-11,-101.079517970999,
8.40164026751963));
#38119=CARTESIAN_POINT('Ctrl Pts',(4.85068927010198,-100.904517970999,8.4016402675109));
#38120=CARTESIAN_POINT('Ctrl Pts',(7.27603390513785,-100.729517970999,4.20082013374672));
#38121=CARTESIAN_POINT('Ctrl Pts',(9.70137854017372,-100.554517970999,-1.74689612655491E-11));
#38122=CARTESIAN_POINT('Ctrl Pts',(7.27603390512273,-100.379517970999,-4.20082013377291));
#38123=CARTESIAN_POINT('Ctrl Pts',(4.85068927007173,-100.204517970999,-8.40164026752836));
#38124=CARTESIAN_POINT('Ctrl Pts',(-1.51301075899711E-11,-100.029517970999,
-8.40164026751963));
#38125=CARTESIAN_POINT('Ctrl Pts',(-4.85068927010199,-99.8545179709986,
-8.4016402675109));
#38126=CARTESIAN_POINT('Ctrl Pts',(-7.27603390513785,-99.6795179709985,
-4.20082013374671));
#38127=CARTESIAN_POINT('Ctrl Pts',(-9.70137854017372,-99.5045179709985,
1.74701493417668E-11));
#38128=CARTESIAN_POINT('Ctrl Pts',(-7.27603390512272,-99.3295179709985,
4.20082013377292));
#38129=CARTESIAN_POINT('Ctrl Pts',(-4.85068927007173,-99.1545179709985,
8.40164026752836));
#38130=CARTESIAN_POINT('Ctrl Pts',(1.5129078685785E-11,-98.9795179709985,
8.40164026751963));
#38131=CARTESIAN_POINT('Ctrl Pts',(4.85068927010198,-98.8045179709985,8.4016402675109));
#38132=CARTESIAN_POINT('Ctrl Pts',(7.27603390513785,-98.6295179709985,4.20082013374672));
#38133=CARTESIAN_POINT('Ctrl Pts',(9.70137854017372,-98.4545179709986,-1.74689612655491E-11));
#38134=CARTESIAN_POINT('Ctrl Pts',(7.27603390512273,-98.2795179709986,-4.20082013377291));
#38135=CARTESIAN_POINT('Ctrl Pts',(4.85068927007173,-98.1045179709986,-8.40164026752836));
#38136=CARTESIAN_POINT('Ctrl Pts',(-1.51301075899711E-11,-97.9295179709985,
-8.40164026751963));
#38137=CARTESIAN_POINT('Ctrl Pts',(-4.85068927010199,-97.7545179709985,
-8.4016402675109));
#38138=CARTESIAN_POINT('Ctrl Pts',(-7.27603390513785,-97.5795179709986,
-4.20082013374671));
#38139=CARTESIAN_POINT('Ctrl Pts',(-9.70137854017372,-97.4045179709985,
1.74701493417668E-11));
#38140=CARTESIAN_POINT('Ctrl Pts',(-7.27603390512272,-97.2295179709985,
4.20082013377292));
#38141=CARTESIAN_POINT('Ctrl Pts',(-4.85068927007173,-97.0545179709985,
8.40164026752836));
#38142=CARTESIAN_POINT('Ctrl Pts',(1.5129078685785E-11,-96.8795179709986,
8.40164026751963));
#38143=CARTESIAN_POINT('Ctrl Pts',(4.85068927010198,-96.7045179709986,8.4016402675109));
#38144=CARTESIAN_POINT('Ctrl Pts',(7.27603390513785,-96.5295179709985,4.20082013374672));
#38145=CARTESIAN_POINT('Ctrl Pts',(9.70137854017372,-96.3545179709985,-1.74689612655491E-11));
#38146=CARTESIAN_POINT('Ctrl Pts',(7.27603390512273,-96.1795179709985,-4.20082013377291));
#38147=CARTESIAN_POINT('Ctrl Pts',(4.85068927007173,-96.0045179709986,-8.40164026752836));
#38148=CARTESIAN_POINT('Ctrl Pts',(-1.51301075899711E-11,-95.8295179709985,
-8.40164026751963));
#38149=CARTESIAN_POINT('Ctrl Pts',(-4.85068927010199,-95.6545179709985,
-8.4016402675109));
#38150=CARTESIAN_POINT('Ctrl Pts',(-7.27603390513785,-95.4795179709985,
-4.20082013374671));
#38151=CARTESIAN_POINT('Ctrl Pts',(-9.70137854017372,-95.3045179709986,
1.74701493417668E-11));
#38152=CARTESIAN_POINT('Ctrl Pts',(-7.27603390512272,-95.1295179709986,
4.20082013377292));
#38153=CARTESIAN_POINT('Ctrl Pts',(-4.85068927007173,-94.9545179709986,
8.40164026752836));
#38154=CARTESIAN_POINT('Ctrl Pts',(1.5129078685785E-11,-94.7795179709985,
8.40164026751963));
#38155=CARTESIAN_POINT('Ctrl Pts',(4.85068927010198,-94.6045179709986,8.4016402675109));
#38156=CARTESIAN_POINT('Ctrl Pts',(7.27603390513785,-94.4295179709985,4.20082013374672));
#38157=CARTESIAN_POINT('Ctrl Pts',(9.70137854017372,-94.2545179709985,-1.74689612655491E-11));
#38158=CARTESIAN_POINT('Ctrl Pts',(7.27603390512273,-94.0795179709986,-4.20082013377291));
#38159=CARTESIAN_POINT('Ctrl Pts',(4.85068927007173,-93.9045179709986,-8.40164026752836));
#38160=CARTESIAN_POINT('Ctrl Pts',(-1.51301075899711E-11,-93.7295179709986,
-8.40164026751963));
#38161=CARTESIAN_POINT('Ctrl Pts',(-4.85068927010199,-93.5545179709985,
-8.4016402675109));
#38162=CARTESIAN_POINT('Ctrl Pts',(-7.27603390513785,-93.3795179709985,
-4.20082013374671));
#38163=CARTESIAN_POINT('Ctrl Pts',(-9.70137854017372,-93.2045179709986,
1.74701493417668E-11));
#38164=CARTESIAN_POINT('Ctrl Pts',(-7.27603390512272,-93.0295179709986,
4.20082013377292));
#38165=CARTESIAN_POINT('Ctrl Pts',(-4.85068927007173,-92.8545179709985,
8.40164026752836));
#38166=CARTESIAN_POINT('Ctrl Pts',(1.5129078685785E-11,-92.6795179709985,
8.40164026751963));
#38167=CARTESIAN_POINT('Ctrl Pts',(4.85068927010198,-92.5045179709985,8.4016402675109));
#38168=CARTESIAN_POINT('Ctrl Pts',(7.27603390513785,-92.3295179709986,4.20082013374672));
#38169=CARTESIAN_POINT('Ctrl Pts',(9.70137854017372,-92.1545179709986,-1.74689612655491E-11));
#38170=CARTESIAN_POINT('Ctrl Pts',(7.27603390512273,-91.9795179709986,-4.20082013377291));
#38171=CARTESIAN_POINT('Ctrl Pts',(4.85068927007173,-91.8045179709985,-8.40164026752836));
#38172=CARTESIAN_POINT('Ctrl Pts',(-1.51301075899711E-11,-91.6295179709986,
-8.40164026751963));
#38173=CARTESIAN_POINT('Ctrl Pts',(-4.85068927010199,-91.4545179709986,
-8.4016402675109));
#38174=CARTESIAN_POINT('Ctrl Pts',(-7.27603390513785,-91.2795179709986,
-4.20082013374671));
#38175=CARTESIAN_POINT('Ctrl Pts',(-9.70137854017372,-91.1045179709985,
1.74701493417668E-11));
#38176=CARTESIAN_POINT('Ctrl Pts',(-7.27603390512272,-90.9295179709986,
4.20082013377292));
#38177=CARTESIAN_POINT('Ctrl Pts',(-4.85068927007173,-90.7545179709986,
8.40164026752836));
#38178=CARTESIAN_POINT('Ctrl Pts',(1.5129078685785E-11,-90.5795179709986,
8.40164026751963));
#38179=CARTESIAN_POINT('Ctrl Pts',(4.85068927010198,-90.4045179709985,8.4016402675109));
#38180=CARTESIAN_POINT('Ctrl Pts',(7.27603390513785,-90.2295179709986,4.20082013374672));
#38181=CARTESIAN_POINT('Ctrl Pts',(9.70137854017372,-90.0545179709986,-1.74689612655491E-11));
#38182=CARTESIAN_POINT('Ctrl Pts',(7.27603390512273,-89.8795179709985,-4.20082013377291));
#38183=CARTESIAN_POINT('Ctrl Pts',(4.85068927007173,-89.7045179709986,-8.40164026752836));
#38184=CARTESIAN_POINT('Ctrl Pts',(-1.51301075899711E-11,-89.5295179709986,
-8.40164026751963));
#38185=CARTESIAN_POINT('Ctrl Pts',(-4.85068927010199,-89.3545179709986,
-8.4016402675109));
#38186=CARTESIAN_POINT('Ctrl Pts',(-7.27603390513785,-89.1795179709986,
-4.20082013374671));
#38187=CARTESIAN_POINT('Ctrl Pts',(-9.70137854017372,-89.0045179709985,
1.74701493417668E-11));
#38188=CARTESIAN_POINT('Ctrl Pts',(-7.27603390512272,-88.8295179709986,
4.20082013377292));
#38189=CARTESIAN_POINT('Ctrl Pts',(-4.85068927007173,-88.6545179709986,
8.40164026752836));
#38190=CARTESIAN_POINT('Ctrl Pts',(1.5129078685785E-11,-88.4795179709986,
8.40164026751963));
#38191=CARTESIAN_POINT('Ctrl Pts',(4.85068927010198,-88.3045179709985,8.4016402675109));
#38192=CARTESIAN_POINT('Ctrl Pts',(7.27603390513785,-88.1295179709985,4.20082013374672));
#38193=CARTESIAN_POINT('Ctrl Pts',(9.70137854017372,-87.9545179709986,-1.74689612655491E-11));
#38194=CARTESIAN_POINT('Ctrl Pts',(7.27603390512273,-87.7795179709986,-4.20082013377291));
#38195=CARTESIAN_POINT('Ctrl Pts',(4.85068927007173,-87.6045179709986,-8.40164026752836));
#38196=CARTESIAN_POINT('Ctrl Pts',(-1.51301075899711E-11,-87.4295179709986,
-8.40164026751963));
#38197=CARTESIAN_POINT('Ctrl Pts',(-4.85068927010199,-87.2545179709986,
-8.4016402675109));
#38198=CARTESIAN_POINT('Ctrl Pts',(-7.27603390513785,-87.0795179709986,
-4.20082013374671));
#38199=CARTESIAN_POINT('Ctrl Pts',(-9.70137854017372,-86.9045179709986,
1.74701493417668E-11));
#38200=CARTESIAN_POINT('Ctrl Pts',(-7.27603390512272,-86.7295179709986,
4.20082013377292));
#38201=CARTESIAN_POINT('Ctrl Pts',(-4.85068927007173,-86.5545179709986,
8.40164026752836));
#38202=CARTESIAN_POINT('Ctrl Pts',(1.5129078685785E-11,-86.3795179709986,
8.40164026751963));
#38203=CARTESIAN_POINT('Ctrl Pts',(4.85068927010198,-86.2045179709986,8.4016402675109));
#38204=CARTESIAN_POINT('Ctrl Pts',(7.27603390513785,-86.0295179709986,4.20082013374672));
#38205=CARTESIAN_POINT('Ctrl Pts',(9.70137854017372,-85.8545179709986,-1.74689612655491E-11));
#38206=CARTESIAN_POINT('Ctrl Pts',(7.27603390512273,-85.6795179709986,-4.20082013377291));
#38207=CARTESIAN_POINT('Ctrl Pts',(4.85068927007173,-85.5045179709986,-8.40164026752836));
#38208=CARTESIAN_POINT('Ctrl Pts',(-1.51301075899711E-11,-85.3295179709986,
-8.40164026751963));
#38209=CARTESIAN_POINT('Ctrl Pts',(-4.85068927010199,-85.1545179709986,
-8.4016402675109));
#38210=CARTESIAN_POINT('Ctrl Pts',(-7.27603390513785,-84.9795179709986,
-4.20082013374671));
#38211=CARTESIAN_POINT('Ctrl Pts',(-9.70137854017372,-84.8045179709986,
1.74701493417668E-11));
#38212=CARTESIAN_POINT('Ctrl Pts',(-7.27603390512272,-84.6295179709986,
4.20082013377292));
#38213=CARTESIAN_POINT('Ctrl Pts',(-4.85068927007173,-84.4545179709986,
8.40164026752836));
#38214=CARTESIAN_POINT('Ctrl Pts',(1.5129078685785E-11,-84.2795179709986,
8.40164026751963));
#38215=CARTESIAN_POINT('Ctrl Pts',(4.85068927010198,-84.1045179709986,8.4016402675109));
#38216=CARTESIAN_POINT('Ctrl Pts',(7.27603390513785,-83.9295179709986,4.20082013374672));
#38217=CARTESIAN_POINT('Ctrl Pts',(9.70137854017372,-83.7545179709985,-1.74689612655491E-11));
#38218=CARTESIAN_POINT('Ctrl Pts',(7.27603390512273,-83.5795179709986,-4.20082013377291));
#38219=CARTESIAN_POINT('Ctrl Pts',(4.85068927007173,-83.4045179709986,-8.40164026752836));
#38220=CARTESIAN_POINT('Ctrl Pts',(-1.51301075899711E-11,-83.2295179709986,
-8.40164026751963));
#38221=CARTESIAN_POINT('Ctrl Pts',(-4.85068927010199,-83.0545179709986,
-8.4016402675109));
#38222=CARTESIAN_POINT('Ctrl Pts',(-7.27603390513785,-82.8795179709986,
-4.20082013374671));
#38223=CARTESIAN_POINT('Ctrl Pts',(-9.70137854017372,-82.7045179709986,
1.74701493417668E-11));
#38224=CARTESIAN_POINT('Ctrl Pts',(-7.27603390512272,-82.5295179709986,
4.20082013377292));
#38225=CARTESIAN_POINT('Ctrl Pts',(-4.85068927007173,-82.3545179709986,
8.40164026752836));
#38226=CARTESIAN_POINT('Ctrl Pts',(1.5129078685785E-11,-82.1795179709986,
8.40164026751963));
#38227=CARTESIAN_POINT('Ctrl Pts',(4.85068927010198,-82.0045179709986,8.4016402675109));
#38228=CARTESIAN_POINT('Ctrl Pts',(7.27603390513785,-81.8295179709986,4.20082013374672));
#38229=CARTESIAN_POINT('Ctrl Pts',(9.70137854017372,-81.6545179709986,-1.74689612655491E-11));
#38230=CARTESIAN_POINT('Ctrl Pts',(7.27603390512273,-81.4795179709986,-4.20082013377291));
#38231=CARTESIAN_POINT('Ctrl Pts',(4.85068927007173,-81.3045179709986,-8.40164026752836));
#38232=CARTESIAN_POINT('Ctrl Pts',(-1.51301075899711E-11,-81.1295179709986,
-8.40164026751963));
#38233=CARTESIAN_POINT('Ctrl Pts',(-4.85068927010199,-80.9545179709986,
-8.4016402675109));
#38234=CARTESIAN_POINT('Ctrl Pts',(-7.27603390513785,-80.7795179709986,
-4.20082013374671));
#38235=CARTESIAN_POINT('Ctrl Pts',(-9.70137854017372,-80.6045179709986,
1.74701493417668E-11));
#38236=CARTESIAN_POINT('Ctrl Pts',(-7.27603390512272,-80.4295179709986,
4.20082013377292));
#38237=CARTESIAN_POINT('Ctrl Pts',(-4.85068927007173,-80.2545179709986,
8.40164026752836));
#38238=CARTESIAN_POINT('Ctrl Pts',(1.5129078685785E-11,-80.0795179709986,
8.40164026751963));
#38239=CARTESIAN_POINT('Ctrl Pts',(4.85068927010198,-79.9045179709986,8.4016402675109));
#38240=CARTESIAN_POINT('Ctrl Pts',(7.27603390513785,-79.7295179709986,4.20082013374672));
#38241=CARTESIAN_POINT('Ctrl Pts',(9.70137854017372,-79.5545179709986,-1.74689612655491E-11));
#38242=CARTESIAN_POINT('Ctrl Pts',(7.27603390512273,-79.3795179709986,-4.20082013377291));
#38243=CARTESIAN_POINT('Ctrl Pts',(4.85068927007173,-79.2045179709986,-8.40164026752836));
#38244=CARTESIAN_POINT('Ctrl Pts',(-1.51301075899711E-11,-79.0295179709986,
-8.40164026751963));
#38245=CARTESIAN_POINT('Ctrl Pts',(-4.85068927010199,-78.8545179709986,
-8.4016402675109));
#38246=CARTESIAN_POINT('Ctrl Pts',(-7.27603390513785,-78.6795179709986,
-4.20082013374671));
#38247=CARTESIAN_POINT('Ctrl Pts',(-9.70137854017372,-78.5045179709986,
1.74701493417668E-11));
#38248=CARTESIAN_POINT('Ctrl Pts',(-7.27603390512272,-78.3295179709986,
4.20082013377292));
#38249=CARTESIAN_POINT('Ctrl Pts',(-4.85068927007173,-78.1545179709986,
8.40164026752836));
#38250=CARTESIAN_POINT('Ctrl Pts',(1.5129078685785E-11,-77.9795179709986,
8.40164026751963));
#38251=CARTESIAN_POINT('Ctrl Pts',(4.85068927010198,-77.8045179709986,8.4016402675109));
#38252=CARTESIAN_POINT('Ctrl Pts',(7.27603390513785,-77.6295179709986,4.20082013374672));
#38253=CARTESIAN_POINT('Ctrl Pts',(9.70137854017372,-77.4545179709986,-1.74689612655491E-11));
#38254=CARTESIAN_POINT('Ctrl Pts',(7.27603390512273,-77.2795179709986,-4.20082013377291));
#38255=CARTESIAN_POINT('Ctrl Pts',(4.85068927007173,-77.1045179709986,-8.40164026752836));
#38256=CARTESIAN_POINT('Ctrl Pts',(-1.51301075899711E-11,-76.9295179709986,
-8.40164026751963));
#38257=CARTESIAN_POINT('Ctrl Pts',(-4.85068927010199,-76.7545179709986,
-8.4016402675109));
#38258=CARTESIAN_POINT('Ctrl Pts',(-7.27603390513785,-76.5795179709986,
-4.20082013374671));
#38259=CARTESIAN_POINT('Ctrl Pts',(-9.70137854017372,-76.4045179709986,
1.74701493417668E-11));
#38260=CARTESIAN_POINT('Ctrl Pts',(-7.27603390512272,-76.2295179709986,
4.20082013377292));
#38261=CARTESIAN_POINT('Ctrl Pts',(-4.85068927007173,-76.0545179709986,
8.40164026752836));
#38262=CARTESIAN_POINT('Ctrl Pts',(1.5129078685785E-11,-75.8795179709986,
8.40164026751963));
#38263=CARTESIAN_POINT('Ctrl Pts',(4.85068927010198,-75.7045179709986,8.4016402675109));
#38264=CARTESIAN_POINT('Ctrl Pts',(7.27603390513785,-75.5295179709986,4.20082013374672));
#38265=CARTESIAN_POINT('Ctrl Pts',(9.70137854017372,-75.3545179709986,-1.74689612655491E-11));
#38266=CARTESIAN_POINT('Ctrl Pts',(7.27603390512273,-75.1795179709986,-4.20082013377291));
#38267=CARTESIAN_POINT('Ctrl Pts',(4.85068927007173,-75.0045179709986,-8.40164026752836));
#38268=CARTESIAN_POINT('Ctrl Pts',(-1.51301075899711E-11,-74.8295179709986,
-8.40164026751963));
#38269=CARTESIAN_POINT('Ctrl Pts',(-4.85068927010199,-74.6545179709986,
-8.4016402675109));
#38270=CARTESIAN_POINT('Ctrl Pts',(-7.27603390513785,-74.4795179709986,
-4.20082013374671));
#38271=CARTESIAN_POINT('Ctrl Pts',(-9.70137854017372,-74.3045179709986,
1.74701493417668E-11));
#38272=CARTESIAN_POINT('Ctrl Pts',(-7.27603390512272,-74.1295179709986,
4.20082013377292));
#38273=CARTESIAN_POINT('Ctrl Pts',(-4.85068927007173,-73.9545179709986,
8.40164026752836));
#38274=CARTESIAN_POINT('Ctrl Pts',(1.5129078685785E-11,-73.7795179709986,
8.40164026751963));
#38275=CARTESIAN_POINT('Ctrl Pts',(4.85068927010198,-73.6045179709986,8.4016402675109));
#38276=CARTESIAN_POINT('Ctrl Pts',(7.27603390513785,-73.4295179709986,4.20082013374672));
#38277=CARTESIAN_POINT('Ctrl Pts',(9.70137854017372,-73.2545179709986,-1.74689612655491E-11));
#38278=CARTESIAN_POINT('Ctrl Pts',(7.27603390512273,-73.0795179709986,-4.20082013377291));
#38279=CARTESIAN_POINT('Ctrl Pts',(4.85068927007173,-72.9045179709986,-8.40164026752836));
#38280=CARTESIAN_POINT('Ctrl Pts',(-1.51301075899711E-11,-72.7295179709986,
-8.40164026751963));
#38281=CARTESIAN_POINT('Ctrl Pts',(-4.85068927010199,-72.5545179709986,
-8.4016402675109));
#38282=CARTESIAN_POINT('Ctrl Pts',(-7.27603390513785,-72.3795179709986,
-4.20082013374671));
#38283=CARTESIAN_POINT('Ctrl Pts',(-9.70137854017372,-72.2045179709986,
1.74701493417668E-11));
#38284=CARTESIAN_POINT('Ctrl Pts',(-7.27603390512272,-72.0295179709986,
4.20082013377292));
#38285=CARTESIAN_POINT('Ctrl Pts',(-4.85068927007173,-71.8545179709986,
8.40164026752836));
#38286=CARTESIAN_POINT('Ctrl Pts',(1.5129078685785E-11,-71.6795179709986,
8.40164026751963));
#38287=CARTESIAN_POINT('Ctrl Pts',(4.85068927010198,-71.5045179709986,8.4016402675109));
#38288=CARTESIAN_POINT('Ctrl Pts',(7.27603390513785,-71.3295179709986,4.20082013374672));
#38289=CARTESIAN_POINT('Ctrl Pts',(9.70137854017372,-71.1545179709986,-1.74689612655491E-11));
#38290=CARTESIAN_POINT('Ctrl Pts',(7.27603390512273,-70.9795179709986,-4.20082013377291));
#38291=CARTESIAN_POINT('Ctrl Pts',(4.85068927007173,-70.8045179709986,-8.40164026752836));
#38292=CARTESIAN_POINT('Ctrl Pts',(-1.51301075899711E-11,-70.6295179709986,
-8.40164026751963));
#38293=CARTESIAN_POINT('Ctrl Pts',(-4.85068927010199,-70.4545179709986,
-8.4016402675109));
#38294=CARTESIAN_POINT('Ctrl Pts',(-7.27603390513785,-70.2795179709986,
-4.20082013374671));
#38295=CARTESIAN_POINT('Ctrl Pts',(-9.70137854017372,-70.1045179709986,
1.74701493417668E-11));
#38296=CARTESIAN_POINT('Ctrl Pts',(-7.27603390512272,-69.9295179709986,
4.20082013377292));
#38297=CARTESIAN_POINT('Ctrl Pts',(-4.85068927007173,-69.7545179709986,
8.40164026752836));
#38298=CARTESIAN_POINT('Ctrl Pts',(1.5129078685785E-11,-69.5795179709986,
8.40164026751963));
#38299=CARTESIAN_POINT('Ctrl Pts',(4.85068927010198,-69.4045179709986,8.4016402675109));
#38300=CARTESIAN_POINT('Ctrl Pts',(7.27603390513785,-69.2295179709986,4.20082013374672));
#38301=CARTESIAN_POINT('Ctrl Pts',(9.70137854017372,-69.0545179709986,-1.74689612655491E-11));
#38302=CARTESIAN_POINT('Ctrl Pts',(7.27603390512273,-68.8795179709986,-4.20082013377291));
#38303=CARTESIAN_POINT('Ctrl Pts',(4.85068927007173,-68.7045179709986,-8.40164026752836));
#38304=CARTESIAN_POINT('Ctrl Pts',(-1.51301075899711E-11,-68.5295179709986,
-8.40164026751963));
#38305=CARTESIAN_POINT('Ctrl Pts',(-4.85068927010199,-68.3545179709986,
-8.4016402675109));
#38306=CARTESIAN_POINT('Ctrl Pts',(-7.27603390513785,-68.1795179709986,
-4.20082013374671));
#38307=CARTESIAN_POINT('Ctrl Pts',(-9.70137854017372,-68.0045179709986,
1.74701493417668E-11));
#38308=CARTESIAN_POINT('Ctrl Pts',(-7.27603390512272,-67.8295179709986,
4.20082013377292));
#38309=CARTESIAN_POINT('Ctrl Pts',(-4.85068927007173,-67.6545179709986,
8.40164026752836));
#38310=CARTESIAN_POINT('Ctrl Pts',(1.5129078685785E-11,-67.4795179709986,
8.40164026751963));
#38311=CARTESIAN_POINT('Ctrl Pts',(4.85068927010198,-67.3045179709986,8.4016402675109));
#38312=CARTESIAN_POINT('Ctrl Pts',(7.27603390513785,-67.1295179709986,4.20082013374672));
#38313=CARTESIAN_POINT('Ctrl Pts',(9.70137854017372,-66.9545179709986,-1.74689612655491E-11));
#38314=CARTESIAN_POINT('Ctrl Pts',(7.27603390512273,-66.7795179709986,-4.20082013377291));
#38315=CARTESIAN_POINT('Ctrl Pts',(4.85068927007173,-66.6045179709986,-8.40164026752836));
#38316=CARTESIAN_POINT('Ctrl Pts',(-1.51301075899711E-11,-66.4295179709986,
-8.40164026751963));
#38317=CARTESIAN_POINT('Ctrl Pts',(-4.85068927010199,-66.2545179709986,
-8.4016402675109));
#38318=CARTESIAN_POINT('Ctrl Pts',(-7.27603390513785,-66.0795179709986,
-4.20082013374671));
#38319=CARTESIAN_POINT('Ctrl Pts',(-9.70137854017372,-65.9045179709986,
1.74701493417668E-11));
#38320=CARTESIAN_POINT('Ctrl Pts',(-7.27603390512272,-65.7295179709986,
4.20082013377292));
#38321=CARTESIAN_POINT('Ctrl Pts',(-4.85068927007173,-65.5545179709986,
8.40164026752836));
#38322=CARTESIAN_POINT('Ctrl Pts',(1.5129078685785E-11,-65.3795179709986,
8.40164026751963));
#38323=CARTESIAN_POINT('Ctrl Pts',(4.85068927010198,-65.2045179709986,8.4016402675109));
#38324=CARTESIAN_POINT('Ctrl Pts',(7.27603390513785,-65.0295179709986,4.20082013374672));
#38325=CARTESIAN_POINT('Ctrl Pts',(9.70137854017372,-64.8545179709986,-1.74689612655491E-11));
#38326=CARTESIAN_POINT('Ctrl Pts',(7.27603390512273,-64.6795179709986,-4.20082013377291));
#38327=CARTESIAN_POINT('Ctrl Pts',(4.85068927007173,-64.5045179709986,-8.40164026752836));
#38328=CARTESIAN_POINT('Ctrl Pts',(-1.51301075899711E-11,-64.3295179709986,
-8.40164026751963));
#38329=CARTESIAN_POINT('Ctrl Pts',(-4.85068927010199,-64.1545179709986,
-8.4016402675109));
#38330=CARTESIAN_POINT('Ctrl Pts',(-7.27603390513785,-63.9795179709986,
-4.20082013374671));
#38331=CARTESIAN_POINT('Ctrl Pts',(-9.70137854017372,-63.8045179709986,
1.74701493417668E-11));
#38332=CARTESIAN_POINT('Ctrl Pts',(-7.27603390512272,-63.6295179709986,
4.20082013377292));
#38333=CARTESIAN_POINT('Ctrl Pts',(-4.85068927007173,-63.4545179709986,
8.40164026752836));
#38334=CARTESIAN_POINT('Ctrl Pts',(1.5129078685785E-11,-63.2795179709986,
8.40164026751963));
#38335=CARTESIAN_POINT('Ctrl Pts',(4.85068927010198,-63.1045179709986,8.4016402675109));
#38336=CARTESIAN_POINT('Ctrl Pts',(7.27603390513785,-62.9295179709986,4.20082013374672));
#38337=CARTESIAN_POINT('Ctrl Pts',(9.70137854017372,-62.7545179709986,-1.74689612655491E-11));
#38338=CARTESIAN_POINT('Ctrl Pts',(7.27603390512273,-62.5795179709986,-4.20082013377291));
#38339=CARTESIAN_POINT('Ctrl Pts',(4.85068927007173,-62.4045179709986,-8.40164026752836));
#38340=CARTESIAN_POINT('Ctrl Pts',(-1.51301075899711E-11,-62.2295179709986,
-8.40164026751963));
#38341=CARTESIAN_POINT('Ctrl Pts',(-4.85068927010199,-62.0545179709986,
-8.4016402675109));
#38342=CARTESIAN_POINT('Ctrl Pts',(-7.27603390513785,-61.8795179709986,
-4.20082013374671));
#38343=CARTESIAN_POINT('Ctrl Pts',(-9.70137854017372,-61.7045179709986,
1.74701493417668E-11));
#38344=CARTESIAN_POINT('Ctrl Pts',(-7.27603390512272,-61.5295179709986,
4.20082013377292));
#38345=CARTESIAN_POINT('Ctrl Pts',(-4.85068927007173,-61.3545179709986,
8.40164026752836));
#38346=CARTESIAN_POINT('Ctrl Pts',(1.5129078685785E-11,-61.1795179709986,
8.40164026751963));
#38347=CARTESIAN_POINT('Ctrl Pts',(4.85068927010198,-61.0045179709986,8.4016402675109));
#38348=CARTESIAN_POINT('Ctrl Pts',(7.27603390513785,-60.8295179709986,4.20082013374672));
#38349=CARTESIAN_POINT('Ctrl Pts',(9.70137854017372,-60.6545179709986,-1.74689612655491E-11));
#38350=CARTESIAN_POINT('Ctrl Pts',(7.27603390512273,-60.4795179709986,-4.20082013377291));
#38351=CARTESIAN_POINT('Ctrl Pts',(4.85068927007173,-60.3045179709986,-8.40164026752836));
#38352=CARTESIAN_POINT('Ctrl Pts',(-1.51301075899711E-11,-60.1295179709986,
-8.40164026751963));
#38353=CARTESIAN_POINT('Ctrl Pts',(-4.85068927010199,-59.9545179709986,
-8.4016402675109));
#38354=CARTESIAN_POINT('Ctrl Pts',(-7.27603390513785,-59.7795179709986,
-4.20082013374671));
#38355=CARTESIAN_POINT('Ctrl Pts',(-9.70137854017372,-59.6045179709986,
1.74701493417668E-11));
#38356=CARTESIAN_POINT('Ctrl Pts',(-7.27603390512272,-59.4295179709986,
4.20082013377292));
#38357=CARTESIAN_POINT('Ctrl Pts',(-4.85068927007173,-59.2545179709986,
8.40164026752836));
#38358=CARTESIAN_POINT('Ctrl Pts',(1.5129078685785E-11,-59.0795179709986,
8.40164026751963));
#38359=CARTESIAN_POINT('Ctrl Pts',(4.85068927010198,-58.9045179709986,8.4016402675109));
#38360=CARTESIAN_POINT('Ctrl Pts',(7.27603390513785,-58.7295179709986,4.20082013374672));
#38361=CARTESIAN_POINT('Ctrl Pts',(9.70137854017372,-58.5545179709986,-1.74689612655491E-11));
#38362=CARTESIAN_POINT('Ctrl Pts',(7.27603390512273,-58.3795179709986,-4.20082013377291));
#38363=CARTESIAN_POINT('Ctrl Pts',(4.85068927007173,-58.2045179709986,-8.40164026752836));
#38364=CARTESIAN_POINT('Ctrl Pts',(-1.51301075899711E-11,-58.0295179709986,
-8.40164026751963));
#38365=CARTESIAN_POINT('Ctrl Pts',(-4.85068927010199,-57.8545179709986,
-8.4016402675109));
#38366=CARTESIAN_POINT('Ctrl Pts',(-7.27603390513785,-57.6795179709986,
-4.20082013374671));
#38367=CARTESIAN_POINT('Ctrl Pts',(-9.70137854017372,-57.5045179709986,
1.74701493417668E-11));
#38368=CARTESIAN_POINT('Ctrl Pts',(-7.27603390512272,-57.3295179709986,
4.20082013377292));
#38369=CARTESIAN_POINT('Ctrl Pts',(-4.85068927007173,-57.1545179709986,
8.40164026752836));
#38370=CARTESIAN_POINT('Ctrl Pts',(1.5129078685785E-11,-56.9795179709986,
8.40164026751963));
#38371=CARTESIAN_POINT('Ctrl Pts',(4.85068927010198,-56.8045179709986,8.4016402675109));
#38372=CARTESIAN_POINT('Ctrl Pts',(7.27603390513785,-56.6295179709986,4.20082013374672));
#38373=CARTESIAN_POINT('Ctrl Pts',(9.70137854017372,-56.4545179709986,-1.74689612655491E-11));
#38374=CARTESIAN_POINT('Ctrl Pts',(7.27603390512273,-56.2795179709986,-4.20082013377291));
#38375=CARTESIAN_POINT('Ctrl Pts',(4.85068927007173,-56.1045179709986,-8.40164026752836));
#38376=CARTESIAN_POINT('Ctrl Pts',(-1.51301075899711E-11,-55.9295179709986,
-8.40164026751963));
#38377=CARTESIAN_POINT('Ctrl Pts',(-4.85068927010199,-55.7545179709987,
-8.4016402675109));
#38378=CARTESIAN_POINT('Ctrl Pts',(-7.27603390513785,-55.5795179709986,
-4.20082013374671));
#38379=CARTESIAN_POINT('Ctrl Pts',(-9.70137854017372,-55.4045179709986,
1.74701493417668E-11));
#38380=CARTESIAN_POINT('Ctrl Pts',(-7.27603390512272,-55.2295179709986,
4.20082013377292));
#38381=CARTESIAN_POINT('Ctrl Pts',(-4.85068927007173,-55.0545179709987,
8.40164026752836));
#38382=CARTESIAN_POINT('Ctrl Pts',(1.5129078685785E-11,-54.8795179709986,
8.40164026751963));
#38383=CARTESIAN_POINT('Ctrl Pts',(4.85068927010198,-54.7045179709987,8.4016402675109));
#38384=CARTESIAN_POINT('Ctrl Pts',(7.27603390513785,-54.5295179709986,4.20082013374672));
#38385=CARTESIAN_POINT('Ctrl Pts',(9.70137854017372,-54.3545179709986,-1.74689612655491E-11));
#38386=CARTESIAN_POINT('Ctrl Pts',(7.27603390512273,-54.1795179709986,-4.20082013377291));
#38387=CARTESIAN_POINT('Ctrl Pts',(4.85068927007173,-54.0045179709987,-8.40164026752836));
#38388=CARTESIAN_POINT('Ctrl Pts',(-1.51301075899711E-11,-53.8295179709986,
-8.40164026751963));
#38389=CARTESIAN_POINT('Ctrl Pts',(-4.85068927010199,-53.6545179709986,
-8.4016402675109));
#38390=CARTESIAN_POINT('Ctrl Pts',(-7.27603390513785,-53.4795179709987,
-4.20082013374671));
#38391=CARTESIAN_POINT('Ctrl Pts',(-9.70137854017372,-53.3045179709987,
1.74701493417668E-11));
#38392=CARTESIAN_POINT('Ctrl Pts',(-7.27603390512272,-53.1295179709986,
4.20082013377292));
#38393=CARTESIAN_POINT('Ctrl Pts',(-4.85068927007173,-52.9545179709987,
8.40164026752836));
#38394=CARTESIAN_POINT('Ctrl Pts',(1.5129078685785E-11,-52.7795179709986,
8.40164026751963));
#38395=CARTESIAN_POINT('Ctrl Pts',(4.85068927010198,-52.6045179709986,8.4016402675109));
#38396=CARTESIAN_POINT('Ctrl Pts',(7.27603390513785,-52.4295179709987,4.20082013374672));
#38397=CARTESIAN_POINT('Ctrl Pts',(9.70137854017372,-52.2545179709986,-1.74689612655491E-11));
#38398=CARTESIAN_POINT('Ctrl Pts',(7.27603390512273,-52.0795179709986,-4.20082013377291));
#38399=CARTESIAN_POINT('Ctrl Pts',(4.85068927007173,-51.9045179709987,-8.40164026752836));
#38400=CARTESIAN_POINT('Ctrl Pts',(-1.51301075899711E-11,-51.7295179709986,
-8.40164026751963));
#38401=CARTESIAN_POINT('Ctrl Pts',(-4.85068927010199,-51.5545179709986,
-8.4016402675109));
#38402=CARTESIAN_POINT('Ctrl Pts',(-7.27603390513785,-51.3795179709987,
-4.20082013374671));
#38403=CARTESIAN_POINT('Ctrl Pts',(-9.70137854017372,-51.2045179709987,
1.74701493417668E-11));
#38404=CARTESIAN_POINT('Ctrl Pts',(-7.27603390512272,-51.0295179709986,
4.20082013377292));
#38405=CARTESIAN_POINT('Ctrl Pts',(-4.85068927007173,-50.8545179709987,
8.40164026752836));
#38406=CARTESIAN_POINT('Ctrl Pts',(1.5129078685785E-11,-50.6795179709987,
8.40164026751963));
#38407=CARTESIAN_POINT('Ctrl Pts',(4.85068927010198,-50.5045179709986,8.4016402675109));
#38408=CARTESIAN_POINT('Ctrl Pts',(7.27603390513785,-50.3295179709987,4.20082013374672));
#38409=CARTESIAN_POINT('Ctrl Pts',(9.70137854017372,-50.1545179709987,-1.74689612655491E-11));
#38410=CARTESIAN_POINT('Ctrl Pts',(7.27603390512273,-49.9795179709986,-4.20082013377291));
#38411=CARTESIAN_POINT('Ctrl Pts',(4.85068927007173,-49.8045179709986,-8.40164026752836));
#38412=CARTESIAN_POINT('Ctrl Pts',(-1.51301075899711E-11,-49.6295179709987,
-8.40164026751963));
#38413=CARTESIAN_POINT('Ctrl Pts',(-4.85068927010199,-49.4545179709986,
-8.4016402675109));
#38414=CARTESIAN_POINT('Ctrl Pts',(-7.27603390513785,-49.2795179709986,
-4.20082013374671));
#38415=CARTESIAN_POINT('Ctrl Pts',(-9.70137854017372,-49.1045179709987,
1.74701493417668E-11));
#38416=CARTESIAN_POINT('Ctrl Pts',(-7.27603390512272,-48.9295179709987,
4.20082013377292));
#38417=CARTESIAN_POINT('Ctrl Pts',(-4.85068927007173,-48.7545179709986,
8.40164026752836));
#38418=CARTESIAN_POINT('Ctrl Pts',(1.5129078685785E-11,-48.5795179709987,
8.40164026751963));
#38419=CARTESIAN_POINT('Ctrl Pts',(4.85068927010198,-48.4045179709987,8.4016402675109));
#38420=CARTESIAN_POINT('Ctrl Pts',(7.27603390513785,-48.2295179709986,4.20082013374672));
#38421=CARTESIAN_POINT('Ctrl Pts',(9.70137854017372,-48.0545179709987,-1.74689612655491E-11));
#38422=CARTESIAN_POINT('Ctrl Pts',(7.27603390512273,-47.8795179709987,-4.20082013377291));
#38423=CARTESIAN_POINT('Ctrl Pts',(4.85068927007173,-47.7045179709986,-8.40164026752836));
#38424=CARTESIAN_POINT('Ctrl Pts',(-1.51301075899711E-11,-47.5295179709987,
-8.40164026751963));
#38425=CARTESIAN_POINT('Ctrl Pts',(-4.85068927010199,-47.3545179709987,
-8.4016402675109));
#38426=CARTESIAN_POINT('Ctrl Pts',(-7.27603390513785,-47.1795179709986,
-4.20082013374671));
#38427=CARTESIAN_POINT('Ctrl Pts',(-9.70137854017372,-47.0045179709987,
1.74701493417668E-11));
#38428=CARTESIAN_POINT('Ctrl Pts',(-7.27603390512272,-46.8295179709987,
4.20082013377292));
#38429=CARTESIAN_POINT('Ctrl Pts',(-4.85068927007173,-46.6545179709987,
8.40164026752836));
#38430=CARTESIAN_POINT('Ctrl Pts',(1.5129078685785E-11,-46.4795179709987,
8.40164026751963));
#38431=CARTESIAN_POINT('Ctrl Pts',(4.85068927010198,-46.3045179709987,8.4016402675109));
#38432=CARTESIAN_POINT('Ctrl Pts',(7.27603390513785,-46.1295179709986,4.20082013374672));
#38433=CARTESIAN_POINT('Ctrl Pts',(9.70137854017372,-45.9545179709987,-1.74689612655491E-11));
#38434=CARTESIAN_POINT('Ctrl Pts',(7.27603390512273,-45.7795179709987,-4.20082013377291));
#38435=CARTESIAN_POINT('Ctrl Pts',(4.85068927007173,-45.6045179709986,-8.40164026752836));
#38436=CARTESIAN_POINT('Ctrl Pts',(-1.51301075899711E-11,-45.4295179709987,
-8.40164026751963));
#38437=CARTESIAN_POINT('Ctrl Pts',(-4.85068927010199,-45.2545179709987,
-8.4016402675109));
#38438=CARTESIAN_POINT('Ctrl Pts',(-7.27603390513785,-45.0795179709987,
-4.20082013374671));
#38439=CARTESIAN_POINT('Ctrl Pts',(-9.70137854017372,-44.9045179709986,
1.74701493417668E-11));
#38440=CARTESIAN_POINT('Ctrl Pts',(-7.27603390512272,-44.7295179709987,
4.20082013377292));
#38441=CARTESIAN_POINT('Ctrl Pts',(-4.85068927007173,-44.5545179709987,
8.40164026752836));
#38442=CARTESIAN_POINT('Ctrl Pts',(1.5129078685785E-11,-44.3795179709986,
8.40164026751963));
#38443=CARTESIAN_POINT('Ctrl Pts',(4.85068927010198,-44.2045179709987,8.4016402675109));
#38444=CARTESIAN_POINT('Ctrl Pts',(7.27603390513785,-44.0295179709987,4.20082013374672));
#38445=CARTESIAN_POINT('Ctrl Pts',(9.70137854017372,-43.8545179709986,-1.74689612655491E-11));
#38446=CARTESIAN_POINT('Ctrl Pts',(7.27603390512273,-43.6795179709987,-4.20082013377291));
#38447=CARTESIAN_POINT('Ctrl Pts',(4.85068927007173,-43.5045179709987,-8.40164026752836));
#38448=CARTESIAN_POINT('Ctrl Pts',(-1.51301075899711E-11,-43.3295179709987,
-8.40164026751963));
#38449=CARTESIAN_POINT('Ctrl Pts',(-1.78726082715848E-11,-212.63675111262,
-9.92453123331945));
#38450=CARTESIAN_POINT('Ctrl Pts',(-5.7299307791557,-212.46175111262,-9.92453123330913));
#38451=CARTESIAN_POINT('Ctrl Pts',(-8.59489616871569,-212.28675111262,-4.96226561664425));
#38452=CARTESIAN_POINT('Ctrl Pts',(-11.4598615582757,-212.11175111262,2.06368086793017E-11));
#38453=CARTESIAN_POINT('Ctrl Pts',(-8.59489616869782,-211.93675111262,4.9622656166752));
#38454=CARTESIAN_POINT('Ctrl Pts',(-5.72993077911996,-211.76175111262,9.92453123332977));
#38455=CARTESIAN_POINT('Ctrl Pts',(1.7871392867044E-11,-211.58675111262,
9.92453123331945));
#38456=CARTESIAN_POINT('Ctrl Pts',(5.7299307791557,-211.41175111262,9.92453123330913));
#38457=CARTESIAN_POINT('Ctrl Pts',(8.59489616871569,-211.23675111262,4.96226561664425));
#38458=CARTESIAN_POINT('Ctrl Pts',(11.4598615582757,-211.06175111262,-2.06354052510241E-11));
#38459=CARTESIAN_POINT('Ctrl Pts',(8.59489616869782,-210.88675111262,-4.9622656166752));
#38460=CARTESIAN_POINT('Ctrl Pts',(5.72993077911996,-210.71175111262,-9.92453123332976));
#38461=CARTESIAN_POINT('Ctrl Pts',(-1.78726082715848E-11,-210.53675111262,
-9.92453123331945));
#38462=CARTESIAN_POINT('Ctrl Pts',(-5.7299307791557,-210.36175111262,-9.92453123330913));
#38463=CARTESIAN_POINT('Ctrl Pts',(-8.59489616871569,-210.18675111262,-4.96226561664425));
#38464=CARTESIAN_POINT('Ctrl Pts',(-11.4598615582757,-210.01175111262,2.06368086793017E-11));
#38465=CARTESIAN_POINT('Ctrl Pts',(-8.59489616869782,-209.83675111262,4.9622656166752));
#38466=CARTESIAN_POINT('Ctrl Pts',(-5.72993077911996,-209.66175111262,9.92453123332977));
#38467=CARTESIAN_POINT('Ctrl Pts',(1.7871392867044E-11,-209.48675111262,
9.92453123331945));
#38468=CARTESIAN_POINT('Ctrl Pts',(5.7299307791557,-209.31175111262,9.92453123330913));
#38469=CARTESIAN_POINT('Ctrl Pts',(8.59489616871569,-209.13675111262,4.96226561664425));
#38470=CARTESIAN_POINT('Ctrl Pts',(11.4598615582757,-208.96175111262,-2.06354052510241E-11));
#38471=CARTESIAN_POINT('Ctrl Pts',(8.59489616869782,-208.78675111262,-4.9622656166752));
#38472=CARTESIAN_POINT('Ctrl Pts',(5.72993077911996,-208.61175111262,-9.92453123332976));
#38473=CARTESIAN_POINT('Ctrl Pts',(-1.78726082715848E-11,-208.43675111262,
-9.92453123331945));
#38474=CARTESIAN_POINT('Ctrl Pts',(-5.7299307791557,-208.26175111262,-9.92453123330913));
#38475=CARTESIAN_POINT('Ctrl Pts',(-8.59489616871569,-208.08675111262,-4.96226561664425));
#38476=CARTESIAN_POINT('Ctrl Pts',(-11.4598615582757,-207.91175111262,2.06368086793017E-11));
#38477=CARTESIAN_POINT('Ctrl Pts',(-8.59489616869782,-207.73675111262,4.9622656166752));
#38478=CARTESIAN_POINT('Ctrl Pts',(-5.72993077911996,-207.56175111262,9.92453123332977));
#38479=CARTESIAN_POINT('Ctrl Pts',(1.7871392867044E-11,-207.38675111262,
9.92453123331945));
#38480=CARTESIAN_POINT('Ctrl Pts',(5.7299307791557,-207.21175111262,9.92453123330913));
#38481=CARTESIAN_POINT('Ctrl Pts',(8.59489616871569,-207.03675111262,4.96226561664425));
#38482=CARTESIAN_POINT('Ctrl Pts',(11.4598615582757,-206.86175111262,-2.06354052510241E-11));
#38483=CARTESIAN_POINT('Ctrl Pts',(8.59489616869782,-206.68675111262,-4.9622656166752));
#38484=CARTESIAN_POINT('Ctrl Pts',(5.72993077911996,-206.51175111262,-9.92453123332976));
#38485=CARTESIAN_POINT('Ctrl Pts',(-1.78726082715848E-11,-206.33675111262,
-9.92453123331945));
#38486=CARTESIAN_POINT('Ctrl Pts',(-5.7299307791557,-206.16175111262,-9.92453123330913));
#38487=CARTESIAN_POINT('Ctrl Pts',(-8.59489616871569,-205.98675111262,-4.96226561664425));
#38488=CARTESIAN_POINT('Ctrl Pts',(-11.4598615582757,-205.81175111262,2.06368086793017E-11));
#38489=CARTESIAN_POINT('Ctrl Pts',(-8.59489616869782,-205.63675111262,4.9622656166752));
#38490=CARTESIAN_POINT('Ctrl Pts',(-5.72993077911996,-205.46175111262,9.92453123332977));
#38491=CARTESIAN_POINT('Ctrl Pts',(1.7871392867044E-11,-205.28675111262,
9.92453123331945));
#38492=CARTESIAN_POINT('Ctrl Pts',(5.7299307791557,-205.11175111262,9.92453123330913));
#38493=CARTESIAN_POINT('Ctrl Pts',(8.59489616871569,-204.93675111262,4.96226561664425));
#38494=CARTESIAN_POINT('Ctrl Pts',(11.4598615582757,-204.76175111262,-2.06354052510241E-11));
#38495=CARTESIAN_POINT('Ctrl Pts',(8.59489616869782,-204.58675111262,-4.9622656166752));
#38496=CARTESIAN_POINT('Ctrl Pts',(5.72993077911996,-204.41175111262,-9.92453123332976));
#38497=CARTESIAN_POINT('Ctrl Pts',(-1.78726082715848E-11,-204.23675111262,
-9.92453123331945));
#38498=CARTESIAN_POINT('Ctrl Pts',(-5.7299307791557,-204.06175111262,-9.92453123330913));
#38499=CARTESIAN_POINT('Ctrl Pts',(-8.59489616871569,-203.88675111262,-4.96226561664425));
#38500=CARTESIAN_POINT('Ctrl Pts',(-11.4598615582757,-203.71175111262,2.06368086793017E-11));
#38501=CARTESIAN_POINT('Ctrl Pts',(-8.59489616869782,-203.53675111262,4.9622656166752));
#38502=CARTESIAN_POINT('Ctrl Pts',(-5.72993077911996,-203.36175111262,9.92453123332977));
#38503=CARTESIAN_POINT('Ctrl Pts',(1.7871392867044E-11,-203.18675111262,
9.92453123331945));
#38504=CARTESIAN_POINT('Ctrl Pts',(5.7299307791557,-203.01175111262,9.92453123330913));
#38505=CARTESIAN_POINT('Ctrl Pts',(8.59489616871569,-202.83675111262,4.96226561664425));
#38506=CARTESIAN_POINT('Ctrl Pts',(11.4598615582757,-202.66175111262,-2.06354052510241E-11));
#38507=CARTESIAN_POINT('Ctrl Pts',(8.59489616869782,-202.48675111262,-4.9622656166752));
#38508=CARTESIAN_POINT('Ctrl Pts',(5.72993077911996,-202.31175111262,-9.92453123332976));
#38509=CARTESIAN_POINT('Ctrl Pts',(-1.78726082715848E-11,-202.13675111262,
-9.92453123331945));
#38510=CARTESIAN_POINT('Ctrl Pts',(-5.7299307791557,-201.96175111262,-9.92453123330913));
#38511=CARTESIAN_POINT('Ctrl Pts',(-8.59489616871569,-201.78675111262,-4.96226561664425));
#38512=CARTESIAN_POINT('Ctrl Pts',(-11.4598615582757,-201.61175111262,2.06368086793017E-11));
#38513=CARTESIAN_POINT('Ctrl Pts',(-8.59489616869782,-201.43675111262,4.9622656166752));
#38514=CARTESIAN_POINT('Ctrl Pts',(-5.72993077911996,-201.26175111262,9.92453123332977));
#38515=CARTESIAN_POINT('Ctrl Pts',(1.7871392867044E-11,-201.08675111262,
9.92453123331945));
#38516=CARTESIAN_POINT('Ctrl Pts',(5.7299307791557,-200.91175111262,9.92453123330913));
#38517=CARTESIAN_POINT('Ctrl Pts',(8.59489616871569,-200.73675111262,4.96226561664425));
#38518=CARTESIAN_POINT('Ctrl Pts',(11.4598615582757,-200.56175111262,-2.06354052510241E-11));
#38519=CARTESIAN_POINT('Ctrl Pts',(8.59489616869782,-200.38675111262,-4.9622656166752));
#38520=CARTESIAN_POINT('Ctrl Pts',(5.72993077911996,-200.21175111262,-9.92453123332976));
#38521=CARTESIAN_POINT('Ctrl Pts',(-1.78726082715848E-11,-200.03675111262,
-9.92453123331945));
#38522=CARTESIAN_POINT('Ctrl Pts',(-5.7299307791557,-199.86175111262,-9.92453123330913));
#38523=CARTESIAN_POINT('Ctrl Pts',(-8.59489616871569,-199.68675111262,-4.96226561664425));
#38524=CARTESIAN_POINT('Ctrl Pts',(-11.4598615582757,-199.51175111262,2.06368086793017E-11));
#38525=CARTESIAN_POINT('Ctrl Pts',(-8.59489616869782,-199.33675111262,4.9622656166752));
#38526=CARTESIAN_POINT('Ctrl Pts',(-5.72993077911996,-199.16175111262,9.92453123332977));
#38527=CARTESIAN_POINT('Ctrl Pts',(1.7871392867044E-11,-198.98675111262,
9.92453123331945));
#38528=CARTESIAN_POINT('Ctrl Pts',(5.7299307791557,-198.81175111262,9.92453123330913));
#38529=CARTESIAN_POINT('Ctrl Pts',(8.59489616871569,-198.63675111262,4.96226561664425));
#38530=CARTESIAN_POINT('Ctrl Pts',(11.4598615582757,-198.46175111262,-2.06354052510241E-11));
#38531=CARTESIAN_POINT('Ctrl Pts',(8.59489616869782,-198.28675111262,-4.9622656166752));
#38532=CARTESIAN_POINT('Ctrl Pts',(5.72993077911996,-198.11175111262,-9.92453123332976));
#38533=CARTESIAN_POINT('Ctrl Pts',(-1.78726082715848E-11,-197.93675111262,
-9.92453123331945));
#38534=CARTESIAN_POINT('Ctrl Pts',(-5.7299307791557,-197.76175111262,-9.92453123330913));
#38535=CARTESIAN_POINT('Ctrl Pts',(-8.59489616871569,-197.58675111262,-4.96226561664425));
#38536=CARTESIAN_POINT('Ctrl Pts',(-11.4598615582757,-197.41175111262,2.06368086793017E-11));
#38537=CARTESIAN_POINT('Ctrl Pts',(-8.59489616869782,-197.23675111262,4.9622656166752));
#38538=CARTESIAN_POINT('Ctrl Pts',(-5.72993077911996,-197.06175111262,9.92453123332977));
#38539=CARTESIAN_POINT('Ctrl Pts',(1.7871392867044E-11,-196.88675111262,
9.92453123331945));
#38540=CARTESIAN_POINT('Ctrl Pts',(5.7299307791557,-196.71175111262,9.92453123330913));
#38541=CARTESIAN_POINT('Ctrl Pts',(8.59489616871569,-196.53675111262,4.96226561664425));
#38542=CARTESIAN_POINT('Ctrl Pts',(11.4598615582757,-196.36175111262,-2.06354052510241E-11));
#38543=CARTESIAN_POINT('Ctrl Pts',(8.59489616869782,-196.18675111262,-4.9622656166752));
#38544=CARTESIAN_POINT('Ctrl Pts',(5.72993077911996,-196.01175111262,-9.92453123332976));
#38545=CARTESIAN_POINT('Ctrl Pts',(-1.78726082715848E-11,-195.83675111262,
-9.92453123331945));
#38546=CARTESIAN_POINT('Ctrl Pts',(-5.7299307791557,-195.66175111262,-9.92453123330913));
#38547=CARTESIAN_POINT('Ctrl Pts',(-8.59489616871569,-195.48675111262,-4.96226561664425));
#38548=CARTESIAN_POINT('Ctrl Pts',(-11.4598615582757,-195.31175111262,2.06368086793017E-11));
#38549=CARTESIAN_POINT('Ctrl Pts',(-8.59489616869782,-195.13675111262,4.9622656166752));
#38550=CARTESIAN_POINT('Ctrl Pts',(-5.72993077911996,-194.96175111262,9.92453123332977));
#38551=CARTESIAN_POINT('Ctrl Pts',(1.7871392867044E-11,-194.78675111262,
9.92453123331945));
#38552=CARTESIAN_POINT('Ctrl Pts',(5.7299307791557,-194.61175111262,9.92453123330913));
#38553=CARTESIAN_POINT('Ctrl Pts',(8.59489616871569,-194.43675111262,4.96226561664425));
#38554=CARTESIAN_POINT('Ctrl Pts',(11.4598615582757,-194.26175111262,-2.06354052510241E-11));
#38555=CARTESIAN_POINT('Ctrl Pts',(8.59489616869782,-194.08675111262,-4.9622656166752));
#38556=CARTESIAN_POINT('Ctrl Pts',(5.72993077911996,-193.91175111262,-9.92453123332976));
#38557=CARTESIAN_POINT('Ctrl Pts',(-1.78726082715848E-11,-193.73675111262,
-9.92453123331945));
#38558=CARTESIAN_POINT('Ctrl Pts',(-5.7299307791557,-193.56175111262,-9.92453123330913));
#38559=CARTESIAN_POINT('Ctrl Pts',(-8.59489616871569,-193.38675111262,-4.96226561664425));
#38560=CARTESIAN_POINT('Ctrl Pts',(-11.4598615582757,-193.21175111262,2.06368086793017E-11));
#38561=CARTESIAN_POINT('Ctrl Pts',(-8.59489616869782,-193.03675111262,4.9622656166752));
#38562=CARTESIAN_POINT('Ctrl Pts',(-5.72993077911996,-192.86175111262,9.92453123332977));
#38563=CARTESIAN_POINT('Ctrl Pts',(1.7871392867044E-11,-192.68675111262,
9.92453123331945));
#38564=CARTESIAN_POINT('Ctrl Pts',(5.7299307791557,-192.51175111262,9.92453123330913));
#38565=CARTESIAN_POINT('Ctrl Pts',(8.59489616871569,-192.33675111262,4.96226561664425));
#38566=CARTESIAN_POINT('Ctrl Pts',(11.4598615582757,-192.16175111262,-2.06354052510241E-11));
#38567=CARTESIAN_POINT('Ctrl Pts',(8.59489616869782,-191.98675111262,-4.9622656166752));
#38568=CARTESIAN_POINT('Ctrl Pts',(5.72993077911996,-191.81175111262,-9.92453123332976));
#38569=CARTESIAN_POINT('Ctrl Pts',(-1.78726082715848E-11,-191.63675111262,
-9.92453123331945));
#38570=CARTESIAN_POINT('Ctrl Pts',(-5.7299307791557,-191.46175111262,-9.92453123330913));
#38571=CARTESIAN_POINT('Ctrl Pts',(-8.59489616871569,-191.28675111262,-4.96226561664425));
#38572=CARTESIAN_POINT('Ctrl Pts',(-11.4598615582757,-191.11175111262,2.06368086793017E-11));
#38573=CARTESIAN_POINT('Ctrl Pts',(-8.59489616869782,-190.93675111262,4.9622656166752));
#38574=CARTESIAN_POINT('Ctrl Pts',(-5.72993077911996,-190.76175111262,9.92453123332977));
#38575=CARTESIAN_POINT('Ctrl Pts',(1.7871392867044E-11,-190.58675111262,
9.92453123331945));
#38576=CARTESIAN_POINT('Ctrl Pts',(5.7299307791557,-190.41175111262,9.92453123330913));
#38577=CARTESIAN_POINT('Ctrl Pts',(8.59489616871569,-190.23675111262,4.96226561664425));
#38578=CARTESIAN_POINT('Ctrl Pts',(11.4598615582757,-190.06175111262,-2.06354052510241E-11));
#38579=CARTESIAN_POINT('Ctrl Pts',(8.59489616869782,-189.88675111262,-4.9622656166752));
#38580=CARTESIAN_POINT('Ctrl Pts',(5.72993077911996,-189.71175111262,-9.92453123332976));
#38581=CARTESIAN_POINT('Ctrl Pts',(-1.78726082715848E-11,-189.53675111262,
-9.92453123331945));
#38582=CARTESIAN_POINT('Ctrl Pts',(-5.7299307791557,-189.36175111262,-9.92453123330913));
#38583=CARTESIAN_POINT('Ctrl Pts',(-8.59489616871569,-189.18675111262,-4.96226561664425));
#38584=CARTESIAN_POINT('Ctrl Pts',(-11.4598615582757,-189.01175111262,2.06368086793017E-11));
#38585=CARTESIAN_POINT('Ctrl Pts',(-8.59489616869782,-188.83675111262,4.9622656166752));
#38586=CARTESIAN_POINT('Ctrl Pts',(-5.72993077911996,-188.66175111262,9.92453123332977));
#38587=CARTESIAN_POINT('Ctrl Pts',(1.7871392867044E-11,-188.48675111262,
9.92453123331945));
#38588=CARTESIAN_POINT('Ctrl Pts',(5.7299307791557,-188.31175111262,9.92453123330913));
#38589=CARTESIAN_POINT('Ctrl Pts',(8.59489616871569,-188.13675111262,4.96226561664425));
#38590=CARTESIAN_POINT('Ctrl Pts',(11.4598615582757,-187.96175111262,-2.06354052510241E-11));
#38591=CARTESIAN_POINT('Ctrl Pts',(8.59489616869782,-187.78675111262,-4.9622656166752));
#38592=CARTESIAN_POINT('Ctrl Pts',(5.72993077911996,-187.61175111262,-9.92453123332976));
#38593=CARTESIAN_POINT('Ctrl Pts',(-1.78726082715848E-11,-187.43675111262,
-9.92453123331945));
#38594=CARTESIAN_POINT('Ctrl Pts',(-5.7299307791557,-187.26175111262,-9.92453123330913));
#38595=CARTESIAN_POINT('Ctrl Pts',(-8.59489616871569,-187.08675111262,-4.96226561664425));
#38596=CARTESIAN_POINT('Ctrl Pts',(-11.4598615582757,-186.91175111262,2.06368086793017E-11));
#38597=CARTESIAN_POINT('Ctrl Pts',(-8.59489616869782,-186.73675111262,4.9622656166752));
#38598=CARTESIAN_POINT('Ctrl Pts',(-5.72993077911996,-186.56175111262,9.92453123332977));
#38599=CARTESIAN_POINT('Ctrl Pts',(1.7871392867044E-11,-186.38675111262,
9.92453123331945));
#38600=CARTESIAN_POINT('Ctrl Pts',(5.7299307791557,-186.21175111262,9.92453123330913));
#38601=CARTESIAN_POINT('Ctrl Pts',(8.59489616871569,-186.03675111262,4.96226561664425));
#38602=CARTESIAN_POINT('Ctrl Pts',(11.4598615582757,-185.86175111262,-2.06354052510241E-11));
#38603=CARTESIAN_POINT('Ctrl Pts',(8.59489616869782,-185.68675111262,-4.9622656166752));
#38604=CARTESIAN_POINT('Ctrl Pts',(5.72993077911996,-185.51175111262,-9.92453123332976));
#38605=CARTESIAN_POINT('Ctrl Pts',(-1.78726082715848E-11,-185.33675111262,
-9.92453123331945));
#38606=CARTESIAN_POINT('Ctrl Pts',(-5.7299307791557,-185.16175111262,-9.92453123330913));
#38607=CARTESIAN_POINT('Ctrl Pts',(-8.59489616871569,-184.98675111262,-4.96226561664425));
#38608=CARTESIAN_POINT('Ctrl Pts',(-11.4598615582757,-184.81175111262,2.06368086793017E-11));
#38609=CARTESIAN_POINT('Ctrl Pts',(-8.59489616869782,-184.63675111262,4.9622656166752));
#38610=CARTESIAN_POINT('Ctrl Pts',(-5.72993077911996,-184.46175111262,9.92453123332977));
#38611=CARTESIAN_POINT('Ctrl Pts',(1.7871392867044E-11,-184.28675111262,
9.92453123331945));
#38612=CARTESIAN_POINT('Ctrl Pts',(5.7299307791557,-184.11175111262,9.92453123330913));
#38613=CARTESIAN_POINT('Ctrl Pts',(8.59489616871569,-183.93675111262,4.96226561664425));
#38614=CARTESIAN_POINT('Ctrl Pts',(11.4598615582757,-183.76175111262,-2.06354052510241E-11));
#38615=CARTESIAN_POINT('Ctrl Pts',(8.59489616869782,-183.58675111262,-4.9622656166752));
#38616=CARTESIAN_POINT('Ctrl Pts',(5.72993077911996,-183.41175111262,-9.92453123332976));
#38617=CARTESIAN_POINT('Ctrl Pts',(-1.78726082715848E-11,-183.23675111262,
-9.92453123331945));
#38618=CARTESIAN_POINT('Ctrl Pts',(-5.7299307791557,-183.06175111262,-9.92453123330913));
#38619=CARTESIAN_POINT('Ctrl Pts',(-8.59489616871569,-182.88675111262,-4.96226561664425));
#38620=CARTESIAN_POINT('Ctrl Pts',(-11.4598615582757,-182.71175111262,2.06368086793017E-11));
#38621=CARTESIAN_POINT('Ctrl Pts',(-8.59489616869782,-182.53675111262,4.9622656166752));
#38622=CARTESIAN_POINT('Ctrl Pts',(-5.72993077911996,-182.36175111262,9.92453123332977));
#38623=CARTESIAN_POINT('Ctrl Pts',(1.7871392867044E-11,-182.18675111262,
9.92453123331945));
#38624=CARTESIAN_POINT('Ctrl Pts',(5.7299307791557,-182.01175111262,9.92453123330913));
#38625=CARTESIAN_POINT('Ctrl Pts',(8.59489616871569,-181.83675111262,4.96226561664425));
#38626=CARTESIAN_POINT('Ctrl Pts',(11.4598615582757,-181.66175111262,-2.06354052510241E-11));
#38627=CARTESIAN_POINT('Ctrl Pts',(8.59489616869782,-181.48675111262,-4.9622656166752));
#38628=CARTESIAN_POINT('Ctrl Pts',(5.72993077911996,-181.31175111262,-9.92453123332976));
#38629=CARTESIAN_POINT('Ctrl Pts',(-1.78726082715848E-11,-181.13675111262,
-9.92453123331945));
#38630=CARTESIAN_POINT('Ctrl Pts',(-5.7299307791557,-180.96175111262,-9.92453123330913));
#38631=CARTESIAN_POINT('Ctrl Pts',(-8.59489616871569,-180.78675111262,-4.96226561664425));
#38632=CARTESIAN_POINT('Ctrl Pts',(-11.4598615582757,-180.61175111262,2.06368086793017E-11));
#38633=CARTESIAN_POINT('Ctrl Pts',(-8.59489616869782,-180.43675111262,4.9622656166752));
#38634=CARTESIAN_POINT('Ctrl Pts',(-5.72993077911996,-180.26175111262,9.92453123332977));
#38635=CARTESIAN_POINT('Ctrl Pts',(1.7871392867044E-11,-180.08675111262,
9.92453123331945));
#38636=CARTESIAN_POINT('Ctrl Pts',(5.7299307791557,-179.91175111262,9.92453123330913));
#38637=CARTESIAN_POINT('Ctrl Pts',(8.59489616871569,-179.73675111262,4.96226561664425));
#38638=CARTESIAN_POINT('Ctrl Pts',(11.4598615582757,-179.56175111262,-2.06354052510241E-11));
#38639=CARTESIAN_POINT('Ctrl Pts',(8.59489616869782,-179.38675111262,-4.9622656166752));
#38640=CARTESIAN_POINT('Ctrl Pts',(5.72993077911996,-179.21175111262,-9.92453123332976));
#38641=CARTESIAN_POINT('Ctrl Pts',(-1.78726082715848E-11,-179.03675111262,
-9.92453123331945));
#38642=CARTESIAN_POINT('Ctrl Pts',(-5.7299307791557,-178.86175111262,-9.92453123330913));
#38643=CARTESIAN_POINT('Ctrl Pts',(-8.59489616871569,-178.68675111262,-4.96226561664425));
#38644=CARTESIAN_POINT('Ctrl Pts',(-11.4598615582757,-178.51175111262,2.06368086793017E-11));
#38645=CARTESIAN_POINT('Ctrl Pts',(-8.59489616869782,-178.33675111262,4.9622656166752));
#38646=CARTESIAN_POINT('Ctrl Pts',(-5.72993077911996,-178.16175111262,9.92453123332977));
#38647=CARTESIAN_POINT('Ctrl Pts',(1.7871392867044E-11,-177.98675111262,
9.92453123331945));
#38648=CARTESIAN_POINT('Ctrl Pts',(5.7299307791557,-177.81175111262,9.92453123330913));
#38649=CARTESIAN_POINT('Ctrl Pts',(8.59489616871569,-177.63675111262,4.96226561664425));
#38650=CARTESIAN_POINT('Ctrl Pts',(11.4598615582757,-177.46175111262,-2.06354052510241E-11));
#38651=CARTESIAN_POINT('Ctrl Pts',(8.59489616869782,-177.28675111262,-4.9622656166752));
#38652=CARTESIAN_POINT('Ctrl Pts',(5.72993077911996,-177.11175111262,-9.92453123332976));
#38653=CARTESIAN_POINT('Ctrl Pts',(-1.78726082715848E-11,-176.93675111262,
-9.92453123331945));
#38654=CARTESIAN_POINT('Ctrl Pts',(-5.7299307791557,-176.76175111262,-9.92453123330913));
#38655=CARTESIAN_POINT('Ctrl Pts',(-8.59489616871569,-176.58675111262,-4.96226561664425));
#38656=CARTESIAN_POINT('Ctrl Pts',(-11.4598615582757,-176.41175111262,2.06368086793017E-11));
#38657=CARTESIAN_POINT('Ctrl Pts',(-8.59489616869782,-176.23675111262,4.9622656166752));
#38658=CARTESIAN_POINT('Ctrl Pts',(-5.72993077911996,-176.06175111262,9.92453123332977));
#38659=CARTESIAN_POINT('Ctrl Pts',(1.7871392867044E-11,-175.88675111262,
9.92453123331945));
#38660=CARTESIAN_POINT('Ctrl Pts',(5.7299307791557,-175.71175111262,9.92453123330913));
#38661=CARTESIAN_POINT('Ctrl Pts',(8.59489616871569,-175.53675111262,4.96226561664425));
#38662=CARTESIAN_POINT('Ctrl Pts',(11.4598615582757,-175.36175111262,-2.06354052510241E-11));
#38663=CARTESIAN_POINT('Ctrl Pts',(8.59489616869782,-175.18675111262,-4.9622656166752));
#38664=CARTESIAN_POINT('Ctrl Pts',(5.72993077911996,-175.01175111262,-9.92453123332976));
#38665=CARTESIAN_POINT('Ctrl Pts',(-1.78726082715848E-11,-174.83675111262,
-9.92453123331945));
#38666=CARTESIAN_POINT('Ctrl Pts',(-5.7299307791557,-174.66175111262,-9.92453123330913));
#38667=CARTESIAN_POINT('Ctrl Pts',(-8.59489616871569,-174.48675111262,-4.96226561664425));
#38668=CARTESIAN_POINT('Ctrl Pts',(-11.4598615582757,-174.31175111262,2.06368086793017E-11));
#38669=CARTESIAN_POINT('Ctrl Pts',(-8.59489616869782,-174.13675111262,4.9622656166752));
#38670=CARTESIAN_POINT('Ctrl Pts',(-5.72993077911996,-173.96175111262,9.92453123332977));
#38671=CARTESIAN_POINT('Ctrl Pts',(1.7871392867044E-11,-173.78675111262,
9.92453123331945));
#38672=CARTESIAN_POINT('Ctrl Pts',(5.7299307791557,-173.61175111262,9.92453123330913));
#38673=CARTESIAN_POINT('Ctrl Pts',(8.59489616871569,-173.43675111262,4.96226561664425));
#38674=CARTESIAN_POINT('Ctrl Pts',(11.4598615582757,-173.26175111262,-2.06354052510241E-11));
#38675=CARTESIAN_POINT('Ctrl Pts',(8.59489616869782,-173.08675111262,-4.9622656166752));
#38676=CARTESIAN_POINT('Ctrl Pts',(5.72993077911996,-172.91175111262,-9.92453123332976));
#38677=CARTESIAN_POINT('Ctrl Pts',(-1.78726082715848E-11,-172.73675111262,
-9.92453123331945));
#38678=CARTESIAN_POINT('Ctrl Pts',(-5.7299307791557,-172.56175111262,-9.92453123330913));
#38679=CARTESIAN_POINT('Ctrl Pts',(-8.59489616871569,-172.38675111262,-4.96226561664425));
#38680=CARTESIAN_POINT('Ctrl Pts',(-11.4598615582757,-172.21175111262,2.06368086793017E-11));
#38681=CARTESIAN_POINT('Ctrl Pts',(-8.59489616869782,-172.03675111262,4.9622656166752));
#38682=CARTESIAN_POINT('Ctrl Pts',(-5.72993077911996,-171.86175111262,9.92453123332977));
#38683=CARTESIAN_POINT('Ctrl Pts',(1.7871392867044E-11,-171.68675111262,
9.92453123331945));
#38684=CARTESIAN_POINT('Ctrl Pts',(5.7299307791557,-171.51175111262,9.92453123330913));
#38685=CARTESIAN_POINT('Ctrl Pts',(8.59489616871569,-171.33675111262,4.96226561664425));
#38686=CARTESIAN_POINT('Ctrl Pts',(11.4598615582757,-171.16175111262,-2.06354052510241E-11));
#38687=CARTESIAN_POINT('Ctrl Pts',(8.59489616869782,-170.98675111262,-4.9622656166752));
#38688=CARTESIAN_POINT('Ctrl Pts',(5.72993077911996,-170.81175111262,-9.92453123332976));
#38689=CARTESIAN_POINT('Ctrl Pts',(-1.78726082715848E-11,-170.63675111262,
-9.92453123331945));
#38690=CARTESIAN_POINT('Ctrl Pts',(-5.7299307791557,-170.46175111262,-9.92453123330913));
#38691=CARTESIAN_POINT('Ctrl Pts',(-8.59489616871569,-170.28675111262,-4.96226561664425));
#38692=CARTESIAN_POINT('Ctrl Pts',(-11.4598615582757,-170.11175111262,2.06368086793017E-11));
#38693=CARTESIAN_POINT('Ctrl Pts',(-8.59489616869782,-169.93675111262,4.9622656166752));
#38694=CARTESIAN_POINT('Ctrl Pts',(-5.72993077911996,-169.76175111262,9.92453123332977));
#38695=CARTESIAN_POINT('Ctrl Pts',(1.7871392867044E-11,-169.58675111262,
9.92453123331945));
#38696=CARTESIAN_POINT('Ctrl Pts',(5.7299307791557,-169.41175111262,9.92453123330913));
#38697=CARTESIAN_POINT('Ctrl Pts',(8.59489616871569,-169.23675111262,4.96226561664425));
#38698=CARTESIAN_POINT('Ctrl Pts',(11.4598615582757,-169.06175111262,-2.06354052510241E-11));
#38699=CARTESIAN_POINT('Ctrl Pts',(8.59489616869782,-168.88675111262,-4.9622656166752));
#38700=CARTESIAN_POINT('Ctrl Pts',(5.72993077911996,-168.71175111262,-9.92453123332976));
#38701=CARTESIAN_POINT('Ctrl Pts',(-1.78726082715848E-11,-168.53675111262,
-9.92453123331945));
#38702=CARTESIAN_POINT('Ctrl Pts',(-5.7299307791557,-168.36175111262,-9.92453123330913));
#38703=CARTESIAN_POINT('Ctrl Pts',(-8.59489616871569,-168.18675111262,-4.96226561664425));
#38704=CARTESIAN_POINT('Ctrl Pts',(-11.4598615582757,-168.01175111262,2.06368086793017E-11));
#38705=CARTESIAN_POINT('Ctrl Pts',(-8.59489616869782,-167.83675111262,4.9622656166752));
#38706=CARTESIAN_POINT('Ctrl Pts',(-5.72993077911996,-167.66175111262,9.92453123332977));
#38707=CARTESIAN_POINT('Ctrl Pts',(1.7871392867044E-11,-167.48675111262,
9.92453123331945));
#38708=CARTESIAN_POINT('Ctrl Pts',(5.7299307791557,-167.31175111262,9.92453123330913));
#38709=CARTESIAN_POINT('Ctrl Pts',(8.59489616871569,-167.13675111262,4.96226561664425));
#38710=CARTESIAN_POINT('Ctrl Pts',(11.4598615582757,-166.96175111262,-2.06354052510241E-11));
#38711=CARTESIAN_POINT('Ctrl Pts',(8.59489616869782,-166.78675111262,-4.9622656166752));
#38712=CARTESIAN_POINT('Ctrl Pts',(5.72993077911996,-166.61175111262,-9.92453123332976));
#38713=CARTESIAN_POINT('Ctrl Pts',(-1.78726082715848E-11,-166.43675111262,
-9.92453123331945));
#38714=CARTESIAN_POINT('Ctrl Pts',(-5.7299307791557,-166.26175111262,-9.92453123330913));
#38715=CARTESIAN_POINT('Ctrl Pts',(-8.59489616871569,-166.08675111262,-4.96226561664425));
#38716=CARTESIAN_POINT('Ctrl Pts',(-11.4598615582757,-165.91175111262,2.06368086793017E-11));
#38717=CARTESIAN_POINT('Ctrl Pts',(-8.59489616869782,-165.73675111262,4.9622656166752));
#38718=CARTESIAN_POINT('Ctrl Pts',(-5.72993077911996,-165.56175111262,9.92453123332977));
#38719=CARTESIAN_POINT('Ctrl Pts',(1.7871392867044E-11,-165.38675111262,
9.92453123331945));
#38720=CARTESIAN_POINT('Ctrl Pts',(5.7299307791557,-165.21175111262,9.92453123330913));
#38721=CARTESIAN_POINT('Ctrl Pts',(8.59489616871569,-165.03675111262,4.96226561664425));
#38722=CARTESIAN_POINT('Ctrl Pts',(11.4598615582757,-164.86175111262,-2.06354052510241E-11));
#38723=CARTESIAN_POINT('Ctrl Pts',(8.59489616869782,-164.68675111262,-4.9622656166752));
#38724=CARTESIAN_POINT('Ctrl Pts',(5.72993077911996,-164.51175111262,-9.92453123332976));
#38725=CARTESIAN_POINT('Ctrl Pts',(-1.78726082715848E-11,-164.33675111262,
-9.92453123331945));
#38726=CARTESIAN_POINT('Ctrl Pts',(-5.7299307791557,-164.16175111262,-9.92453123330913));
#38727=CARTESIAN_POINT('Ctrl Pts',(-8.59489616871569,-163.98675111262,-4.96226561664425));
#38728=CARTESIAN_POINT('Ctrl Pts',(-11.4598615582757,-163.81175111262,2.06368086793017E-11));
#38729=CARTESIAN_POINT('Ctrl Pts',(-8.59489616869782,-163.63675111262,4.9622656166752));
#38730=CARTESIAN_POINT('Ctrl Pts',(-5.72993077911996,-163.46175111262,9.92453123332977));
#38731=CARTESIAN_POINT('Ctrl Pts',(1.7871392867044E-11,-163.28675111262,
9.92453123331945));
#38732=CARTESIAN_POINT('Ctrl Pts',(5.7299307791557,-163.11175111262,9.92453123330913));
#38733=CARTESIAN_POINT('Ctrl Pts',(8.59489616871569,-162.93675111262,4.96226561664425));
#38734=CARTESIAN_POINT('Ctrl Pts',(11.4598615582757,-162.76175111262,-2.06354052510241E-11));
#38735=CARTESIAN_POINT('Ctrl Pts',(8.59489616869782,-162.58675111262,-4.9622656166752));
#38736=CARTESIAN_POINT('Ctrl Pts',(5.72993077911996,-162.41175111262,-9.92453123332976));
#38737=CARTESIAN_POINT('Ctrl Pts',(-1.78726082715848E-11,-162.23675111262,
-9.92453123331945));
#38738=CARTESIAN_POINT('Ctrl Pts',(-5.7299307791557,-162.06175111262,-9.92453123330913));
#38739=CARTESIAN_POINT('Ctrl Pts',(-8.59489616871569,-161.88675111262,-4.96226561664425));
#38740=CARTESIAN_POINT('Ctrl Pts',(-11.4598615582757,-161.71175111262,2.06368086793017E-11));
#38741=CARTESIAN_POINT('Ctrl Pts',(-8.59489616869782,-161.53675111262,4.9622656166752));
#38742=CARTESIAN_POINT('Ctrl Pts',(-5.72993077911996,-161.36175111262,9.92453123332977));
#38743=CARTESIAN_POINT('Ctrl Pts',(1.7871392867044E-11,-161.18675111262,
9.92453123331945));
#38744=CARTESIAN_POINT('Ctrl Pts',(5.7299307791557,-161.01175111262,9.92453123330913));
#38745=CARTESIAN_POINT('Ctrl Pts',(8.59489616871569,-160.83675111262,4.96226561664425));
#38746=CARTESIAN_POINT('Ctrl Pts',(11.4598615582757,-160.66175111262,-2.06354052510241E-11));
#38747=CARTESIAN_POINT('Ctrl Pts',(8.59489616869782,-160.48675111262,-4.9622656166752));
#38748=CARTESIAN_POINT('Ctrl Pts',(5.72993077911996,-160.31175111262,-9.92453123332976));
#38749=CARTESIAN_POINT('Ctrl Pts',(-1.78726082715848E-11,-160.13675111262,
-9.92453123331945));
#38750=CARTESIAN_POINT('Ctrl Pts',(-5.7299307791557,-159.96175111262,-9.92453123330913));
#38751=CARTESIAN_POINT('Ctrl Pts',(-8.59489616871569,-159.78675111262,-4.96226561664425));
#38752=CARTESIAN_POINT('Ctrl Pts',(-11.4598615582757,-159.61175111262,2.06368086793017E-11));
#38753=CARTESIAN_POINT('Ctrl Pts',(-8.59489616869782,-159.43675111262,4.9622656166752));
#38754=CARTESIAN_POINT('Ctrl Pts',(-5.72993077911996,-159.26175111262,9.92453123332977));
#38755=CARTESIAN_POINT('Ctrl Pts',(1.7871392867044E-11,-159.08675111262,
9.92453123331945));
#38756=CARTESIAN_POINT('Ctrl Pts',(5.7299307791557,-158.91175111262,9.92453123330913));
#38757=CARTESIAN_POINT('Ctrl Pts',(8.59489616871569,-158.73675111262,4.96226561664425));
#38758=CARTESIAN_POINT('Ctrl Pts',(11.4598615582757,-158.56175111262,-2.06354052510241E-11));
#38759=CARTESIAN_POINT('Ctrl Pts',(8.59489616869782,-158.38675111262,-4.9622656166752));
#38760=CARTESIAN_POINT('Ctrl Pts',(5.72993077911996,-158.21175111262,-9.92453123332976));
#38761=CARTESIAN_POINT('Ctrl Pts',(-1.78726082715848E-11,-158.03675111262,
-9.92453123331945));
#38762=CARTESIAN_POINT('Ctrl Pts',(-5.7299307791557,-157.86175111262,-9.92453123330913));
#38763=CARTESIAN_POINT('Ctrl Pts',(-8.59489616871569,-157.68675111262,-4.96226561664425));
#38764=CARTESIAN_POINT('Ctrl Pts',(-11.4598615582757,-157.51175111262,2.06368086793017E-11));
#38765=CARTESIAN_POINT('Ctrl Pts',(-8.59489616869782,-157.33675111262,4.9622656166752));
#38766=CARTESIAN_POINT('Ctrl Pts',(-5.72993077911996,-157.16175111262,9.92453123332977));
#38767=CARTESIAN_POINT('Ctrl Pts',(1.7871392867044E-11,-156.98675111262,
9.92453123331945));
#38768=CARTESIAN_POINT('Ctrl Pts',(5.7299307791557,-156.81175111262,9.92453123330913));
#38769=CARTESIAN_POINT('Ctrl Pts',(8.59489616871569,-156.63675111262,4.96226561664425));
#38770=CARTESIAN_POINT('Ctrl Pts',(11.4598615582757,-156.46175111262,-2.06354052510241E-11));
#38771=CARTESIAN_POINT('Ctrl Pts',(8.59489616869782,-156.28675111262,-4.9622656166752));
#38772=CARTESIAN_POINT('Ctrl Pts',(5.72993077911996,-156.11175111262,-9.92453123332976));
#38773=CARTESIAN_POINT('Ctrl Pts',(-1.78726082715848E-11,-155.93675111262,
-9.92453123331945));
#38774=CARTESIAN_POINT('Ctrl Pts',(-5.7299307791557,-155.76175111262,-9.92453123330913));
#38775=CARTESIAN_POINT('Ctrl Pts',(-8.59489616871569,-155.58675111262,-4.96226561664425));
#38776=CARTESIAN_POINT('Ctrl Pts',(-11.4598615582757,-155.41175111262,2.06368086793017E-11));
#38777=CARTESIAN_POINT('Ctrl Pts',(-8.59489616869782,-155.23675111262,4.9622656166752));
#38778=CARTESIAN_POINT('Ctrl Pts',(-5.72993077911996,-155.06175111262,9.92453123332977));
#38779=CARTESIAN_POINT('Ctrl Pts',(1.7871392867044E-11,-154.88675111262,
9.92453123331945));
#38780=CARTESIAN_POINT('Ctrl Pts',(5.7299307791557,-154.71175111262,9.92453123330913));
#38781=CARTESIAN_POINT('Ctrl Pts',(8.59489616871569,-154.53675111262,4.96226561664425));
#38782=CARTESIAN_POINT('Ctrl Pts',(11.4598615582757,-154.36175111262,-2.06354052510241E-11));
#38783=CARTESIAN_POINT('Ctrl Pts',(8.59489616869782,-154.18675111262,-4.9622656166752));
#38784=CARTESIAN_POINT('Ctrl Pts',(5.72993077911996,-154.01175111262,-9.92453123332976));
#38785=CARTESIAN_POINT('Ctrl Pts',(-1.78726082715848E-11,-153.83675111262,
-9.92453123331945));
#38786=CARTESIAN_POINT('Ctrl Pts',(-5.7299307791557,-153.66175111262,-9.92453123330913));
#38787=CARTESIAN_POINT('Ctrl Pts',(-8.59489616871569,-153.48675111262,-4.96226561664425));
#38788=CARTESIAN_POINT('Ctrl Pts',(-11.4598615582757,-153.31175111262,2.06368086793017E-11));
#38789=CARTESIAN_POINT('Ctrl Pts',(-8.59489616869782,-153.13675111262,4.9622656166752));
#38790=CARTESIAN_POINT('Ctrl Pts',(-5.72993077911996,-152.96175111262,9.92453123332977));
#38791=CARTESIAN_POINT('Ctrl Pts',(1.7871392867044E-11,-152.78675111262,
9.92453123331945));
#38792=CARTESIAN_POINT('Ctrl Pts',(5.7299307791557,-152.61175111262,9.92453123330913));
#38793=CARTESIAN_POINT('Ctrl Pts',(8.59489616871569,-152.43675111262,4.96226561664425));
#38794=CARTESIAN_POINT('Ctrl Pts',(11.4598615582757,-152.26175111262,-2.06354052510241E-11));
#38795=CARTESIAN_POINT('Ctrl Pts',(8.59489616869782,-152.08675111262,-4.9622656166752));
#38796=CARTESIAN_POINT('Ctrl Pts',(5.72993077911996,-151.91175111262,-9.92453123332976));
#38797=CARTESIAN_POINT('Ctrl Pts',(-1.78726082715848E-11,-151.73675111262,
-9.92453123331945));
#38798=CARTESIAN_POINT('Ctrl Pts',(-5.7299307791557,-151.56175111262,-9.92453123330913));
#38799=CARTESIAN_POINT('Ctrl Pts',(-8.59489616871569,-151.38675111262,-4.96226561664425));
#38800=CARTESIAN_POINT('Ctrl Pts',(-11.4598615582757,-151.21175111262,2.06368086793017E-11));
#38801=CARTESIAN_POINT('Ctrl Pts',(-8.59489616869782,-151.03675111262,4.9622656166752));
#38802=CARTESIAN_POINT('Ctrl Pts',(-5.72993077911996,-150.86175111262,9.92453123332977));
#38803=CARTESIAN_POINT('Ctrl Pts',(1.7871392867044E-11,-150.68675111262,
9.92453123331945));
#38804=CARTESIAN_POINT('Ctrl Pts',(5.7299307791557,-150.51175111262,9.92453123330913));
#38805=CARTESIAN_POINT('Ctrl Pts',(8.59489616871569,-150.33675111262,4.96226561664425));
#38806=CARTESIAN_POINT('Ctrl Pts',(11.4598615582757,-150.16175111262,-2.06354052510241E-11));
#38807=CARTESIAN_POINT('Ctrl Pts',(8.59489616869782,-149.98675111262,-4.9622656166752));
#38808=CARTESIAN_POINT('Ctrl Pts',(5.72993077911996,-149.81175111262,-9.92453123332976));
#38809=CARTESIAN_POINT('Ctrl Pts',(-1.78726082715848E-11,-149.63675111262,
-9.92453123331945));
#38810=CARTESIAN_POINT('Ctrl Pts',(-5.7299307791557,-149.46175111262,-9.92453123330913));
#38811=CARTESIAN_POINT('Ctrl Pts',(-8.59489616871569,-149.28675111262,-4.96226561664425));
#38812=CARTESIAN_POINT('Ctrl Pts',(-11.4598615582757,-149.11175111262,2.06368086793017E-11));
#38813=CARTESIAN_POINT('Ctrl Pts',(-8.59489616869782,-148.93675111262,4.9622656166752));
#38814=CARTESIAN_POINT('Ctrl Pts',(-5.72993077911996,-148.76175111262,9.92453123332977));
#38815=CARTESIAN_POINT('Ctrl Pts',(1.7871392867044E-11,-148.58675111262,
9.92453123331945));
#38816=CARTESIAN_POINT('Ctrl Pts',(5.7299307791557,-148.41175111262,9.92453123330913));
#38817=CARTESIAN_POINT('Ctrl Pts',(8.59489616871569,-148.23675111262,4.96226561664425));
#38818=CARTESIAN_POINT('Ctrl Pts',(11.4598615582757,-148.06175111262,-2.06354052510241E-11));
#38819=CARTESIAN_POINT('Ctrl Pts',(8.59489616869782,-147.88675111262,-4.9622656166752));
#38820=CARTESIAN_POINT('Ctrl Pts',(5.72993077911996,-147.71175111262,-9.92453123332976));
#38821=CARTESIAN_POINT('Ctrl Pts',(-1.78726082715848E-11,-147.53675111262,
-9.92453123331945));
#38822=CARTESIAN_POINT('Ctrl Pts',(-5.7299307791557,-147.36175111262,-9.92453123330913));
#38823=CARTESIAN_POINT('Ctrl Pts',(-8.59489616871569,-147.18675111262,-4.96226561664425));
#38824=CARTESIAN_POINT('Ctrl Pts',(-11.4598615582757,-147.01175111262,2.06368086793017E-11));
#38825=CARTESIAN_POINT('Ctrl Pts',(-8.59489616869782,-146.83675111262,4.9622656166752));
#38826=CARTESIAN_POINT('Ctrl Pts',(-5.72993077911996,-146.66175111262,9.92453123332977));
#38827=CARTESIAN_POINT('Ctrl Pts',(1.7871392867044E-11,-146.48675111262,
9.92453123331945));
#38828=CARTESIAN_POINT('Ctrl Pts',(5.7299307791557,-146.31175111262,9.92453123330913));
#38829=CARTESIAN_POINT('Ctrl Pts',(8.59489616871569,-146.13675111262,4.96226561664425));
#38830=CARTESIAN_POINT('Ctrl Pts',(11.4598615582757,-145.96175111262,-2.06354052510241E-11));
#38831=CARTESIAN_POINT('Ctrl Pts',(8.59489616869782,-145.78675111262,-4.9622656166752));
#38832=CARTESIAN_POINT('Ctrl Pts',(5.72993077911996,-145.61175111262,-9.92453123332976));
#38833=CARTESIAN_POINT('Ctrl Pts',(-1.78726082715848E-11,-145.43675111262,
-9.92453123331945));
#38834=CARTESIAN_POINT('Ctrl Pts',(-5.7299307791557,-145.26175111262,-9.92453123330913));
#38835=CARTESIAN_POINT('Ctrl Pts',(-8.59489616871569,-145.08675111262,-4.96226561664425));
#38836=CARTESIAN_POINT('Ctrl Pts',(-11.4598615582757,-144.91175111262,2.06368086793017E-11));
#38837=CARTESIAN_POINT('Ctrl Pts',(-8.59489616869782,-144.73675111262,4.9622656166752));
#38838=CARTESIAN_POINT('Ctrl Pts',(-5.72993077911996,-144.56175111262,9.92453123332977));
#38839=CARTESIAN_POINT('Ctrl Pts',(1.7871392867044E-11,-144.38675111262,
9.92453123331945));
#38840=CARTESIAN_POINT('Ctrl Pts',(5.7299307791557,-144.21175111262,9.92453123330913));
#38841=CARTESIAN_POINT('Ctrl Pts',(8.59489616871569,-144.03675111262,4.96226561664425));
#38842=CARTESIAN_POINT('Ctrl Pts',(11.4598615582757,-143.86175111262,-2.06354052510241E-11));
#38843=CARTESIAN_POINT('Ctrl Pts',(8.59489616869782,-143.68675111262,-4.9622656166752));
#38844=CARTESIAN_POINT('Ctrl Pts',(5.72993077911996,-143.51175111262,-9.92453123332976));
#38845=CARTESIAN_POINT('Ctrl Pts',(-1.78726082715848E-11,-143.33675111262,
-9.92453123331945));
#38846=CARTESIAN_POINT('Ctrl Pts',(-5.7299307791557,-143.16175111262,-9.92453123330913));
#38847=CARTESIAN_POINT('Ctrl Pts',(-8.59489616871569,-142.98675111262,-4.96226561664425));
#38848=CARTESIAN_POINT('Ctrl Pts',(-11.4598615582757,-142.81175111262,2.06368086793017E-11));
#38849=CARTESIAN_POINT('Ctrl Pts',(-8.59489616869782,-142.63675111262,4.9622656166752));
#38850=CARTESIAN_POINT('Ctrl Pts',(-5.72993077911996,-142.46175111262,9.92453123332977));
#38851=CARTESIAN_POINT('Ctrl Pts',(1.7871392867044E-11,-142.28675111262,
9.92453123331945));
#38852=CARTESIAN_POINT('Ctrl Pts',(5.7299307791557,-142.11175111262,9.92453123330913));
#38853=CARTESIAN_POINT('Ctrl Pts',(8.59489616871569,-141.93675111262,4.96226561664425));
#38854=CARTESIAN_POINT('Ctrl Pts',(11.4598615582757,-141.76175111262,-2.06354052510241E-11));
#38855=CARTESIAN_POINT('Ctrl Pts',(8.59489616869782,-141.58675111262,-4.9622656166752));
#38856=CARTESIAN_POINT('Ctrl Pts',(5.72993077911996,-141.41175111262,-9.92453123332976));
#38857=CARTESIAN_POINT('Ctrl Pts',(-1.78726082715848E-11,-141.23675111262,
-9.92453123331945));
#38858=CARTESIAN_POINT('Ctrl Pts',(-5.7299307791557,-141.06175111262,-9.92453123330913));
#38859=CARTESIAN_POINT('Ctrl Pts',(-8.59489616871569,-140.88675111262,-4.96226561664425));
#38860=CARTESIAN_POINT('Ctrl Pts',(-11.4598615582757,-140.71175111262,2.06368086793017E-11));
#38861=CARTESIAN_POINT('Ctrl Pts',(-8.59489616869782,-140.53675111262,4.9622656166752));
#38862=CARTESIAN_POINT('Ctrl Pts',(-5.72993077911996,-140.36175111262,9.92453123332977));
#38863=CARTESIAN_POINT('Ctrl Pts',(1.7871392867044E-11,-140.18675111262,
9.92453123331945));
#38864=CARTESIAN_POINT('Ctrl Pts',(5.7299307791557,-140.01175111262,9.92453123330913));
#38865=CARTESIAN_POINT('Ctrl Pts',(8.59489616871569,-139.83675111262,4.96226561664425));
#38866=CARTESIAN_POINT('Ctrl Pts',(11.4598615582757,-139.66175111262,-2.06354052510241E-11));
#38867=CARTESIAN_POINT('Ctrl Pts',(8.59489616869782,-139.48675111262,-4.9622656166752));
#38868=CARTESIAN_POINT('Ctrl Pts',(5.72993077911996,-139.31175111262,-9.92453123332976));
#38869=CARTESIAN_POINT('Ctrl Pts',(-1.78726082715848E-11,-139.13675111262,
-9.92453123331945));
#38870=CARTESIAN_POINT('Ctrl Pts',(-5.7299307791557,-138.96175111262,-9.92453123330913));
#38871=CARTESIAN_POINT('Ctrl Pts',(-8.59489616871569,-138.78675111262,-4.96226561664425));
#38872=CARTESIAN_POINT('Ctrl Pts',(-11.4598615582757,-138.61175111262,2.06368086793017E-11));
#38873=CARTESIAN_POINT('Ctrl Pts',(-8.59489616869782,-138.43675111262,4.9622656166752));
#38874=CARTESIAN_POINT('Ctrl Pts',(-5.72993077911996,-138.26175111262,9.92453123332977));
#38875=CARTESIAN_POINT('Ctrl Pts',(1.7871392867044E-11,-138.08675111262,
9.92453123331945));
#38876=CARTESIAN_POINT('Ctrl Pts',(5.7299307791557,-137.91175111262,9.92453123330913));
#38877=CARTESIAN_POINT('Ctrl Pts',(8.59489616871569,-137.73675111262,4.96226561664425));
#38878=CARTESIAN_POINT('Ctrl Pts',(11.4598615582757,-137.56175111262,-2.06354052510241E-11));
#38879=CARTESIAN_POINT('Ctrl Pts',(8.59489616869782,-137.38675111262,-4.9622656166752));
#38880=CARTESIAN_POINT('Ctrl Pts',(5.72993077911996,-137.21175111262,-9.92453123332976));
#38881=CARTESIAN_POINT('Ctrl Pts',(-1.78726082715848E-11,-137.03675111262,
-9.92453123331945));
#38882=CARTESIAN_POINT('Ctrl Pts',(-5.7299307791557,-136.86175111262,-9.92453123330913));
#38883=CARTESIAN_POINT('Ctrl Pts',(-8.59489616871569,-136.68675111262,-4.96226561664425));
#38884=CARTESIAN_POINT('Ctrl Pts',(-11.4598615582757,-136.51175111262,2.06368086793017E-11));
#38885=CARTESIAN_POINT('Ctrl Pts',(-8.59489616869782,-136.33675111262,4.9622656166752));
#38886=CARTESIAN_POINT('Ctrl Pts',(-5.72993077911996,-136.16175111262,9.92453123332977));
#38887=CARTESIAN_POINT('Ctrl Pts',(1.7871392867044E-11,-135.98675111262,
9.92453123331945));
#38888=CARTESIAN_POINT('Ctrl Pts',(5.7299307791557,-135.81175111262,9.92453123330913));
#38889=CARTESIAN_POINT('Ctrl Pts',(8.59489616871569,-135.63675111262,4.96226561664425));
#38890=CARTESIAN_POINT('Ctrl Pts',(11.4598615582757,-135.46175111262,-2.06354052510241E-11));
#38891=CARTESIAN_POINT('Ctrl Pts',(8.59489616869782,-135.28675111262,-4.9622656166752));
#38892=CARTESIAN_POINT('Ctrl Pts',(5.72993077911996,-135.11175111262,-9.92453123332976));
#38893=CARTESIAN_POINT('Ctrl Pts',(-1.78726082715848E-11,-134.93675111262,
-9.92453123331945));
#38894=CARTESIAN_POINT('Ctrl Pts',(-5.7299307791557,-134.76175111262,-9.92453123330913));
#38895=CARTESIAN_POINT('Ctrl Pts',(-8.59489616871569,-134.58675111262,-4.96226561664425));
#38896=CARTESIAN_POINT('Ctrl Pts',(-11.4598615582757,-134.41175111262,2.06368086793017E-11));
#38897=CARTESIAN_POINT('Ctrl Pts',(-8.59489616869782,-134.23675111262,4.9622656166752));
#38898=CARTESIAN_POINT('Ctrl Pts',(-5.72993077911996,-134.06175111262,9.92453123332977));
#38899=CARTESIAN_POINT('Ctrl Pts',(1.7871392867044E-11,-133.88675111262,
9.92453123331945));
#38900=CARTESIAN_POINT('Ctrl Pts',(5.7299307791557,-133.71175111262,9.92453123330913));
#38901=CARTESIAN_POINT('Ctrl Pts',(8.59489616871569,-133.53675111262,4.96226561664425));
#38902=CARTESIAN_POINT('Ctrl Pts',(11.4598615582757,-133.36175111262,-2.06354052510241E-11));
#38903=CARTESIAN_POINT('Ctrl Pts',(8.59489616869782,-133.18675111262,-4.9622656166752));
#38904=CARTESIAN_POINT('Ctrl Pts',(5.72993077911996,-133.01175111262,-9.92453123332976));
#38905=CARTESIAN_POINT('Ctrl Pts',(-1.78726082715848E-11,-132.83675111262,
-9.92453123331945));
#38906=CARTESIAN_POINT('Ctrl Pts',(-5.7299307791557,-132.66175111262,-9.92453123330913));
#38907=CARTESIAN_POINT('Ctrl Pts',(-8.59489616871569,-132.48675111262,-4.96226561664425));
#38908=CARTESIAN_POINT('Ctrl Pts',(-11.4598615582757,-132.31175111262,2.06368086793017E-11));
#38909=CARTESIAN_POINT('Ctrl Pts',(-8.59489616869782,-132.13675111262,4.9622656166752));
#38910=CARTESIAN_POINT('Ctrl Pts',(-5.72993077911996,-131.96175111262,9.92453123332977));
#38911=CARTESIAN_POINT('Ctrl Pts',(1.7871392867044E-11,-131.78675111262,
9.92453123331945));
#38912=CARTESIAN_POINT('Ctrl Pts',(5.7299307791557,-131.61175111262,9.92453123330913));
#38913=CARTESIAN_POINT('Ctrl Pts',(8.59489616871569,-131.43675111262,4.96226561664425));
#38914=CARTESIAN_POINT('Ctrl Pts',(11.4598615582757,-131.26175111262,-2.06354052510241E-11));
#38915=CARTESIAN_POINT('Ctrl Pts',(8.59489616869782,-131.08675111262,-4.9622656166752));
#38916=CARTESIAN_POINT('Ctrl Pts',(5.72993077911996,-130.91175111262,-9.92453123332976));
#38917=CARTESIAN_POINT('Ctrl Pts',(-1.78726082715848E-11,-130.73675111262,
-9.92453123331945));
#38918=CARTESIAN_POINT('Ctrl Pts',(-5.7299307791557,-130.56175111262,-9.92453123330913));
#38919=CARTESIAN_POINT('Ctrl Pts',(-8.59489616871569,-130.38675111262,-4.96226561664425));
#38920=CARTESIAN_POINT('Ctrl Pts',(-11.4598615582757,-130.21175111262,2.06368086793017E-11));
#38921=CARTESIAN_POINT('Ctrl Pts',(-8.59489616869782,-130.03675111262,4.9622656166752));
#38922=CARTESIAN_POINT('Ctrl Pts',(-5.72993077911996,-129.86175111262,9.92453123332977));
#38923=CARTESIAN_POINT('Ctrl Pts',(1.7871392867044E-11,-129.68675111262,
9.92453123331945));
#38924=CARTESIAN_POINT('Ctrl Pts',(5.7299307791557,-129.51175111262,9.92453123330913));
#38925=CARTESIAN_POINT('Ctrl Pts',(8.59489616871569,-129.33675111262,4.96226561664425));
#38926=CARTESIAN_POINT('Ctrl Pts',(11.4598615582757,-129.16175111262,-2.06354052510241E-11));
#38927=CARTESIAN_POINT('Ctrl Pts',(8.59489616869782,-128.98675111262,-4.9622656166752));
#38928=CARTESIAN_POINT('Ctrl Pts',(5.72993077911996,-128.81175111262,-9.92453123332976));
#38929=CARTESIAN_POINT('Ctrl Pts',(-1.78726082715848E-11,-128.63675111262,
-9.92453123331945));
#38930=CARTESIAN_POINT('Ctrl Pts',(-5.7299307791557,-128.46175111262,-9.92453123330913));
#38931=CARTESIAN_POINT('Ctrl Pts',(-8.59489616871569,-128.28675111262,-4.96226561664425));
#38932=CARTESIAN_POINT('Ctrl Pts',(-11.4598615582757,-128.11175111262,2.06368086793017E-11));
#38933=CARTESIAN_POINT('Ctrl Pts',(-8.59489616869782,-127.93675111262,4.9622656166752));
#38934=CARTESIAN_POINT('Ctrl Pts',(-5.72993077911996,-127.76175111262,9.92453123332977));
#38935=CARTESIAN_POINT('Ctrl Pts',(1.7871392867044E-11,-127.58675111262,
9.92453123331945));
#38936=CARTESIAN_POINT('Ctrl Pts',(5.7299307791557,-127.41175111262,9.92453123330913));
#38937=CARTESIAN_POINT('Ctrl Pts',(8.59489616871569,-127.23675111262,4.96226561664425));
#38938=CARTESIAN_POINT('Ctrl Pts',(11.4598615582757,-127.06175111262,-2.06354052510241E-11));
#38939=CARTESIAN_POINT('Ctrl Pts',(8.59489616869782,-126.88675111262,-4.9622656166752));
#38940=CARTESIAN_POINT('Ctrl Pts',(5.72993077911996,-126.71175111262,-9.92453123332976));
#38941=CARTESIAN_POINT('Ctrl Pts',(-1.78726082715848E-11,-126.53675111262,
-9.92453123331945));
#38942=CARTESIAN_POINT('Ctrl Pts',(-5.7299307791557,-126.36175111262,-9.92453123330913));
#38943=CARTESIAN_POINT('Ctrl Pts',(-8.59489616871569,-126.18675111262,-4.96226561664425));
#38944=CARTESIAN_POINT('Ctrl Pts',(-11.4598615582757,-126.01175111262,2.06368086793017E-11));
#38945=CARTESIAN_POINT('Ctrl Pts',(-8.59489616869782,-125.83675111262,4.9622656166752));
#38946=CARTESIAN_POINT('Ctrl Pts',(-5.72993077911996,-125.66175111262,9.92453123332977));
#38947=CARTESIAN_POINT('Ctrl Pts',(1.7871392867044E-11,-125.48675111262,
9.92453123331945));
#38948=CARTESIAN_POINT('Ctrl Pts',(5.7299307791557,-125.31175111262,9.92453123330913));
#38949=CARTESIAN_POINT('Ctrl Pts',(8.59489616871569,-125.13675111262,4.96226561664425));
#38950=CARTESIAN_POINT('Ctrl Pts',(11.4598615582757,-124.96175111262,-2.06354052510241E-11));
#38951=CARTESIAN_POINT('Ctrl Pts',(8.59489616869782,-124.78675111262,-4.9622656166752));
#38952=CARTESIAN_POINT('Ctrl Pts',(5.72993077911996,-124.61175111262,-9.92453123332976));
#38953=CARTESIAN_POINT('Ctrl Pts',(-1.78726082715848E-11,-124.43675111262,
-9.92453123331945));
#38954=CARTESIAN_POINT('Ctrl Pts',(-5.7299307791557,-124.26175111262,-9.92453123330913));
#38955=CARTESIAN_POINT('Ctrl Pts',(-8.59489616871569,-124.08675111262,-4.96226561664425));
#38956=CARTESIAN_POINT('Ctrl Pts',(-11.4598615582757,-123.91175111262,2.06368086793017E-11));
#38957=CARTESIAN_POINT('Ctrl Pts',(-8.59489616869782,-123.73675111262,4.9622656166752));
#38958=CARTESIAN_POINT('Ctrl Pts',(-5.72993077911996,-123.56175111262,9.92453123332977));
#38959=CARTESIAN_POINT('Ctrl Pts',(1.7871392867044E-11,-123.38675111262,
9.92453123331945));
#38960=CARTESIAN_POINT('Ctrl Pts',(5.7299307791557,-123.21175111262,9.92453123330913));
#38961=CARTESIAN_POINT('Ctrl Pts',(8.59489616871569,-123.03675111262,4.96226561664425));
#38962=CARTESIAN_POINT('Ctrl Pts',(11.4598615582757,-122.86175111262,-2.06354052510241E-11));
#38963=CARTESIAN_POINT('Ctrl Pts',(8.59489616869782,-122.68675111262,-4.9622656166752));
#38964=CARTESIAN_POINT('Ctrl Pts',(5.72993077911996,-122.51175111262,-9.92453123332976));
#38965=CARTESIAN_POINT('Ctrl Pts',(-1.78726082715848E-11,-122.33675111262,
-9.92453123331945));
#38966=CARTESIAN_POINT('Ctrl Pts',(-5.7299307791557,-122.16175111262,-9.92453123330913));
#38967=CARTESIAN_POINT('Ctrl Pts',(-8.59489616871569,-121.98675111262,-4.96226561664425));
#38968=CARTESIAN_POINT('Ctrl Pts',(-11.4598615582757,-121.81175111262,2.06368086793017E-11));
#38969=CARTESIAN_POINT('Ctrl Pts',(-8.59489616869782,-121.63675111262,4.9622656166752));
#38970=CARTESIAN_POINT('Ctrl Pts',(-5.72993077911996,-121.46175111262,9.92453123332977));
#38971=CARTESIAN_POINT('Ctrl Pts',(1.7871392867044E-11,-121.28675111262,
9.92453123331945));
#38972=CARTESIAN_POINT('Ctrl Pts',(5.7299307791557,-121.11175111262,9.92453123330913));
#38973=CARTESIAN_POINT('Ctrl Pts',(8.59489616871569,-120.93675111262,4.96226561664425));
#38974=CARTESIAN_POINT('Ctrl Pts',(11.4598615582757,-120.76175111262,-2.06354052510241E-11));
#38975=CARTESIAN_POINT('Ctrl Pts',(8.59489616869782,-120.58675111262,-4.9622656166752));
#38976=CARTESIAN_POINT('Ctrl Pts',(5.72993077911996,-120.41175111262,-9.92453123332976));
#38977=CARTESIAN_POINT('Ctrl Pts',(-1.78726082715848E-11,-120.23675111262,
-9.92453123331945));
#38978=CARTESIAN_POINT('Ctrl Pts',(-5.7299307791557,-120.06175111262,-9.92453123330913));
#38979=CARTESIAN_POINT('Ctrl Pts',(-8.59489616871569,-119.88675111262,-4.96226561664425));
#38980=CARTESIAN_POINT('Ctrl Pts',(-11.4598615582757,-119.71175111262,2.06368086793017E-11));
#38981=CARTESIAN_POINT('Ctrl Pts',(-8.59489616869782,-119.53675111262,4.9622656166752));
#38982=CARTESIAN_POINT('Ctrl Pts',(-5.72993077911996,-119.36175111262,9.92453123332977));
#38983=CARTESIAN_POINT('Ctrl Pts',(1.7871392867044E-11,-119.18675111262,
9.92453123331945));
#38984=CARTESIAN_POINT('Ctrl Pts',(5.7299307791557,-119.01175111262,9.92453123330913));
#38985=CARTESIAN_POINT('Ctrl Pts',(8.59489616871569,-118.83675111262,4.96226561664425));
#38986=CARTESIAN_POINT('Ctrl Pts',(11.4598615582757,-118.66175111262,-2.06354052510241E-11));
#38987=CARTESIAN_POINT('Ctrl Pts',(8.59489616869782,-118.48675111262,-4.9622656166752));
#38988=CARTESIAN_POINT('Ctrl Pts',(5.72993077911996,-118.31175111262,-9.92453123332976));
#38989=CARTESIAN_POINT('Ctrl Pts',(-1.78726082715848E-11,-118.13675111262,
-9.92453123331945));
#38990=CARTESIAN_POINT('Ctrl Pts',(-5.7299307791557,-117.96175111262,-9.92453123330913));
#38991=CARTESIAN_POINT('Ctrl Pts',(-8.59489616871569,-117.78675111262,-4.96226561664425));
#38992=CARTESIAN_POINT('Ctrl Pts',(-11.4598615582757,-117.61175111262,2.06368086793017E-11));
#38993=CARTESIAN_POINT('Ctrl Pts',(-8.59489616869782,-117.43675111262,4.9622656166752));
#38994=CARTESIAN_POINT('Ctrl Pts',(-5.72993077911996,-117.26175111262,9.92453123332977));
#38995=CARTESIAN_POINT('Ctrl Pts',(1.7871392867044E-11,-117.08675111262,
9.92453123331945));
#38996=CARTESIAN_POINT('Ctrl Pts',(5.7299307791557,-116.91175111262,9.92453123330913));
#38997=CARTESIAN_POINT('Ctrl Pts',(8.59489616871569,-116.73675111262,4.96226561664425));
#38998=CARTESIAN_POINT('Ctrl Pts',(11.4598615582757,-116.56175111262,-2.06354052510241E-11));
#38999=CARTESIAN_POINT('Ctrl Pts',(8.59489616869782,-116.38675111262,-4.9622656166752));
#39000=CARTESIAN_POINT('Ctrl Pts',(5.72993077911996,-116.21175111262,-9.92453123332976));
#39001=CARTESIAN_POINT('Ctrl Pts',(-1.78726082715848E-11,-116.03675111262,
-9.92453123331945));
#39002=CARTESIAN_POINT('Ctrl Pts',(-5.7299307791557,-115.86175111262,-9.92453123330913));
#39003=CARTESIAN_POINT('Ctrl Pts',(-8.59489616871569,-115.68675111262,-4.96226561664425));
#39004=CARTESIAN_POINT('Ctrl Pts',(-11.4598615582757,-115.51175111262,2.06368086793017E-11));
#39005=CARTESIAN_POINT('Ctrl Pts',(-8.59489616869782,-115.33675111262,4.9622656166752));
#39006=CARTESIAN_POINT('Ctrl Pts',(-5.72993077911996,-115.16175111262,9.92453123332977));
#39007=CARTESIAN_POINT('Ctrl Pts',(1.7871392867044E-11,-114.98675111262,
9.92453123331945));
#39008=CARTESIAN_POINT('Ctrl Pts',(5.7299307791557,-114.81175111262,9.92453123330913));
#39009=CARTESIAN_POINT('Ctrl Pts',(8.59489616871569,-114.63675111262,4.96226561664425));
#39010=CARTESIAN_POINT('Ctrl Pts',(11.4598615582757,-114.46175111262,-2.06354052510241E-11));
#39011=CARTESIAN_POINT('Ctrl Pts',(8.59489616869782,-114.28675111262,-4.9622656166752));
#39012=CARTESIAN_POINT('Ctrl Pts',(5.72993077911996,-114.11175111262,-9.92453123332976));
#39013=CARTESIAN_POINT('Ctrl Pts',(-1.78726082715848E-11,-113.93675111262,
-9.92453123331945));
#39014=CARTESIAN_POINT('Ctrl Pts',(-5.7299307791557,-113.76175111262,-9.92453123330913));
#39015=CARTESIAN_POINT('Ctrl Pts',(-8.59489616871569,-113.58675111262,-4.96226561664425));
#39016=CARTESIAN_POINT('Ctrl Pts',(-11.4598615582757,-113.41175111262,2.06368086793017E-11));
#39017=CARTESIAN_POINT('Ctrl Pts',(-8.59489616869782,-113.23675111262,4.9622656166752));
#39018=CARTESIAN_POINT('Ctrl Pts',(-5.72993077911996,-113.06175111262,9.92453123332977));
#39019=CARTESIAN_POINT('Ctrl Pts',(1.7871392867044E-11,-112.88675111262,
9.92453123331945));
#39020=CARTESIAN_POINT('Ctrl Pts',(5.7299307791557,-112.71175111262,9.92453123330913));
#39021=CARTESIAN_POINT('Ctrl Pts',(8.59489616871569,-112.53675111262,4.96226561664425));
#39022=CARTESIAN_POINT('Ctrl Pts',(11.4598615582757,-112.36175111262,-2.06354052510241E-11));
#39023=CARTESIAN_POINT('Ctrl Pts',(8.59489616869782,-112.18675111262,-4.9622656166752));
#39024=CARTESIAN_POINT('Ctrl Pts',(5.72993077911996,-112.01175111262,-9.92453123332976));
#39025=CARTESIAN_POINT('Ctrl Pts',(-1.78726082715848E-11,-111.83675111262,
-9.92453123331945));
#39026=CARTESIAN_POINT('Ctrl Pts',(-5.7299307791557,-111.66175111262,-9.92453123330913));
#39027=CARTESIAN_POINT('Ctrl Pts',(-8.59489616871569,-111.48675111262,-4.96226561664425));
#39028=CARTESIAN_POINT('Ctrl Pts',(-11.4598615582757,-111.31175111262,2.06368086793017E-11));
#39029=CARTESIAN_POINT('Ctrl Pts',(-8.59489616869782,-111.13675111262,4.9622656166752));
#39030=CARTESIAN_POINT('Ctrl Pts',(-5.72993077911996,-110.96175111262,9.92453123332977));
#39031=CARTESIAN_POINT('Ctrl Pts',(1.7871392867044E-11,-110.78675111262,
9.92453123331945));
#39032=CARTESIAN_POINT('Ctrl Pts',(5.7299307791557,-110.61175111262,9.92453123330913));
#39033=CARTESIAN_POINT('Ctrl Pts',(8.59489616871569,-110.43675111262,4.96226561664425));
#39034=CARTESIAN_POINT('Ctrl Pts',(11.4598615582757,-110.26175111262,-2.06354052510241E-11));
#39035=CARTESIAN_POINT('Ctrl Pts',(8.59489616869782,-110.08675111262,-4.9622656166752));
#39036=CARTESIAN_POINT('Ctrl Pts',(5.72993077911996,-109.91175111262,-9.92453123332976));
#39037=CARTESIAN_POINT('Ctrl Pts',(-1.78726082715848E-11,-109.73675111262,
-9.92453123331945));
#39038=CARTESIAN_POINT('Ctrl Pts',(-5.7299307791557,-109.56175111262,-9.92453123330913));
#39039=CARTESIAN_POINT('Ctrl Pts',(-8.59489616871569,-109.38675111262,-4.96226561664425));
#39040=CARTESIAN_POINT('Ctrl Pts',(-11.4598615582757,-109.21175111262,2.06368086793017E-11));
#39041=CARTESIAN_POINT('Ctrl Pts',(-8.59489616869782,-109.03675111262,4.9622656166752));
#39042=CARTESIAN_POINT('Ctrl Pts',(-5.72993077911996,-108.86175111262,9.92453123332977));
#39043=CARTESIAN_POINT('Ctrl Pts',(1.7871392867044E-11,-108.68675111262,
9.92453123331945));
#39044=CARTESIAN_POINT('Ctrl Pts',(5.7299307791557,-108.51175111262,9.92453123330913));
#39045=CARTESIAN_POINT('Ctrl Pts',(8.59489616871569,-108.33675111262,4.96226561664425));
#39046=CARTESIAN_POINT('Ctrl Pts',(11.4598615582757,-108.16175111262,-2.06354052510241E-11));
#39047=CARTESIAN_POINT('Ctrl Pts',(8.59489616869782,-107.98675111262,-4.9622656166752));
#39048=CARTESIAN_POINT('Ctrl Pts',(5.72993077911996,-107.81175111262,-9.92453123332976));
#39049=CARTESIAN_POINT('Ctrl Pts',(-1.78726082715848E-11,-107.63675111262,
-9.92453123331945));
#39050=CARTESIAN_POINT('Ctrl Pts',(-5.7299307791557,-107.46175111262,-9.92453123330913));
#39051=CARTESIAN_POINT('Ctrl Pts',(-8.59489616871569,-107.28675111262,-4.96226561664425));
#39052=CARTESIAN_POINT('Ctrl Pts',(-11.4598615582757,-107.11175111262,2.06368086793017E-11));
#39053=CARTESIAN_POINT('Ctrl Pts',(-8.59489616869782,-106.93675111262,4.9622656166752));
#39054=CARTESIAN_POINT('Ctrl Pts',(-5.72993077911996,-106.76175111262,9.92453123332977));
#39055=CARTESIAN_POINT('Ctrl Pts',(1.7871392867044E-11,-106.58675111262,
9.92453123331945));
#39056=CARTESIAN_POINT('Ctrl Pts',(5.7299307791557,-106.41175111262,9.92453123330913));
#39057=CARTESIAN_POINT('Ctrl Pts',(8.59489616871569,-106.23675111262,4.96226561664425));
#39058=CARTESIAN_POINT('Ctrl Pts',(11.4598615582757,-106.06175111262,-2.06354052510241E-11));
#39059=CARTESIAN_POINT('Ctrl Pts',(8.59489616869782,-105.88675111262,-4.9622656166752));
#39060=CARTESIAN_POINT('Ctrl Pts',(5.72993077911996,-105.71175111262,-9.92453123332976));
#39061=CARTESIAN_POINT('Ctrl Pts',(-1.78726082715848E-11,-105.53675111262,
-9.92453123331945));
#39062=CARTESIAN_POINT('Ctrl Pts',(-5.7299307791557,-105.36175111262,-9.92453123330913));
#39063=CARTESIAN_POINT('Ctrl Pts',(-8.59489616871569,-105.18675111262,-4.96226561664425));
#39064=CARTESIAN_POINT('Ctrl Pts',(-11.4598615582757,-105.01175111262,2.06368086793017E-11));
#39065=CARTESIAN_POINT('Ctrl Pts',(-8.59489616869782,-104.83675111262,4.9622656166752));
#39066=CARTESIAN_POINT('Ctrl Pts',(-5.72993077911996,-104.66175111262,9.92453123332977));
#39067=CARTESIAN_POINT('Ctrl Pts',(1.7871392867044E-11,-104.48675111262,
9.92453123331945));
#39068=CARTESIAN_POINT('Ctrl Pts',(5.7299307791557,-104.31175111262,9.92453123330913));
#39069=CARTESIAN_POINT('Ctrl Pts',(8.59489616871569,-104.13675111262,4.96226561664425));
#39070=CARTESIAN_POINT('Ctrl Pts',(11.4598615582757,-103.96175111262,-2.06354052510241E-11));
#39071=CARTESIAN_POINT('Ctrl Pts',(8.59489616869782,-103.78675111262,-4.9622656166752));
#39072=CARTESIAN_POINT('Ctrl Pts',(5.72993077911996,-103.61175111262,-9.92453123332976));
#39073=CARTESIAN_POINT('Ctrl Pts',(-1.78726082715848E-11,-103.43675111262,
-9.92453123331945));
#39074=CARTESIAN_POINT('Ctrl Pts',(-5.7299307791557,-103.26175111262,-9.92453123330913));
#39075=CARTESIAN_POINT('Ctrl Pts',(-8.59489616871569,-103.08675111262,-4.96226561664425));
#39076=CARTESIAN_POINT('Ctrl Pts',(-11.4598615582757,-102.91175111262,2.06368086793017E-11));
#39077=CARTESIAN_POINT('Ctrl Pts',(-8.59489616869782,-102.73675111262,4.9622656166752));
#39078=CARTESIAN_POINT('Ctrl Pts',(-5.72993077911996,-102.56175111262,9.92453123332977));
#39079=CARTESIAN_POINT('Ctrl Pts',(1.7871392867044E-11,-102.38675111262,
9.92453123331945));
#39080=CARTESIAN_POINT('Ctrl Pts',(5.7299307791557,-102.21175111262,9.92453123330913));
#39081=CARTESIAN_POINT('Ctrl Pts',(8.59489616871569,-102.03675111262,4.96226561664425));
#39082=CARTESIAN_POINT('Ctrl Pts',(11.4598615582757,-101.86175111262,-2.06354052510241E-11));
#39083=CARTESIAN_POINT('Ctrl Pts',(8.59489616869782,-101.68675111262,-4.9622656166752));
#39084=CARTESIAN_POINT('Ctrl Pts',(5.72993077911996,-101.51175111262,-9.92453123332976));
#39085=CARTESIAN_POINT('Ctrl Pts',(-1.78726082715848E-11,-101.33675111262,
-9.92453123331945));
#39086=CARTESIAN_POINT('Ctrl Pts',(-5.7299307791557,-101.16175111262,-9.92453123330913));
#39087=CARTESIAN_POINT('Ctrl Pts',(-8.59489616871569,-100.98675111262,-4.96226561664425));
#39088=CARTESIAN_POINT('Ctrl Pts',(-11.4598615582757,-100.81175111262,2.06368086793017E-11));
#39089=CARTESIAN_POINT('Ctrl Pts',(-8.59489616869782,-100.63675111262,4.9622656166752));
#39090=CARTESIAN_POINT('Ctrl Pts',(-5.72993077911996,-100.46175111262,9.92453123332977));
#39091=CARTESIAN_POINT('Ctrl Pts',(1.7871392867044E-11,-100.28675111262,
9.92453123331945));
#39092=CARTESIAN_POINT('Ctrl Pts',(5.7299307791557,-100.11175111262,9.92453123330913));
#39093=CARTESIAN_POINT('Ctrl Pts',(8.59489616871569,-99.9367511126202,4.96226561664425));
#39094=CARTESIAN_POINT('Ctrl Pts',(11.4598615582757,-99.7617511126202,-2.06354052510241E-11));
#39095=CARTESIAN_POINT('Ctrl Pts',(8.59489616869782,-99.5867511126202,-4.9622656166752));
#39096=CARTESIAN_POINT('Ctrl Pts',(5.72993077911996,-99.4117511126202,-9.92453123332976));
#39097=CARTESIAN_POINT('Ctrl Pts',(-1.78726082715848E-11,-99.2367511126202,
-9.92453123331945));
#39098=CARTESIAN_POINT('Ctrl Pts',(-5.7299307791557,-99.0617511126202,-9.92453123330913));
#39099=CARTESIAN_POINT('Ctrl Pts',(-8.59489616871569,-98.8867511126202,
-4.96226561664425));
#39100=CARTESIAN_POINT('Ctrl Pts',(-11.4598615582757,-98.7117511126202,
2.06368086793017E-11));
#39101=CARTESIAN_POINT('Ctrl Pts',(-8.59489616869782,-98.5367511126202,
4.9622656166752));
#39102=CARTESIAN_POINT('Ctrl Pts',(-5.72993077911996,-98.3617511126202,
9.92453123332977));
#39103=CARTESIAN_POINT('Ctrl Pts',(1.7871392867044E-11,-98.1867511126202,
9.92453123331945));
#39104=CARTESIAN_POINT('Ctrl Pts',(5.7299307791557,-98.0117511126202,9.92453123330913));
#39105=CARTESIAN_POINT('Ctrl Pts',(8.59489616871569,-97.8367511126202,4.96226561664425));
#39106=CARTESIAN_POINT('Ctrl Pts',(11.4598615582757,-97.6617511126202,-2.06354052510241E-11));
#39107=CARTESIAN_POINT('Ctrl Pts',(8.59489616869782,-97.4867511126202,-4.9622656166752));
#39108=CARTESIAN_POINT('Ctrl Pts',(5.72993077911996,-97.3117511126202,-9.92453123332976));
#39109=CARTESIAN_POINT('Ctrl Pts',(-1.78726082715848E-11,-97.1367511126202,
-9.92453123331945));
#39110=CARTESIAN_POINT('Ctrl Pts',(-5.7299307791557,-96.9617511126202,-9.92453123330913));
#39111=CARTESIAN_POINT('Ctrl Pts',(-8.59489616871569,-96.7867511126202,
-4.96226561664425));
#39112=CARTESIAN_POINT('Ctrl Pts',(-11.4598615582757,-96.6117511126202,
2.06368086793017E-11));
#39113=CARTESIAN_POINT('Ctrl Pts',(-8.59489616869782,-96.4367511126202,
4.9622656166752));
#39114=CARTESIAN_POINT('Ctrl Pts',(-5.72993077911996,-96.2617511126202,
9.92453123332977));
#39115=CARTESIAN_POINT('Ctrl Pts',(1.7871392867044E-11,-96.0867511126202,
9.92453123331945));
#39116=CARTESIAN_POINT('Ctrl Pts',(5.7299307791557,-95.9117511126202,9.92453123330913));
#39117=CARTESIAN_POINT('Ctrl Pts',(8.59489616871569,-95.7367511126202,4.96226561664425));
#39118=CARTESIAN_POINT('Ctrl Pts',(11.4598615582757,-95.5617511126202,-2.06354052510241E-11));
#39119=CARTESIAN_POINT('Ctrl Pts',(8.59489616869782,-95.3867511126202,-4.9622656166752));
#39120=CARTESIAN_POINT('Ctrl Pts',(5.72993077911996,-95.2117511126202,-9.92453123332976));
#39121=CARTESIAN_POINT('Ctrl Pts',(-1.78726082715848E-11,-95.0367511126202,
-9.92453123331945));
#39122=CARTESIAN_POINT('Ctrl Pts',(-5.7299307791557,-94.8617511126203,-9.92453123330913));
#39123=CARTESIAN_POINT('Ctrl Pts',(-8.59489616871569,-94.6867511126202,
-4.96226561664425));
#39124=CARTESIAN_POINT('Ctrl Pts',(-11.4598615582757,-94.5117511126202,
2.06368086793017E-11));
#39125=CARTESIAN_POINT('Ctrl Pts',(-8.59489616869782,-94.3367511126202,
4.9622656166752));
#39126=CARTESIAN_POINT('Ctrl Pts',(-5.72993077911996,-94.1617511126202,
9.92453123332977));
#39127=CARTESIAN_POINT('Ctrl Pts',(1.7871392867044E-11,-93.9867511126202,
9.92453123331945));
#39128=CARTESIAN_POINT('Ctrl Pts',(5.7299307791557,-93.8117511126202,9.92453123330913));
#39129=CARTESIAN_POINT('Ctrl Pts',(8.59489616871569,-93.6367511126202,4.96226561664425));
#39130=CARTESIAN_POINT('Ctrl Pts',(11.4598615582757,-93.4617511126202,-2.06354052510241E-11));
#39131=CARTESIAN_POINT('Ctrl Pts',(8.59489616869782,-93.2867511126202,-4.9622656166752));
#39132=CARTESIAN_POINT('Ctrl Pts',(5.72993077911996,-93.1117511126202,-9.92453123332976));
#39133=CARTESIAN_POINT('Ctrl Pts',(-1.78726082715848E-11,-92.9367511126202,
-9.92453123331945));
#39134=CARTESIAN_POINT('Ctrl Pts',(-5.7299307791557,-92.7617511126202,-9.92453123330913));
#39135=CARTESIAN_POINT('Ctrl Pts',(-8.59489616871569,-92.5867511126202,
-4.96226561664425));
#39136=CARTESIAN_POINT('Ctrl Pts',(-11.4598615582757,-92.4117511126202,
2.06368086793017E-11));
#39137=CARTESIAN_POINT('Ctrl Pts',(-8.59489616869782,-92.2367511126202,
4.9622656166752));
#39138=CARTESIAN_POINT('Ctrl Pts',(-5.72993077911996,-92.0617511126202,
9.92453123332977));
#39139=CARTESIAN_POINT('Ctrl Pts',(1.7871392867044E-11,-91.8867511126202,
9.92453123331945));
#39140=CARTESIAN_POINT('Ctrl Pts',(5.7299307791557,-91.7117511126202,9.92453123330913));
#39141=CARTESIAN_POINT('Ctrl Pts',(8.59489616871569,-91.5367511126202,4.96226561664425));
#39142=CARTESIAN_POINT('Ctrl Pts',(11.4598615582757,-91.3617511126203,-2.06354052510241E-11));
#39143=CARTESIAN_POINT('Ctrl Pts',(8.59489616869782,-91.1867511126202,-4.9622656166752));
#39144=CARTESIAN_POINT('Ctrl Pts',(5.72993077911996,-91.0117511126202,-9.92453123332976));
#39145=CARTESIAN_POINT('Ctrl Pts',(-1.78726082715848E-11,-90.8367511126202,
-9.92453123331945));
#39146=CARTESIAN_POINT('Ctrl Pts',(-5.7299307791557,-90.6617511126203,-9.92453123330913));
#39147=CARTESIAN_POINT('Ctrl Pts',(-8.59489616871569,-90.4867511126203,
-4.96226561664425));
#39148=CARTESIAN_POINT('Ctrl Pts',(-11.4598615582757,-90.3117511126203,
2.06368086793017E-11));
#39149=CARTESIAN_POINT('Ctrl Pts',(-8.59489616869782,-90.1367511126202,
4.9622656166752));
#39150=CARTESIAN_POINT('Ctrl Pts',(-5.72993077911996,-89.9617511126202,
9.92453123332977));
#39151=CARTESIAN_POINT('Ctrl Pts',(1.7871392867044E-11,-89.7867511126202,
9.92453123331945));
#39152=CARTESIAN_POINT('Ctrl Pts',(5.7299307791557,-89.6117511126202,9.92453123330913));
#39153=CARTESIAN_POINT('Ctrl Pts',(8.59489616871569,-89.4367511126202,4.96226561664425));
#39154=CARTESIAN_POINT('Ctrl Pts',(11.4598615582757,-89.2617511126202,-2.06354052510241E-11));
#39155=CARTESIAN_POINT('Ctrl Pts',(8.59489616869782,-89.0867511126202,-4.9622656166752));
#39156=CARTESIAN_POINT('Ctrl Pts',(5.72993077911996,-88.9117511126203,-9.92453123332976));
#39157=CARTESIAN_POINT('Ctrl Pts',(-1.78726082715848E-11,-88.7367511126203,
-9.92453123331945));
#39158=CARTESIAN_POINT('Ctrl Pts',(-5.7299307791557,-88.5617511126202,-9.92453123330913));
#39159=CARTESIAN_POINT('Ctrl Pts',(-8.59489616871569,-88.3867511126203,
-4.96226561664425));
#39160=CARTESIAN_POINT('Ctrl Pts',(-11.4598615582757,-88.2117511126202,
2.06368086793017E-11));
#39161=CARTESIAN_POINT('Ctrl Pts',(-8.59489616869782,-88.0367511126202,
4.9622656166752));
#39162=CARTESIAN_POINT('Ctrl Pts',(-5.72993077911996,-87.8617511126202,
9.92453123332977));
#39163=CARTESIAN_POINT('Ctrl Pts',(1.7871392867044E-11,-87.6867511126203,
9.92453123331945));
#39164=CARTESIAN_POINT('Ctrl Pts',(5.7299307791557,-87.5117511126203,9.92453123330913));
#39165=CARTESIAN_POINT('Ctrl Pts',(8.59489616871569,-87.3367511126202,4.96226561664425));
#39166=CARTESIAN_POINT('Ctrl Pts',(11.4598615582757,-87.1617511126203,-2.06354052510241E-11));
#39167=CARTESIAN_POINT('Ctrl Pts',(8.59489616869782,-86.9867511126203,-4.9622656166752));
#39168=CARTESIAN_POINT('Ctrl Pts',(5.72993077911996,-86.8117511126202,-9.92453123332976));
#39169=CARTESIAN_POINT('Ctrl Pts',(-1.78726082715848E-11,-86.6367511126203,
-9.92453123331945));
#39170=CARTESIAN_POINT('Ctrl Pts',(-5.7299307791557,-86.4617511126202,-9.92453123330913));
#39171=CARTESIAN_POINT('Ctrl Pts',(-8.59489616871569,-86.2867511126203,
-4.96226561664425));
#39172=CARTESIAN_POINT('Ctrl Pts',(-11.4598615582757,-86.1117511126203,
2.06368086793017E-11));
#39173=CARTESIAN_POINT('Ctrl Pts',(-8.59489616869782,-85.9367511126203,
4.9622656166752));
#39174=CARTESIAN_POINT('Ctrl Pts',(-5.72993077911996,-85.7617511126202,
9.92453123332977));
#39175=CARTESIAN_POINT('Ctrl Pts',(1.7871392867044E-11,-85.5867511126203,
9.92453123331945));
#39176=CARTESIAN_POINT('Ctrl Pts',(5.7299307791557,-85.4117511126203,9.92453123330913));
#39177=CARTESIAN_POINT('Ctrl Pts',(8.59489616871569,-85.2367511126202,4.96226561664425));
#39178=CARTESIAN_POINT('Ctrl Pts',(11.4598615582757,-85.0617511126203,-2.06354052510241E-11));
#39179=CARTESIAN_POINT('Ctrl Pts',(8.59489616869782,-84.8867511126203,-4.9622656166752));
#39180=CARTESIAN_POINT('Ctrl Pts',(5.72993077911996,-84.7117511126202,-9.92453123332976));
#39181=CARTESIAN_POINT('Ctrl Pts',(-1.78726082715848E-11,-84.5367511126202,
-9.92453123331945));
#39182=CARTESIAN_POINT('Ctrl Pts',(-5.7299307791557,-84.3617511126203,-9.92453123330913));
#39183=CARTESIAN_POINT('Ctrl Pts',(-8.59489616871569,-84.1867511126203,
-4.96226561664425));
#39184=CARTESIAN_POINT('Ctrl Pts',(-11.4598615582757,-84.0117511126203,
2.06368086793017E-11));
#39185=CARTESIAN_POINT('Ctrl Pts',(-8.59489616869782,-83.8367511126203,
4.9622656166752));
#39186=CARTESIAN_POINT('Ctrl Pts',(-5.72993077911996,-83.6617511126203,
9.92453123332977));
#39187=CARTESIAN_POINT('Ctrl Pts',(1.7871392867044E-11,-83.4867511126202,
9.92453123331945));
#39188=CARTESIAN_POINT('Ctrl Pts',(5.7299307791557,-83.3117511126203,9.92453123330913));
#39189=CARTESIAN_POINT('Ctrl Pts',(8.59489616871569,-83.1367511126203,4.96226561664425));
#39190=CARTESIAN_POINT('Ctrl Pts',(11.4598615582757,-82.9617511126203,-2.06354052510241E-11));
#39191=CARTESIAN_POINT('Ctrl Pts',(8.59489616869782,-82.7867511126203,-4.9622656166752));
#39192=CARTESIAN_POINT('Ctrl Pts',(5.72993077911996,-82.6117511126203,-9.92453123332976));
#39193=CARTESIAN_POINT('Ctrl Pts',(-1.78726082715848E-11,-82.4367511126202,
-9.92453123331945));
#39194=CARTESIAN_POINT('Ctrl Pts',(-5.7299307791557,-82.2617511126203,-9.92453123330913));
#39195=CARTESIAN_POINT('Ctrl Pts',(-8.59489616871569,-82.0867511126203,
-4.96226561664425));
#39196=CARTESIAN_POINT('Ctrl Pts',(-11.4598615582757,-81.9117511126203,
2.06368086793017E-11));
#39197=CARTESIAN_POINT('Ctrl Pts',(-8.59489616869782,-81.7367511126203,
4.9622656166752));
#39198=CARTESIAN_POINT('Ctrl Pts',(-5.72993077911996,-81.5617511126202,
9.92453123332977));
#39199=CARTESIAN_POINT('Ctrl Pts',(1.7871392867044E-11,-81.3867511126203,
9.92453123331945));
#39200=CARTESIAN_POINT('Ctrl Pts',(5.7299307791557,-81.2117511126203,9.92453123330913));
#39201=CARTESIAN_POINT('Ctrl Pts',(8.59489616871569,-81.0367511126203,4.96226561664425));
#39202=CARTESIAN_POINT('Ctrl Pts',(11.4598615582757,-80.8617511126203,-2.06354052510241E-11));
#39203=CARTESIAN_POINT('Ctrl Pts',(8.59489616869782,-80.6867511126203,-4.9622656166752));
#39204=CARTESIAN_POINT('Ctrl Pts',(5.72993077911996,-80.5117511126203,-9.92453123332976));
#39205=CARTESIAN_POINT('Ctrl Pts',(-1.78726082715848E-11,-80.3367511126203,
-9.92453123331945));
#39206=CARTESIAN_POINT('Ctrl Pts',(-5.7299307791557,-80.1617511126202,-9.92453123330913));
#39207=CARTESIAN_POINT('Ctrl Pts',(-8.59489616871569,-79.9867511126203,
-4.96226561664425));
#39208=CARTESIAN_POINT('Ctrl Pts',(-11.4598615582757,-79.8117511126203,
2.06368086793017E-11));
#39209=CARTESIAN_POINT('Ctrl Pts',(-8.59489616869782,-79.6367511126202,
4.9622656166752));
#39210=CARTESIAN_POINT('Ctrl Pts',(-5.72993077911996,-79.4617511126203,
9.92453123332977));
#39211=CARTESIAN_POINT('Ctrl Pts',(1.7871392867044E-11,-79.2867511126203,
9.92453123331945));
#39212=CARTESIAN_POINT('Ctrl Pts',(5.7299307791557,-79.1117511126203,9.92453123330913));
#39213=CARTESIAN_POINT('Ctrl Pts',(8.59489616871569,-78.9367511126203,4.96226561664425));
#39214=CARTESIAN_POINT('Ctrl Pts',(11.4598615582757,-78.7617511126203,-2.06354052510241E-11));
#39215=CARTESIAN_POINT('Ctrl Pts',(8.59489616869782,-78.5867511126203,-4.9622656166752));
#39216=CARTESIAN_POINT('Ctrl Pts',(5.72993077911996,-78.4117511126203,-9.92453123332976));
#39217=CARTESIAN_POINT('Ctrl Pts',(-1.78726082715848E-11,-78.2367511126203,
-9.92453123331945));
#39218=CARTESIAN_POINT('Ctrl Pts',(-5.7299307791557,-78.0617511126203,-9.92453123330913));
#39219=CARTESIAN_POINT('Ctrl Pts',(-8.59489616871569,-77.8867511126203,
-4.96226561664425));
#39220=CARTESIAN_POINT('Ctrl Pts',(-11.4598615582757,-77.7117511126203,
2.06368086793017E-11));
#39221=CARTESIAN_POINT('Ctrl Pts',(-8.59489616869782,-77.5367511126203,
4.9622656166752));
#39222=CARTESIAN_POINT('Ctrl Pts',(-5.72993077911996,-77.3617511126203,
9.92453123332977));
#39223=CARTESIAN_POINT('Ctrl Pts',(1.7871392867044E-11,-77.1867511126203,
9.92453123331945));
#39224=CARTESIAN_POINT('Ctrl Pts',(5.7299307791557,-77.0117511126203,9.92453123330913));
#39225=CARTESIAN_POINT('Ctrl Pts',(8.59489616871569,-76.8367511126203,4.96226561664425));
#39226=CARTESIAN_POINT('Ctrl Pts',(11.4598615582757,-76.6617511126203,-2.06354052510241E-11));
#39227=CARTESIAN_POINT('Ctrl Pts',(8.59489616869782,-76.4867511126203,-4.9622656166752));
#39228=CARTESIAN_POINT('Ctrl Pts',(5.72993077911996,-76.3117511126203,-9.92453123332976));
#39229=CARTESIAN_POINT('Ctrl Pts',(-1.78726082715848E-11,-76.1367511126203,
-9.92453123331945));
#39230=CARTESIAN_POINT('Ctrl Pts',(-5.7299307791557,-75.9617511126203,-9.92453123330913));
#39231=CARTESIAN_POINT('Ctrl Pts',(-8.59489616871569,-75.7867511126203,
-4.96226561664425));
#39232=CARTESIAN_POINT('Ctrl Pts',(-11.4598615582757,-75.6117511126203,
2.06368086793017E-11));
#39233=CARTESIAN_POINT('Ctrl Pts',(-8.59489616869782,-75.4367511126203,
4.9622656166752));
#39234=CARTESIAN_POINT('Ctrl Pts',(-5.72993077911996,-75.2617511126203,
9.92453123332977));
#39235=CARTESIAN_POINT('Ctrl Pts',(1.7871392867044E-11,-75.0867511126203,
9.92453123331945));
#39236=CARTESIAN_POINT('Ctrl Pts',(5.7299307791557,-74.9117511126203,9.92453123330913));
#39237=CARTESIAN_POINT('Ctrl Pts',(8.59489616871569,-74.7367511126203,4.96226561664425));
#39238=CARTESIAN_POINT('Ctrl Pts',(11.4598615582757,-74.5617511126203,-2.06354052510241E-11));
#39239=CARTESIAN_POINT('Ctrl Pts',(8.59489616869782,-74.3867511126203,-4.9622656166752));
#39240=CARTESIAN_POINT('Ctrl Pts',(5.72993077911996,-74.2117511126203,-9.92453123332976));
#39241=CARTESIAN_POINT('Ctrl Pts',(-1.78726082715848E-11,-74.0367511126203,
-9.92453123331945));
#39242=CARTESIAN_POINT('Ctrl Pts',(-5.7299307791557,-73.8617511126203,-9.92453123330913));
#39243=CARTESIAN_POINT('Ctrl Pts',(-8.59489616871569,-73.6867511126203,
-4.96226561664425));
#39244=CARTESIAN_POINT('Ctrl Pts',(-11.4598615582757,-73.5117511126203,
2.06368086793017E-11));
#39245=CARTESIAN_POINT('Ctrl Pts',(-8.59489616869782,-73.3367511126203,
4.9622656166752));
#39246=CARTESIAN_POINT('Ctrl Pts',(-5.72993077911996,-73.1617511126203,
9.92453123332977));
#39247=CARTESIAN_POINT('Ctrl Pts',(1.7871392867044E-11,-72.9867511126203,
9.92453123331945));
#39248=CARTESIAN_POINT('Ctrl Pts',(5.7299307791557,-72.8117511126203,9.92453123330913));
#39249=CARTESIAN_POINT('Ctrl Pts',(8.59489616871569,-72.6367511126203,4.96226561664425));
#39250=CARTESIAN_POINT('Ctrl Pts',(11.4598615582757,-72.4617511126203,-2.06354052510241E-11));
#39251=CARTESIAN_POINT('Ctrl Pts',(8.59489616869782,-72.2867511126203,-4.9622656166752));
#39252=CARTESIAN_POINT('Ctrl Pts',(5.72993077911996,-72.1117511126203,-9.92453123332976));
#39253=CARTESIAN_POINT('Ctrl Pts',(-1.78726082715848E-11,-71.9367511126203,
-9.92453123331945));
#39254=CARTESIAN_POINT('Ctrl Pts',(-5.7299307791557,-71.7617511126203,-9.92453123330913));
#39255=CARTESIAN_POINT('Ctrl Pts',(-8.59489616871569,-71.5867511126203,
-4.96226561664425));
#39256=CARTESIAN_POINT('Ctrl Pts',(-11.4598615582757,-71.4117511126203,
2.06368086793017E-11));
#39257=CARTESIAN_POINT('Ctrl Pts',(-8.59489616869782,-71.2367511126203,
4.9622656166752));
#39258=CARTESIAN_POINT('Ctrl Pts',(-5.72993077911996,-71.0617511126203,
9.92453123332977));
#39259=CARTESIAN_POINT('Ctrl Pts',(1.7871392867044E-11,-70.8867511126203,
9.92453123331945));
#39260=CARTESIAN_POINT('Ctrl Pts',(5.7299307791557,-70.7117511126203,9.92453123330913));
#39261=CARTESIAN_POINT('Ctrl Pts',(8.59489616871569,-70.5367511126203,4.96226561664425));
#39262=CARTESIAN_POINT('Ctrl Pts',(11.4598615582757,-70.3617511126203,-2.06354052510241E-11));
#39263=CARTESIAN_POINT('Ctrl Pts',(8.59489616869782,-70.1867511126203,-4.9622656166752));
#39264=CARTESIAN_POINT('Ctrl Pts',(5.72993077911996,-70.0117511126203,-9.92453123332976));
#39265=CARTESIAN_POINT('Ctrl Pts',(-1.78726082715848E-11,-69.8367511126203,
-9.92453123331945));
#39266=CARTESIAN_POINT('Ctrl Pts',(-5.7299307791557,-69.6617511126203,-9.92453123330913));
#39267=CARTESIAN_POINT('Ctrl Pts',(-8.59489616871569,-69.4867511126203,
-4.96226561664425));
#39268=CARTESIAN_POINT('Ctrl Pts',(-11.4598615582757,-69.3117511126203,
2.06368086793017E-11));
#39269=CARTESIAN_POINT('Ctrl Pts',(-8.59489616869782,-69.1367511126203,
4.9622656166752));
#39270=CARTESIAN_POINT('Ctrl Pts',(-5.72993077911996,-68.9617511126203,
9.92453123332977));
#39271=CARTESIAN_POINT('Ctrl Pts',(1.7871392867044E-11,-68.7867511126203,
9.92453123331945));
#39272=CARTESIAN_POINT('Ctrl Pts',(5.7299307791557,-68.6117511126203,9.92453123330913));
#39273=CARTESIAN_POINT('Ctrl Pts',(8.59489616871569,-68.4367511126203,4.96226561664425));
#39274=CARTESIAN_POINT('Ctrl Pts',(11.4598615582757,-68.2617511126203,-2.06354052510241E-11));
#39275=CARTESIAN_POINT('Ctrl Pts',(8.59489616869782,-68.0867511126203,-4.9622656166752));
#39276=CARTESIAN_POINT('Ctrl Pts',(5.72993077911996,-67.9117511126203,-9.92453123332976));
#39277=CARTESIAN_POINT('Ctrl Pts',(-1.78726082715848E-11,-67.7367511126203,
-9.92453123331945));
#39278=CARTESIAN_POINT('Ctrl Pts',(-5.7299307791557,-67.5617511126203,-9.92453123330913));
#39279=CARTESIAN_POINT('Ctrl Pts',(-8.59489616871569,-67.3867511126203,
-4.96226561664425));
#39280=CARTESIAN_POINT('Ctrl Pts',(-11.4598615582757,-67.2117511126203,
2.06368086793017E-11));
#39281=CARTESIAN_POINT('Ctrl Pts',(-8.59489616869782,-67.0367511126203,
4.9622656166752));
#39282=CARTESIAN_POINT('Ctrl Pts',(-5.72993077911996,-66.8617511126203,
9.92453123332977));
#39283=CARTESIAN_POINT('Ctrl Pts',(1.7871392867044E-11,-66.6867511126203,
9.92453123331945));
#39284=CARTESIAN_POINT('Ctrl Pts',(5.7299307791557,-66.5117511126203,9.92453123330913));
#39285=CARTESIAN_POINT('Ctrl Pts',(8.59489616871569,-66.3367511126203,4.96226561664425));
#39286=CARTESIAN_POINT('Ctrl Pts',(11.4598615582757,-66.1617511126203,-2.06354052510241E-11));
#39287=CARTESIAN_POINT('Ctrl Pts',(8.59489616869782,-65.9867511126203,-4.9622656166752));
#39288=CARTESIAN_POINT('Ctrl Pts',(5.72993077911996,-65.8117511126203,-9.92453123332976));
#39289=CARTESIAN_POINT('Ctrl Pts',(-1.78726082715848E-11,-65.6367511126203,
-9.92453123331945));
#39290=CARTESIAN_POINT('Ctrl Pts',(-5.7299307791557,-65.4617511126203,-9.92453123330913));
#39291=CARTESIAN_POINT('Ctrl Pts',(-8.59489616871569,-65.2867511126203,
-4.96226561664425));
#39292=CARTESIAN_POINT('Ctrl Pts',(-11.4598615582757,-65.1117511126203,
2.06368086793017E-11));
#39293=CARTESIAN_POINT('Ctrl Pts',(-8.59489616869782,-64.9367511126203,
4.9622656166752));
#39294=CARTESIAN_POINT('Ctrl Pts',(-5.72993077911996,-64.7617511126203,
9.92453123332977));
#39295=CARTESIAN_POINT('Ctrl Pts',(1.7871392867044E-11,-64.5867511126203,
9.92453123331945));
#39296=CARTESIAN_POINT('Ctrl Pts',(5.7299307791557,-64.4117511126203,9.92453123330913));
#39297=CARTESIAN_POINT('Ctrl Pts',(8.59489616871569,-64.2367511126203,4.96226561664425));
#39298=CARTESIAN_POINT('Ctrl Pts',(11.4598615582757,-64.0617511126203,-2.06354052510241E-11));
#39299=CARTESIAN_POINT('Ctrl Pts',(8.59489616869782,-63.8867511126203,-4.9622656166752));
#39300=CARTESIAN_POINT('Ctrl Pts',(5.72993077911996,-63.7117511126203,-9.92453123332976));
#39301=CARTESIAN_POINT('Ctrl Pts',(-1.78726082715848E-11,-63.5367511126203,
-9.92453123331945));
#39302=CARTESIAN_POINT('Ctrl Pts',(-5.7299307791557,-63.3617511126203,-9.92453123330913));
#39303=CARTESIAN_POINT('Ctrl Pts',(-8.59489616871569,-63.1867511126203,
-4.96226561664425));
#39304=CARTESIAN_POINT('Ctrl Pts',(-11.4598615582757,-63.0117511126203,
2.06368086793017E-11));
#39305=CARTESIAN_POINT('Ctrl Pts',(-8.59489616869782,-62.8367511126203,
4.9622656166752));
#39306=CARTESIAN_POINT('Ctrl Pts',(-5.72993077911996,-62.6617511126203,
9.92453123332977));
#39307=CARTESIAN_POINT('Ctrl Pts',(1.7871392867044E-11,-62.4867511126203,
9.92453123331945));
#39308=CARTESIAN_POINT('Ctrl Pts',(5.7299307791557,-62.3117511126203,9.92453123330913));
#39309=CARTESIAN_POINT('Ctrl Pts',(8.59489616871569,-62.1367511126203,4.96226561664425));
#39310=CARTESIAN_POINT('Ctrl Pts',(11.4598615582757,-61.9617511126203,-2.06354052510241E-11));
#39311=CARTESIAN_POINT('Ctrl Pts',(8.59489616869782,-61.7867511126203,-4.9622656166752));
#39312=CARTESIAN_POINT('Ctrl Pts',(5.72993077911996,-61.6117511126203,-9.92453123332976));
#39313=CARTESIAN_POINT('Ctrl Pts',(-1.78726082715848E-11,-61.4367511126203,
-9.92453123331945));
#39314=CARTESIAN_POINT('Ctrl Pts',(-5.7299307791557,-61.2617511126203,-9.92453123330913));
#39315=CARTESIAN_POINT('Ctrl Pts',(-8.59489616871569,-61.0867511126203,
-4.96226561664425));
#39316=CARTESIAN_POINT('Ctrl Pts',(-11.4598615582757,-60.9117511126203,
2.06368086793017E-11));
#39317=CARTESIAN_POINT('Ctrl Pts',(-8.59489616869782,-60.7367511126203,
4.9622656166752));
#39318=CARTESIAN_POINT('Ctrl Pts',(-5.72993077911996,-60.5617511126203,
9.92453123332977));
#39319=CARTESIAN_POINT('Ctrl Pts',(1.7871392867044E-11,-60.3867511126203,
9.92453123331945));
#39320=CARTESIAN_POINT('Ctrl Pts',(5.7299307791557,-60.2117511126203,9.92453123330913));
#39321=CARTESIAN_POINT('Ctrl Pts',(8.59489616871569,-60.0367511126203,4.96226561664425));
#39322=CARTESIAN_POINT('Ctrl Pts',(11.4598615582757,-59.8617511126203,-2.06354052510241E-11));
#39323=CARTESIAN_POINT('Ctrl Pts',(8.59489616869782,-59.6867511126203,-4.9622656166752));
#39324=CARTESIAN_POINT('Ctrl Pts',(5.72993077911996,-59.5117511126203,-9.92453123332976));
#39325=CARTESIAN_POINT('Ctrl Pts',(-1.78726082715848E-11,-59.3367511126203,
-9.92453123331945));
#39326=CARTESIAN_POINT('Ctrl Pts',(-5.7299307791557,-59.1617511126203,-9.92453123330913));
#39327=CARTESIAN_POINT('Ctrl Pts',(-8.59489616871569,-58.9867511126203,
-4.96226561664425));
#39328=CARTESIAN_POINT('Ctrl Pts',(-11.4598615582757,-58.8117511126203,
2.06368086793017E-11));
#39329=CARTESIAN_POINT('Ctrl Pts',(-8.59489616869782,-58.6367511126203,
4.9622656166752));
#39330=CARTESIAN_POINT('Ctrl Pts',(-5.72993077911996,-58.4617511126203,
9.92453123332977));
#39331=CARTESIAN_POINT('Ctrl Pts',(1.7871392867044E-11,-58.2867511126203,
9.92453123331945));
#39332=CARTESIAN_POINT('Ctrl Pts',(5.7299307791557,-58.1117511126203,9.92453123330913));
#39333=CARTESIAN_POINT('Ctrl Pts',(8.59489616871569,-57.9367511126203,4.96226561664425));
#39334=CARTESIAN_POINT('Ctrl Pts',(11.4598615582757,-57.7617511126203,-2.06354052510241E-11));
#39335=CARTESIAN_POINT('Ctrl Pts',(8.59489616869782,-57.5867511126203,-4.9622656166752));
#39336=CARTESIAN_POINT('Ctrl Pts',(5.72993077911996,-57.4117511126203,-9.92453123332976));
#39337=CARTESIAN_POINT('Ctrl Pts',(-1.78726082715848E-11,-57.2367511126203,
-9.92453123331945));
#39338=CARTESIAN_POINT('Ctrl Pts',(-5.7299307791557,-57.0617511126203,-9.92453123330913));
#39339=CARTESIAN_POINT('Ctrl Pts',(-8.59489616871569,-56.8867511126203,
-4.96226561664425));
#39340=CARTESIAN_POINT('Ctrl Pts',(-11.4598615582757,-56.7117511126203,
2.06368086793017E-11));
#39341=CARTESIAN_POINT('Ctrl Pts',(-8.59489616869782,-56.5367511126203,
4.9622656166752));
#39342=CARTESIAN_POINT('Ctrl Pts',(-5.72993077911996,-56.3617511126203,
9.92453123332977));
#39343=CARTESIAN_POINT('Ctrl Pts',(1.7871392867044E-11,-56.1867511126203,
9.92453123331945));
#39344=CARTESIAN_POINT('Ctrl Pts',(5.7299307791557,-56.0117511126203,9.92453123330913));
#39345=CARTESIAN_POINT('Ctrl Pts',(8.59489616871569,-55.8367511126203,4.96226561664425));
#39346=CARTESIAN_POINT('Ctrl Pts',(11.4598615582757,-55.6617511126203,-2.06354052510241E-11));
#39347=CARTESIAN_POINT('Ctrl Pts',(8.59489616869782,-55.4867511126203,-4.9622656166752));
#39348=CARTESIAN_POINT('Ctrl Pts',(5.72993077911996,-55.3117511126203,-9.92453123332976));
#39349=CARTESIAN_POINT('Ctrl Pts',(-1.78726082715848E-11,-55.1367511126203,
-9.92453123331945));
#39350=CARTESIAN_POINT('Ctrl Pts',(-5.7299307791557,-54.9617511126203,-9.92453123330913));
#39351=CARTESIAN_POINT('Ctrl Pts',(-8.59489616871569,-54.7867511126203,
-4.96226561664425));
#39352=CARTESIAN_POINT('Ctrl Pts',(-11.4598615582757,-54.6117511126203,
2.06368086793017E-11));
#39353=CARTESIAN_POINT('Ctrl Pts',(-8.59489616869782,-54.4367511126203,
4.9622656166752));
#39354=CARTESIAN_POINT('Ctrl Pts',(-5.72993077911996,-54.2617511126203,
9.92453123332977));
#39355=CARTESIAN_POINT('Ctrl Pts',(1.7871392867044E-11,-54.0867511126203,
9.92453123331945));
#39356=CARTESIAN_POINT('Ctrl Pts',(5.7299307791557,-53.9117511126203,9.92453123330913));
#39357=CARTESIAN_POINT('Ctrl Pts',(8.59489616871569,-53.7367511126203,4.96226561664425));
#39358=CARTESIAN_POINT('Ctrl Pts',(11.4598615582757,-53.5617511126203,-2.06354052510241E-11));
#39359=CARTESIAN_POINT('Ctrl Pts',(8.59489616869782,-53.3867511126203,-4.9622656166752));
#39360=CARTESIAN_POINT('Ctrl Pts',(5.72993077911996,-53.2117511126203,-9.92453123332976));
#39361=CARTESIAN_POINT('Ctrl Pts',(-1.78726082715848E-11,-53.0367511126203,
-9.92453123331945));
#39362=CARTESIAN_POINT('Ctrl Pts',(-5.7299307791557,-52.8617511126203,-9.92453123330913));
#39363=CARTESIAN_POINT('Ctrl Pts',(-8.59489616871569,-52.6867511126203,
-4.96226561664425));
#39364=CARTESIAN_POINT('Ctrl Pts',(-11.4598615582757,-52.5117511126203,
2.06368086793017E-11));
#39365=CARTESIAN_POINT('Ctrl Pts',(-8.59489616869782,-52.3367511126203,
4.9622656166752));
#39366=CARTESIAN_POINT('Ctrl Pts',(-5.72993077911996,-52.1617511126203,
9.92453123332977));
#39367=CARTESIAN_POINT('Ctrl Pts',(1.7871392867044E-11,-51.9867511126203,
9.92453123331945));
#39368=CARTESIAN_POINT('Ctrl Pts',(5.7299307791557,-51.8117511126203,9.92453123330913));
#39369=CARTESIAN_POINT('Ctrl Pts',(8.59489616871569,-51.6367511126203,4.96226561664425));
#39370=CARTESIAN_POINT('Ctrl Pts',(11.4598615582757,-51.4617511126203,-2.06354052510241E-11));
#39371=CARTESIAN_POINT('Ctrl Pts',(8.59489616869782,-51.2867511126203,-4.9622656166752));
#39372=CARTESIAN_POINT('Ctrl Pts',(5.72993077911996,-51.1117511126203,-9.92453123332976));
#39373=CARTESIAN_POINT('Ctrl Pts',(-1.78726082715848E-11,-50.9367511126203,
-9.92453123331945));
#39374=CARTESIAN_POINT('Ctrl Pts',(-5.7299307791557,-50.7617511126203,-9.92453123330913));
#39375=CARTESIAN_POINT('Ctrl Pts',(-8.59489616871569,-50.5867511126203,
-4.96226561664425));
#39376=CARTESIAN_POINT('Ctrl Pts',(-11.4598615582757,-50.4117511126203,
2.06368086793017E-11));
#39377=CARTESIAN_POINT('Ctrl Pts',(-8.59489616869782,-50.2367511126203,
4.9622656166752));
#39378=CARTESIAN_POINT('Ctrl Pts',(-5.72993077911996,-50.0617511126203,
9.92453123332977));
#39379=CARTESIAN_POINT('Ctrl Pts',(1.7871392867044E-11,-49.8867511126203,
9.92453123331945));
#39380=CARTESIAN_POINT('Ctrl Pts',(5.7299307791557,-49.7117511126203,9.92453123330913));
#39381=CARTESIAN_POINT('Ctrl Pts',(8.59489616871569,-49.5367511126204,4.96226561664425));
#39382=CARTESIAN_POINT('Ctrl Pts',(11.4598615582757,-49.3617511126203,-2.06354052510241E-11));
#39383=CARTESIAN_POINT('Ctrl Pts',(8.59489616869782,-49.1867511126203,-4.9622656166752));
#39384=CARTESIAN_POINT('Ctrl Pts',(5.72993077911996,-49.0117511126203,-9.92453123332976));
#39385=CARTESIAN_POINT('Ctrl Pts',(-1.78726082715848E-11,-48.8367511126203,
-9.92453123331945));
#39386=CARTESIAN_POINT('Ctrl Pts',(-5.7299307791557,-48.6617511126203,-9.92453123330913));
#39387=CARTESIAN_POINT('Ctrl Pts',(-8.59489616871569,-48.4867511126203,
-4.96226561664425));
#39388=CARTESIAN_POINT('Ctrl Pts',(-11.4598615582757,-48.3117511126203,
2.06368086793017E-11));
#39389=CARTESIAN_POINT('Ctrl Pts',(-8.59489616869782,-48.1367511126203,
4.9622656166752));
#39390=CARTESIAN_POINT('Ctrl Pts',(-5.72993077911996,-47.9617511126203,
9.92453123332977));
#39391=CARTESIAN_POINT('Ctrl Pts',(1.7871392867044E-11,-47.7867511126204,
9.92453123331945));
#39392=CARTESIAN_POINT('Ctrl Pts',(5.7299307791557,-47.6117511126203,9.92453123330913));
#39393=CARTESIAN_POINT('Ctrl Pts',(8.59489616871569,-47.4367511126203,4.96226561664425));
#39394=CARTESIAN_POINT('Ctrl Pts',(11.4598615582757,-47.2617511126203,-2.06354052510241E-11));
#39395=CARTESIAN_POINT('Ctrl Pts',(8.59489616869782,-47.0867511126203,-4.9622656166752));
#39396=CARTESIAN_POINT('Ctrl Pts',(5.72993077911996,-46.9117511126203,-9.92453123332976));
#39397=CARTESIAN_POINT('Ctrl Pts',(-1.78726082715848E-11,-46.7367511126204,
-9.92453123331945));
#39398=CARTESIAN_POINT('Ctrl Pts',(-5.7299307791557,-46.5617511126203,-9.92453123330913));
#39399=CARTESIAN_POINT('Ctrl Pts',(-8.59489616871569,-46.3867511126203,
-4.96226561664425));
#39400=CARTESIAN_POINT('Ctrl Pts',(-11.4598615582757,-46.2117511126204,
2.06368086793017E-11));
#39401=CARTESIAN_POINT('Ctrl Pts',(-8.59489616869782,-46.0367511126203,
4.9622656166752));
#39402=CARTESIAN_POINT('Ctrl Pts',(-5.72993077911996,-45.8617511126203,
9.92453123332977));
#39403=CARTESIAN_POINT('Ctrl Pts',(1.7871392867044E-11,-45.6867511126204,
9.92453123331945));
#39404=CARTESIAN_POINT('Ctrl Pts',(5.7299307791557,-45.5117511126203,9.92453123330913));
#39405=CARTESIAN_POINT('Ctrl Pts',(8.59489616871569,-45.3367511126203,4.96226561664425));
#39406=CARTESIAN_POINT('Ctrl Pts',(11.4598615582757,-45.1617511126204,-2.06354052510241E-11));
#39407=CARTESIAN_POINT('Ctrl Pts',(8.59489616869782,-44.9867511126203,-4.9622656166752));
#39408=CARTESIAN_POINT('Ctrl Pts',(5.72993077911996,-44.8117511126203,-9.92453123332976));
#39409=CARTESIAN_POINT('Ctrl Pts',(-1.78726082715848E-11,-44.6367511126204,
-9.92453123331945));
#39410=CARTESIAN_POINT('Ctrl Pts',(-5.7299307791557,-44.4617511126204,-9.92453123330913));
#39411=CARTESIAN_POINT('Ctrl Pts',(-8.59489616871569,-44.2867511126203,
-4.96226561664425));
#39412=CARTESIAN_POINT('Ctrl Pts',(-11.4598615582757,-44.1117511126203,
2.06368086793017E-11));
#39413=CARTESIAN_POINT('Ctrl Pts',(-8.59489616869782,-43.9367511126204,
4.9622656166752));
#39414=CARTESIAN_POINT('Ctrl Pts',(-5.72993077911996,-43.7617511126204,
9.92453123332977));
#39415=CARTESIAN_POINT('Ctrl Pts',(1.7871392867044E-11,-43.5867511126203,
9.92453123331945));
#39416=CARTESIAN_POINT('Ctrl Pts',(5.7299307791557,-43.4117511126204,9.92453123330913));
#39417=CARTESIAN_POINT('Ctrl Pts',(8.59489616871569,-43.2367511126203,4.96226561664425));
#39418=CARTESIAN_POINT('Ctrl Pts',(11.4598615582757,-43.0617511126203,-2.06354052510241E-11));
#39419=CARTESIAN_POINT('Ctrl Pts',(8.59489616869782,-42.8867511126204,-4.9622656166752));
#39420=CARTESIAN_POINT('Ctrl Pts',(5.72993077911996,-42.7117511126203,-9.92453123332976));
#39421=CARTESIAN_POINT('Ctrl Pts',(-1.78726082715848E-11,-42.5367511126203,
-9.92453123331945));
#39422=CARTESIAN_POINT('Ctrl Pts',(-0.219644606349529,-212.63,-9.92210040505701));
#39423=CARTESIAN_POINT('Ctrl Pts',(-1.4533920550627,-212.63,-9.8213661461777));
#39424=CARTESIAN_POINT('Ctrl Pts',(-2.65597646823175,-212.63,-9.48288190087395));
#39425=CARTESIAN_POINT('Ctrl Pts',(-4.86098942222034,-212.63,-8.36949832183372));
#39426=CARTESIAN_POINT('Ctrl Pts',(-5.8434616897038,-212.63,-7.60704909264757));
#39427=CARTESIAN_POINT('Ctrl Pts',(-7.32939714963465,-212.63,-5.90751715922259));
#39428=CARTESIAN_POINT('Ctrl Pts',(-7.99853353868902,-212.63,-4.89381432117256));
#39429=CARTESIAN_POINT('Ctrl Pts',(-8.80359152553002,-212.63,-2.62789349339889));
#39430=CARTESIAN_POINT('Ctrl Pts',(-8.97717635487367,-212.63,-1.54602428959771));
#39431=CARTESIAN_POINT('Ctrl Pts',(-8.92442457723671,-212.63,0.700721770435771));
#39432=CARTESIAN_POINT('Ctrl Pts',(-8.67060378400234,-212.63,1.84439401565503));
#39433=CARTESIAN_POINT('Ctrl Pts',(-7.91777274084501,-212.63,3.56131387525748));
#39434=CARTESIAN_POINT('Ctrl Pts',(-7.5464292751167,-212.630000000324,4.19442289602148));
#39435=CARTESIAN_POINT('Ctrl Pts',(-6.6871605411885,-212.630000000324,5.2990234415664));
#39436=CARTESIAN_POINT('Ctrl Pts',(-6.20599255820334,-212.63,5.78118301177607));
#39437=CARTESIAN_POINT('Ctrl Pts',(-5.67113674141197,-212.63,6.19885209091273));
#39438=CARTESIAN_POINT('Origin',(0.,-212.63,9.93750000000001));
#39439=CARTESIAN_POINT('Origin',(-10.8677182860469,-15.875,-3.00462919747432E-15));
#39440=CARTESIAN_POINT('',(-10.8677182860469,-15.875,-6.27448007792623));
#39441=CARTESIAN_POINT('',(-10.8677182860469,-0.848960155852393,-6.27448007792623));
#39442=CARTESIAN_POINT('',(-10.8677182860469,-15.875,-6.27448007792623));
#39443=CARTESIAN_POINT('',(-10.8677182860469,-15.875,6.27448007792622));
#39444=CARTESIAN_POINT('',(-10.8677182860469,-15.875,-3.00462919747432E-15));
#39445=CARTESIAN_POINT('',(-10.8677182860469,-0.848960155852389,6.27448007792622));
#39446=CARTESIAN_POINT('',(-10.8677182860469,-15.875,6.27448007792622));
#39447=CARTESIAN_POINT('',(-10.8677182860469,0.,4.33390115890082));
#39448=CARTESIAN_POINT('Ctrl Pts',(-10.8677182860469,4.31956443403523E-15,
4.33390115890082));
#39449=CARTESIAN_POINT('Ctrl Pts',(-10.8677182860469,-0.34683042785844,
5.27022062193468));
#39450=CARTESIAN_POINT('Ctrl Pts',(-10.8677182860469,-0.848960155837252,
6.27448007789594));
#39451=CARTESIAN_POINT('',(-10.8677182860469,0.,-4.33390115890083));
#39452=CARTESIAN_POINT('',(-10.8677182860469,0.,-3.00462919747432E-15));
#39453=CARTESIAN_POINT('Ctrl Pts',(-10.8677182860469,-0.84896015583725,
-6.27448007789595));
#39454=CARTESIAN_POINT('Ctrl Pts',(-10.8677182860469,-0.346830427858437,
-5.27022062193468));
#39455=CARTESIAN_POINT('Ctrl Pts',(-10.8677182860469,6.60639266381858E-15,
-4.33390115890082));
#39456=CARTESIAN_POINT('Origin',(-5.43385914302348,-15.875,9.41172011688933));
#39457=CARTESIAN_POINT('',(-6.07153216591882E-15,-15.875,12.5489601558524));
#39458=CARTESIAN_POINT('',(-5.43385914302348,-15.875,9.41172011688933));
#39459=CARTESIAN_POINT('',(-6.07153216591882E-15,-0.848960155852391,12.5489601558524));
#39460=CARTESIAN_POINT('',(-6.07153216591882E-15,-15.875,12.5489601558524));
#39461=CARTESIAN_POINT('',(-1.68059064192455,0.,11.5786706963397));
#39462=CARTESIAN_POINT('Ctrl Pts',(-1.68059064192455,2.28682822978336E-15,
11.5786706963397));
#39463=CARTESIAN_POINT('Ctrl Pts',(-0.869714200879427,-0.34683042785844,
12.0468304278567));
#39464=CARTESIAN_POINT('Ctrl Pts',(-2.62300655575992E-11,-0.848960155837252,
12.5489601558373));
#39465=CARTESIAN_POINT('',(-9.18712764412241,0.,7.24476953743892));
#39466=CARTESIAN_POINT('',(-5.43385914302348,0.,9.41172011688933));
#39467=CARTESIAN_POINT('Ctrl Pts',(-10.8677182860207,-0.848960155837241,
6.27448007794137));
#39468=CARTESIAN_POINT('Ctrl Pts',(-9.99800408516752,-0.346830427858434,
6.776609805922));
#39469=CARTESIAN_POINT('Ctrl Pts',(-9.1871276441224,4.82774848509819E-15,
7.24476953743893));
#39470=CARTESIAN_POINT('Origin',(5.43385914302347,-15.875,9.41172011688934));
#39471=CARTESIAN_POINT('',(10.8677182860469,-15.875,6.27448007792623));
#39472=CARTESIAN_POINT('',(5.43385914302347,-15.875,9.41172011688934));
#39473=CARTESIAN_POINT('',(10.8677182860469,-0.848960155852389,6.27448007792623));
#39474=CARTESIAN_POINT('',(10.8677182860469,-15.875,6.27448007792623));
#39475=CARTESIAN_POINT('',(9.1871276441224,0.,7.24476953743893));
#39476=CARTESIAN_POINT('Ctrl Pts',(9.1871276441224,0.,7.24476953743893));
#39477=CARTESIAN_POINT('Ctrl Pts',(9.99800408516752,-0.346830427858443,
6.776609805922));
#39478=CARTESIAN_POINT('Ctrl Pts',(10.8677182860207,-0.848960155837255,
6.27448007794137));
#39479=CARTESIAN_POINT('',(1.68059064192454,0.,11.5786706963397));
#39480=CARTESIAN_POINT('',(5.43385914302347,0.,9.41172011688934));
#39481=CARTESIAN_POINT('Ctrl Pts',(2.6228483654321E-11,-0.848960155837241,
12.5489601558373));
#39482=CARTESIAN_POINT('Ctrl Pts',(0.869714200879426,-0.34683042785843,
12.0468304278567));
#39483=CARTESIAN_POINT('Ctrl Pts',(1.68059064192455,1.11800491233853E-14,
11.5786706963397));
#39484=CARTESIAN_POINT('Origin',(10.8677182860469,-15.875,0.));
#39485=CARTESIAN_POINT('',(10.8677182860469,-15.875,-6.27448007792623));
#39486=CARTESIAN_POINT('',(10.8677182860469,-15.875,0.));
#39487=CARTESIAN_POINT('',(10.8677182860469,-0.848960155852391,-6.27448007792623));
#39488=CARTESIAN_POINT('',(10.8677182860469,-15.875,-6.27448007792623));
#39489=CARTESIAN_POINT('',(10.8677182860469,0.,-4.33390115890083));
#39490=CARTESIAN_POINT('Ctrl Pts',(10.8677182860469,3.0491043063778E-15,
-4.33390115890084));
#39491=CARTESIAN_POINT('Ctrl Pts',(10.8677182860469,-0.346830427858442,
-5.27022062193469));
#39492=CARTESIAN_POINT('Ctrl Pts',(10.8677182860469,-0.848960155837254,
-6.27448007789596));
#39493=CARTESIAN_POINT('',(10.8677182860469,0.,4.33390115890083));
#39494=CARTESIAN_POINT('',(10.8677182860469,0.,0.));
#39495=CARTESIAN_POINT('Ctrl Pts',(10.8677182860469,-0.848960155837236,
6.27448007789593));
#39496=CARTESIAN_POINT('Ctrl Pts',(10.8677182860469,-0.346830427858437,
5.27022062193468));
#39497=CARTESIAN_POINT('Ctrl Pts',(10.8677182860469,1.27046012765742E-15,
4.33390115890084));
#39498=CARTESIAN_POINT('Origin',(5.43385914302348,-15.875,-9.41172011688934));
#39499=CARTESIAN_POINT('',(3.46944695195361E-15,-15.875,-12.5489601558525));
#39500=CARTESIAN_POINT('',(5.43385914302348,-15.875,-9.41172011688934));
#39501=CARTESIAN_POINT('',(3.46944695195361E-15,-15.875,-12.5489601558525));
#39502=CARTESIAN_POINT('',(9.18712764412239,0.,-7.24476953743894));
#39503=CARTESIAN_POINT('',(5.43385914302348,0.,-9.41172011688934));
#39504=CARTESIAN_POINT('Ctrl Pts',(10.8677182860207,-0.848960155837252,
-6.27448007794137));
#39505=CARTESIAN_POINT('Ctrl Pts',(9.99800408516752,-0.346830427858437,
-6.77660980592201));
#39506=CARTESIAN_POINT('Ctrl Pts',(9.18712764412239,6.60639266381857E-15,
-7.24476953743894));
#39507=CARTESIAN_POINT('Origin',(-5.43385914302347,-15.875,-9.41172011688934));
#39508=CARTESIAN_POINT('',(-5.43385914302347,-15.875,-9.41172011688934));
#39509=CARTESIAN_POINT('',(-9.18712764412239,0.,-7.24476953743893));
#39510=CARTESIAN_POINT('Ctrl Pts',(-9.18712764412239,2.54092025531484E-15,
-7.24476953743893));
#39511=CARTESIAN_POINT('Ctrl Pts',(-9.99800408516753,-0.346830427858443,
-6.776609805922));
#39512=CARTESIAN_POINT('Ctrl Pts',(-10.8677182860207,-0.848960155837259,
-6.27448007794136));
#39513=CARTESIAN_POINT('',(-5.43385914302347,0.,-9.41172011688934));
#39514=CARTESIAN_POINT('Origin',(0.,-15.875,0.));
#39515=CARTESIAN_POINT('Origin',(0.,-0.999999999999945,0.));
#39516=CARTESIAN_POINT('Origin',(0.,0.,0.));
#39517=CARTESIAN_POINT('Origin',(0.,-0.999999999999945,0.));
#39518=CARTESIAN_POINT('Origin',(0.,0.,0.));
#39519=CARTESIAN_POINT('Origin',(0.,-0.999999999999945,0.));
#39520=CARTESIAN_POINT('Origin',(0.,0.,0.));
#39521=CARTESIAN_POINT('Origin',(0.,-0.999999999999945,0.));
#39522=CARTESIAN_POINT('Origin',(0.,0.,0.));
#39523=CARTESIAN_POINT('Origin',(0.,-0.999999999999945,0.));
#39524=CARTESIAN_POINT('Origin',(0.,0.,0.));
#39525=CARTESIAN_POINT('Origin',(0.,0.,0.));
#39526=CARTESIAN_POINT('Ctrl Pts',(-0.194315056459259,-26.7212227391133,
-12.1981274139594));
#39527=CARTESIAN_POINT('Ctrl Pts',(-0.203067890482931,-26.7208823204558,
-12.6983912923613));
#39528=CARTESIAN_POINT('Ctrl Pts',(-0.222506667109496,-27.2208450130247,
-12.6980506686299));
#39529=CARTESIAN_POINT('Ctrl Pts',(0.134166779161007,-26.7339981836376,
-12.2044589641634));
#39530=CARTESIAN_POINT('Ctrl Pts',(0.139777617995481,-26.7347920529262,
-12.7038236374003));
#39531=CARTESIAN_POINT('Ctrl Pts',(0.153629648332412,-27.2348979165139,
-12.7046416675251));
#39532=CARTESIAN_POINT('Ctrl Pts',(0.472996743962122,-26.7137256552718,
-12.1943004586851));
#39533=CARTESIAN_POINT('Ctrl Pts',(0.496088949698769,-26.7124000235208,
-12.6949661157068));
#39534=CARTESIAN_POINT('Ctrl Pts',(0.541620041925868,-27.2125982196052,
-12.6940668718406));
#39535=CARTESIAN_POINT('Ctrl Pts',(1.13102669670067,-26.6067914943918,-12.1418208766917));
#39536=CARTESIAN_POINT('Ctrl Pts',(1.18251789112393,-26.5959733556708,-12.6500253820366));
#39537=CARTESIAN_POINT('Ctrl Pts',(1.29511827496423,-27.0949706450248,-12.6394364854779));
#39538=CARTESIAN_POINT('Ctrl Pts',(1.44820857041315,-26.5218354596063,-12.1003567529811));
#39539=CARTESIAN_POINT('Ctrl Pts',(1.51413351942913,-26.5025539703757,-12.6142304394117));
#39540=CARTESIAN_POINT('Ctrl Pts',(1.65831751887342,-27.0015190056013,-12.596273014076));
#39541=CARTESIAN_POINT('Ctrl Pts',(2.06065319481642,-26.2923457172244,-11.9924294251706));
#39542=CARTESIAN_POINT('Ctrl Pts',(2.1480929495222,-26.2540473941778,-12.5230572090411));
#39543=CARTESIAN_POINT('Ctrl Pts',(2.35961681393454,-26.7490802889125,-12.483922433672));
#39544=CARTESIAN_POINT('Ctrl Pts',(2.35854389520533,-26.145712314138,-11.9250475278437));
#39545=CARTESIAN_POINT('Ctrl Pts',(2.4554509163846,-26.09432187406,-12.4661578446707));
#39546=CARTESIAN_POINT('Ctrl Pts',(2.70072608321809,-26.5877835449747,-12.4137789851734));
#39547=CARTESIAN_POINT('Ctrl Pts',(2.9104768853475,-25.803547654477,-11.776582758216));
#39548=CARTESIAN_POINT('Ctrl Pts',(3.01814234426553,-25.727851383016,-12.3439902212264));
#39549=CARTESIAN_POINT('Ctrl Pts',(3.33273459746412,-26.2114024205019,-12.2592295912986));
#39550=CARTESIAN_POINT('Ctrl Pts',(3.16675759630227,-25.6078668562775,-11.6953386900839));
#39551=CARTESIAN_POINT('Ctrl Pts',(3.27655230794715,-25.5181571512881,-12.2779126330183));
#39552=CARTESIAN_POINT('Ctrl Pts',(3.62619701879906,-25.9961535423151,-12.1746558505725));
#39553=CARTESIAN_POINT('Ctrl Pts',(3.52278337011958,-25.2769360215998,-11.5690410381704));
#39554=CARTESIAN_POINT('Ctrl Pts',(3.62723458607873,-25.1735020601709,-12.1792044217791));
#39555=CARTESIAN_POINT('Ctrl Pts',(4.03387571115309,-25.6321296235549,-12.0431820637955));
#39556=CARTESIAN_POINT('Ctrl Pts',(3.63691595191385,-25.1599641836089,-11.5260929344709));
#39557=CARTESIAN_POINT('Ctrl Pts',(3.73963755328883,-25.0511426623102,-12.1457738319626));
#39558=CARTESIAN_POINT('Ctrl Pts',(4.16456687282794,-25.5034606017804,-11.9984737931225));
#39559=CARTESIAN_POINT('Ctrl Pts',(3.85121707642186,-24.9178456922059,-11.4415520283336));
#39560=CARTESIAN_POINT('Ctrl Pts',(3.94898113658373,-24.8000160592407,-12.0809829287729));
#39561=CARTESIAN_POINT('Ctrl Pts',(4.40995922601222,-25.2371302616159,-11.9104680943871));
#39562=CARTESIAN_POINT('Ctrl Pts',(3.95198070070556,-24.7922056825208,-11.3997592507804));
#39563=CARTESIAN_POINT('Ctrl Pts',(4.04625813149204,-24.6705623727243,-12.0494916609173));
#39564=CARTESIAN_POINT('Ctrl Pts',(4.52534183541223,-25.0989262507882,-11.8669624993707));
#39565=CARTESIAN_POINT('Ctrl Pts',(4.23558744018011,-24.401454308808,-11.2775109794014));
#39566=CARTESIAN_POINT('Ctrl Pts',(4.3203397283013,-24.2676859595634,-11.9580183198169));
#39567=CARTESIAN_POINT('Ctrl Pts',(4.85009479778453,-24.6690997396581,-11.7397040511128));
#39568=CARTESIAN_POINT('Ctrl Pts',(4.40029129520591,-24.1219950623208,-11.1999546753906));
#39569=CARTESIAN_POINT('Ctrl Pts',(4.47234649383105,-23.9871950107587,-11.9032777424555));
#39570=CARTESIAN_POINT('Ctrl Pts',(5.03869421244281,-24.3616945682431,-11.6589692124176));
#39571=CARTESIAN_POINT('Ctrl Pts',(4.67633642519072,-23.5250073471767,-11.0637813849082));
#39572=CARTESIAN_POINT('Ctrl Pts',(4.72346035897912,-23.401295578245,-11.8103646186347));
#39573=CARTESIAN_POINT('Ctrl Pts',(5.35478851329005,-23.7050080822041,-11.5172150470738));
#39574=CARTESIAN_POINT('Ctrl Pts',(4.78350043752076,-23.216754789204,-11.007350870447));
#39575=CARTESIAN_POINT('Ctrl Pts',(4.81587476821909,-23.1073726626684,-11.7745863820089));
#39576=CARTESIAN_POINT('Ctrl Pts',(5.47750009197968,-23.3659302682378,-11.458471808437));
#39577=CARTESIAN_POINT('Ctrl Pts',(4.89876860580401,-22.7393314761495,-10.9455338368082));
#39578=CARTESIAN_POINT('Ctrl Pts',(4.91470009013209,-22.6607732404412,-11.7361393743978));
#39579=CARTESIAN_POINT('Ctrl Pts',(5.6094915916466,-22.8407646237077,-11.3941212887981));
#39580=CARTESIAN_POINT('Ctrl Pts',(4.92955208184883,-22.5776667539846,-10.9287329128092));
#39581=CARTESIAN_POINT('Ctrl Pts',(4.94074128439299,-22.5103984492741,-11.725920546492));
#39582=CARTESIAN_POINT('Ctrl Pts',(5.64474119604575,-22.6629334294602,-11.3766318028864));
#39583=CARTESIAN_POINT('Ctrl Pts',(4.97523170289568,-22.2490170068924,-10.9036572997793));
#39584=CARTESIAN_POINT('Ctrl Pts',(4.97935760333758,-22.2060010603353,-11.7107367920172));
#39585=CARTESIAN_POINT('Ctrl Pts',(5.69704810501006,-22.3014187075044,-11.350528500382));
#39586=CARTESIAN_POINT('Ctrl Pts',(4.9900614685414,-22.0812569558744,-10.8954209365004));
#39587=CARTESIAN_POINT('Ctrl Pts',(4.99169258536863,-22.052002659175,-11.7058637040127));
#39588=CARTESIAN_POINT('Ctrl Pts',(5.71402940255624,-22.1168826514477,-11.3419545814996));
#39589=CARTESIAN_POINT('Ctrl Pts',(5.00902637313877,-21.5829271070114,-10.8848943478805));
#39590=CARTESIAN_POINT('Ctrl Pts',(5.0075744573728,-21.5937822825219,-11.6995920372639));
#39591=CARTESIAN_POINT('Ctrl Pts',(5.73574577388715,-21.5687198177408,-11.3309965751315));
#39592=CARTESIAN_POINT('Ctrl Pts',(4.98870840505789,-21.2534958170338,-10.8963611248835));
#39593=CARTESIAN_POINT('Ctrl Pts',(4.99120040430745,-21.2953972536494,-11.7061066151783));
#39594=CARTESIAN_POINT('Ctrl Pts',(5.71248003454301,-21.206345398664,-11.3429333016361));
#39595=CARTESIAN_POINT('Ctrl Pts',(4.90945823057519,-20.7634378238772,-10.9396841355917));
#39596=CARTESIAN_POINT('Ctrl Pts',(4.92366751892991,-20.838223666219,-11.7326137010596));
#39597=CARTESIAN_POINT('Ctrl Pts',(5.62173208850429,-20.6672816063015,-11.3880318463151));
#39598=CARTESIAN_POINT('Ctrl Pts',(4.87455989872081,-20.5998021506003,-10.9586262653569));
#39599=CARTESIAN_POINT('Ctrl Pts',(4.89400424310528,-20.6854463533553,-11.7442263723397));
#39600=CARTESIAN_POINT('Ctrl Pts',(5.58177063740257,-20.4872823658008,-11.4077502922669));
#39601=CARTESIAN_POINT('Ctrl Pts',(4.78945908598975,-20.2798404689652,-11.0039362410179));
#39602=CARTESIAN_POINT('Ctrl Pts',(4.82020327496675,-20.3830544594789,-11.7728329898822));
#39603=CARTESIAN_POINT('Ctrl Pts',(5.48432323279469,-20.1353245157212,-11.4549172348609));
#39604=CARTESIAN_POINT('Ctrl Pts',(4.73937502306188,-20.1234268906168,-11.030240976236));
#39605=CARTESIAN_POINT('Ctrl Pts',(4.77648918248447,-20.2339643104042,-11.789668542258));
#39606=CARTESIAN_POINT('Ctrl Pts',(5.42697287433976,-19.9632695797551,-11.4823000321756));
#39607=CARTESIAN_POINT('Ctrl Pts',(4.56731216496254,-19.6642943627305,-11.1183794655812));
#39608=CARTESIAN_POINT('Ctrl Pts',(4.62447523913058,-19.7943682502535,-11.8473111221715));
#39609=CARTESIAN_POINT('Ctrl Pts',(5.22994679958899,-19.4582237988502,-11.5740507560812));
#39610=CARTESIAN_POINT('Ctrl Pts',(4.4225017548533,-19.3696333894946,-11.1899943284984));
#39611=CARTESIAN_POINT('Ctrl Pts',(4.49417778960582,-19.5042750964007,-11.8958840070277));
#39612=CARTESIAN_POINT('Ctrl Pts',(5.06412700816816,-19.1340967289438,-11.6486006523686));
#39613=CARTESIAN_POINT('Ctrl Pts',(4.07922497844486,-18.8153269570627,-11.3466863829177));
#39614=CARTESIAN_POINT('Ctrl Pts',(4.17144753969082,-18.9460643318112,-12.0086673192177));
#39615=CARTESIAN_POINT('Ctrl Pts',(4.67104696430523,-18.5243596522693,-11.8117145144333));
#39616=CARTESIAN_POINT('Ctrl Pts',(3.88357483934998,-18.5592589877753,-11.4304872091369));
#39617=CARTESIAN_POINT('Ctrl Pts',(3.98456712315329,-18.6823627389427,-12.0711495294318));
#39618=CARTESIAN_POINT('Ctrl Pts',(4.44701151665401,-18.2426848863307,-11.8989497983692));
#39619=CARTESIAN_POINT('Ctrl Pts',(3.44456423424596,-18.08644988691,-11.599515766087));
#39620=CARTESIAN_POINT('Ctrl Pts',(3.55363139810777,-18.190115999482,-12.2017033779511));
#39621=CARTESIAN_POINT('Ctrl Pts',(3.94430838975052,-17.7225948758231,-12.0749057578065));
#39622=CARTESIAN_POINT('Ctrl Pts',(3.19881952916763,-17.8685825627143,-11.6853630222093));
#39623=CARTESIAN_POINT('Ctrl Pts',(3.30880170180714,-17.9587265964904,-12.2701736879534));
#39624=CARTESIAN_POINT('Ctrl Pts',(3.66291055880196,-17.4829408191597,-12.1642713417504));
#39625=CARTESIAN_POINT('Ctrl Pts',(2.67586340966611,-17.4889456042686,-11.8433556306518));
#39626=CARTESIAN_POINT('Ctrl Pts',(2.7799526126078,-17.5545379722142,-12.3984078601019));
#39627=CARTESIAN_POINT('Ctrl Pts',(3.06408293755109,-17.0653401645214,-12.3287390591788));
#39628=CARTESIAN_POINT('Ctrl Pts',(2.39714240324113,-17.3248873383762,-11.916286264565));
#39629=CARTESIAN_POINT('Ctrl Pts',(2.49456444142712,-17.3767916845148,-12.4592374659268));
#39630=CARTESIAN_POINT('Ctrl Pts',(2.74492453899815,-16.8848760712784,-12.4046586511814));
#39631=CARTESIAN_POINT('Ctrl Pts',(1.95126020128702,-17.1185475242902,-12.0108596275047));
#39632=CARTESIAN_POINT('Ctrl Pts',(2.03243224842994,-17.1527631933337,-12.538948153782));
#39633=CARTESIAN_POINT('Ctrl Pts',(2.23435286973199,-16.6579022771869,-12.5031079735321));
#39634=CARTESIAN_POINT('Ctrl Pts',(1.79708542715294,-17.0562076265249,-12.0400265737317));
#39635=CARTESIAN_POINT('Ctrl Pts',(1.87292847323085,-17.0851427079614,-12.5635973650709));
#39636=CARTESIAN_POINT('Ctrl Pts',(2.05781011604666,-16.5893283894317,-12.5334702855318));
#39637=CARTESIAN_POINT('Ctrl Pts',(1.48587265051063,-16.9480427335416,-12.0912569680729));
#39638=CARTESIAN_POINT('Ctrl Pts',(1.55038574292973,-16.9679145460432,-12.6069707100262));
#39639=CARTESIAN_POINT('Ctrl Pts',(1.70144597780252,-16.4703470066414,-12.5868002866746));
#39640=CARTESIAN_POINT('Ctrl Pts',(1.32830296766848,-16.9018752765432,-12.1134730678806));
#39641=CARTESIAN_POINT('Ctrl Pts',(1.38646382234108,-16.9176368740355,-12.6259247675388));
#39642=CARTESIAN_POINT('Ctrl Pts',(1.52101577525149,-16.4195628041692,-12.6099268818699));
#39643=CARTESIAN_POINT('Ctrl Pts',(0.849712379879955,-16.7868148719163,
-12.1692615728115));
#39644=CARTESIAN_POINT('Ctrl Pts',(0.890021886410261,-16.792984727058,-12.6733512894767));
#39645=CARTESIAN_POINT('Ctrl Pts',(0.97299032356098,-16.2929963591646,-12.6680018017417));
#39646=CARTESIAN_POINT('Ctrl Pts',(0.522843528836518,-16.7411087801806,
-12.192015621403));
#39647=CARTESIAN_POINT('Ctrl Pts',(0.546774053144795,-16.7425758435111,
-12.6931350453388));
#39648=CARTESIAN_POINT('Ctrl Pts',(0.598698193236015,-16.2427196426588,
-12.6916884026848));
#39649=CARTESIAN_POINT('Ctrl Pts',(0.187614356002326,-16.7285211545107,
-12.1982543436608));
#39650=CARTESIAN_POINT('Ctrl Pts',(0.196065836120502,-16.7288385017964,
-12.6985003258571));
#39651=CARTESIAN_POINT('Ctrl Pts',(0.214833815848565,-16.2288732699618,
-12.6981828003682));
#39652=CARTESIAN_POINT('Ctrl Pts',(-4.99974790012545,-21.7752089154545,
10.8900436331349));
#39653=CARTESIAN_POINT('Ctrl Pts',(-4.9997892831013,-21.7710880447939,11.7026661900649));
#39654=CARTESIAN_POINT('Ctrl Pts',(-5.7251211610453,-21.780229807,11.3363568967879));
#39655=CARTESIAN_POINT('Ctrl Pts',(-5.00304595984301,-21.4467918007238,
10.888211476959));
#39656=CARTESIAN_POINT('Ctrl Pts',(-5.00254692109715,-21.4695196042577,
11.7015768786492));
#39657=CARTESIAN_POINT('Ctrl Pts',(-5.72889771294517,-21.4189707623668,
11.3344496511539));
#39658=CARTESIAN_POINT('Ctrl Pts',(-4.97288676993301,-21.1079790011279,
10.9051863195259));
#39659=CARTESIAN_POINT('Ctrl Pts',(-4.97816559108657,-21.1617339230278,
11.7112712509762));
#39660=CARTESIAN_POINT('Ctrl Pts',(-5.69436296373837,-21.046276901468,11.3521201845275));
#39661=CARTESIAN_POINT('Ctrl Pts',(-4.8475766924768,-20.4556230070702,10.9732455674719));
#39662=CARTESIAN_POINT('Ctrl Pts',(-4.87122044600907,-20.5529478534329,
11.7531280385312));
#39663=CARTESIAN_POINT('Ctrl Pts',(-5.55087265674237,-20.3286853075499,
11.4229687470194));
#39664=CARTESIAN_POINT('Ctrl Pts',(-4.75402318349561,-20.1421071640224,
11.0233953157927));
#39665=CARTESIAN_POINT('Ctrl Pts',(-4.79168297279574,-20.2572142470778,
11.7841890508463));
#39666=CARTESIAN_POINT('Ctrl Pts',(-5.44374621873778,-19.9838178803991,
11.4751738113353));
#39667=CARTESIAN_POINT('Ctrl Pts',(-4.50822613582157,-19.5381796443928,
11.1476441824275));
#39668=CARTESIAN_POINT('Ctrl Pts',(-4.57102076787078,-19.6706340339177,
11.8671679629395));
#39669=CARTESIAN_POINT('Ctrl Pts',(-5.16228845264427,-19.3194976088576,
11.604514846648));
#39670=CARTESIAN_POINT('Ctrl Pts',(-4.35399453240018,-19.2456108462244,
11.222580760125));
#39671=CARTESIAN_POINT('Ctrl Pts',(-4.43086369345143,-19.3804837094271,
11.918784057563));
#39672=CARTESIAN_POINT('Ctrl Pts',(-4.98568062344723,-18.9976719311581,
11.6825225934331));
#39673=CARTESIAN_POINT('Ctrl Pts',(-3.99822324535597,-18.7052566591967,
11.3816435002527));
#39674=CARTESIAN_POINT('Ctrl Pts',(-4.09403979594845,-18.8333578011231,
12.0345832241545));
#39675=CARTESIAN_POINT('Ctrl Pts',(-4.57829334009813,-18.403282324805,11.8481043005667));
#39676=CARTESIAN_POINT('Ctrl Pts',(-3.79614074972304,-18.4547671323408,
11.4661525699866));
#39677=CARTESIAN_POINT('Ctrl Pts',(-3.89978361880875,-18.5742120955944,
12.0982534904074));
#39678=CARTESIAN_POINT('Ctrl Pts',(-4.34689231755036,-18.1277438450899,
11.9360768542446));
#39679=CARTESIAN_POINT('Ctrl Pts',(-3.4555666172681,-18.1076340724598,11.5934834098038));
#39680=CARTESIAN_POINT('Ctrl Pts',(-3.56063728772652,-18.208019782401,12.1983493706666));
#39681=CARTESIAN_POINT('Ctrl Pts',(-3.95690701991751,-17.7458974799482,
12.0686261731993));
#39682=CARTESIAN_POINT('Ctrl Pts',(-3.33556657674612,-17.9967092756542,
11.6360572166061));
#39683=CARTESIAN_POINT('Ctrl Pts',(-3.44136644280938,-18.091181004224,12.2319898021103));
#39684=CARTESIAN_POINT('Ctrl Pts',(-3.81949713715775,-17.6238802033987,
12.1129448069321));
#39685=CARTESIAN_POINT('Ctrl Pts',(-3.08765794162476,-17.7889455607588,
11.7185578736022));
#39686=CARTESIAN_POINT('Ctrl Pts',(-3.19301676454295,-17.8715401644258,
12.2979092990021));
#39687=CARTESIAN_POINT('Ctrl Pts',(-3.53562143018988,-17.3953401166556,
12.1988266394323));
#39688=CARTESIAN_POINT('Ctrl Pts',(-2.95917839859145,-17.6914812338737,
11.7587096839202));
#39689=CARTESIAN_POINT('Ctrl Pts',(-3.06344399393121,-17.7677610739344,
12.3304098410213));
#39690=CARTESIAN_POINT('Ctrl Pts',(-3.38850182188745,-17.2881293572017,
12.2406240146649));
#39691=CARTESIAN_POINT('Ctrl Pts',(-2.56004783110733,-17.4180060566589,
11.874403875677));
#39692=CARTESIAN_POINT('Ctrl Pts',(-2.66175717787732,-17.4782425461364,
12.424067645299));
#39693=CARTESIAN_POINT('Ctrl Pts',(-2.93146460681647,-16.9873066624433,
12.3610597733481));
#39694=CARTESIAN_POINT('Ctrl Pts',(-2.27486874631425,-17.2602612803891,
11.9454237793291));
#39695=CARTESIAN_POINT('Ctrl Pts',(-2.36897880880302,-17.3070252858775,
12.4835705284405));
#39696=CARTESIAN_POINT('Ctrl Pts',(-2.60491117878045,-16.8137874091111,
12.4349903271314));
#39697=CARTESIAN_POINT('Ctrl Pts',(-1.66829057301287,-16.9999892898167,
12.0659549491969));
#39698=CARTESIAN_POINT('Ctrl Pts',(-1.74288242177667,-17.0257586318796,
12.5848852122335));
#39699=CARTESIAN_POINT('Ctrl Pts',(-1.91032945162938,-16.5274882181152,
12.5604613001046));
#39700=CARTESIAN_POINT('Ctrl Pts',(-1.35602206747909,-16.901197524674,12.1136733746908));
#39701=CARTESIAN_POINT('Ctrl Pts',(-1.41703878619547,-16.917247264823,12.6259413073311));
#39702=CARTESIAN_POINT('Ctrl Pts',(-1.55275641664969,-16.4188172766958,
12.6101353975839));
#39703=CARTESIAN_POINT('Ctrl Pts',(-0.874041288385835,-16.7992494614212,
12.1633518858597));
#39704=CARTESIAN_POINT('Ctrl Pts',(-0.913364126384539,-16.8060095815626,
12.6685169960183));
#39705=CARTESIAN_POINT('Ctrl Pts',(-1.00084891791217,-16.3066744077861,
12.6618499142987));
#39706=CARTESIAN_POINT('Ctrl Pts',(-0.711103423472234,-16.7730315381214,
12.1762593351104));
#39707=CARTESIAN_POINT('Ctrl Pts',(-0.743134712400736,-16.7773731884659,
12.679611525474));
#39708=CARTESIAN_POINT('Ctrl Pts',(-0.814271707084701,-16.2778346913951,
12.6752863566669));
#39709=CARTESIAN_POINT('Ctrl Pts',(-0.380466742863404,-16.7367232651056,
12.1941787863531));
#39710=CARTESIAN_POINT('Ctrl Pts',(-0.397886608443954,-16.7378146965554,
12.6949839945871));
#39711=CARTESIAN_POINT('Ctrl Pts',(-0.435665606334057,-16.2378955921547,
12.6939402123975));
#39712=CARTESIAN_POINT('Ctrl Pts',(-0.212389997256555,-16.726751349885,
12.1991315303899));
#39713=CARTESIAN_POINT('Ctrl Pts',(-0.22198786823178,-16.7269094835482,
12.6992537577252));
#39714=CARTESIAN_POINT('Ctrl Pts',(-0.243203955872194,-16.2269264852237,
12.6990959375268));
#39715=CARTESIAN_POINT('Ctrl Pts',(0.285977783389921,-16.7221395157718,
12.2014184689124));
#39716=CARTESIAN_POINT('Ctrl Pts',(0.298771981497033,-16.7218825451742,
12.701218322749));
#39717=CARTESIAN_POINT('Ctrl Pts',(0.327468002777916,-16.2218534666486,
12.7014766025767));
#39718=CARTESIAN_POINT('Ctrl Pts',(0.61472139864815,-16.7518908218649,12.1865389231491));
#39719=CARTESIAN_POINT('Ctrl Pts',(0.644365017122131,-16.7547284026901,
12.6882557475219));
#39720=CARTESIAN_POINT('Ctrl Pts',(0.703906388566332,-16.2545799035585,
12.6859872398608));
#39721=CARTESIAN_POINT('Ctrl Pts',(1.10267114335561,-16.8452929725738,12.1408822967383));
#39722=CARTESIAN_POINT('Ctrl Pts',(1.15158356010911,-16.8560859875697,12.6493167720793));
#39723=CARTESIAN_POINT('Ctrl Pts',(1.26264884196562,-16.3573222700776,12.6384594399526));
#39724=CARTESIAN_POINT('Ctrl Pts',(1.26533226414711,-16.8849300158631,12.121617968646));
#39725=CARTESIAN_POINT('Ctrl Pts',(1.32111739439795,-16.8993078832869,12.6328274609239));
#39726=CARTESIAN_POINT('Ctrl Pts',(1.44890915812603,-16.4009230179359,12.6184055908425));
#39727=CARTESIAN_POINT('Ctrl Pts',(1.58235492966266,-16.979107453112,12.0764753436775));
#39728=CARTESIAN_POINT('Ctrl Pts',(1.6504058732465,-17.0015359945446,12.5944605703878));
#39729=CARTESIAN_POINT('Ctrl Pts',(1.81192609576926,-16.5045181979368,12.571412857232));
#39730=CARTESIAN_POINT('Ctrl Pts',(1.73719161826021,-17.0336380495884,12.0505998841791));
#39731=CARTESIAN_POINT('Ctrl Pts',(1.81102761429328,-17.0607993356339,12.5724903400979));
#39732=CARTESIAN_POINT('Ctrl Pts',(1.98922679567035,-16.5645018547241,12.5444769290866));
#39733=CARTESIAN_POINT('Ctrl Pts',(2.03985290921885,-17.1570998503607,11.9930699877706));
#39734=CARTESIAN_POINT('Ctrl Pts',(2.12375845988698,-17.1943173681734,12.5240400570731));
#39735=CARTESIAN_POINT('Ctrl Pts',(2.33579878210691,-16.7003098352198,12.4845892490906));
#39736=CARTESIAN_POINT('Ctrl Pts',(2.18767675415801,-17.2260321119876,11.9614136149928));
#39737=CARTESIAN_POINT('Ctrl Pts',(2.27614008230909,-17.2688969498113,12.4974526711999));
#39738=CARTESIAN_POINT('Ctrl Pts',(2.50506920142481,-16.7761353230868,12.4516354848906));
#39739=CARTESIAN_POINT('Ctrl Pts',(2.4764397755925,-17.3782900170458,11.8930970814406));
#39740=CARTESIAN_POINT('Ctrl Pts',(2.57238648290045,-17.4327114608064,12.4406234530185));
#39741=CARTESIAN_POINT('Ctrl Pts',(2.83572652977311,-16.94361901885,12.3805190925443));
#39742=CARTESIAN_POINT('Ctrl Pts',(2.61807236646183,-17.4621017397464,11.8562300451449));
#39743=CARTESIAN_POINT('Ctrl Pts',(2.71713597356284,-17.522827623315,12.4101082654188));
#39744=CARTESIAN_POINT('Ctrl Pts',(2.99790745559855,-17.035811914121,12.3421411132669));
#39745=CARTESIAN_POINT('Ctrl Pts',(3.02646929124701,-17.7316428155805,11.7410636200549));
#39746=CARTESIAN_POINT('Ctrl Pts',(3.13548340049963,-17.8131259362093,12.3150866370692));
#39747=CARTESIAN_POINT('Ctrl Pts',(3.46555540992292,-17.3323070963386,12.2222547506283));
#39748=CARTESIAN_POINT('Ctrl Pts',(3.2768849260661,-17.9347368076371,11.658393449684));
#39749=CARTESIAN_POINT('Ctrl Pts',(3.38675242237018,-18.0299754494791,12.2483628505514));
#39750=CARTESIAN_POINT('Ctrl Pts',(3.75230183806937,-17.5557104881875,12.136196461057));
#39751=CARTESIAN_POINT('Ctrl Pts',(3.73678197419356,-18.3872566959992,11.4897869691041));
#39752=CARTESIAN_POINT('Ctrl Pts',(3.84184833985507,-18.5039941659567,12.1163869493151));
#39753=CARTESIAN_POINT('Ctrl Pts',(4.27892165345747,-18.0534823658125,11.9606798765339));
#39754=CARTESIAN_POINT('Ctrl Pts',(3.94731113881133,-18.639068823405,11.4032110584955));
#39755=CARTESIAN_POINT('Ctrl Pts',(4.0451517869323,-18.7653492151445,12.0507009440076));
#39756=CARTESIAN_POINT('Ctrl Pts',(4.51999480434176,-18.330475705872,11.8705557752602));
#39757=CARTESIAN_POINT('Ctrl Pts',(4.31140221038992,-19.1723450226265,11.2425461846842));
#39758=CARTESIAN_POINT('Ctrl Pts',(4.39127065776726,-19.307031058039,11.9329509628929));
#39759=CARTESIAN_POINT('Ctrl Pts',(4.93690892421083,-18.9170795247627,11.7033062729678));
#39760=CARTESIAN_POINT('Ctrl Pts',(4.46721666360654,-19.4553892620641,11.1676980332676));
#39761=CARTESIAN_POINT('Ctrl Pts',(4.53369372541373,-19.5890447445447,11.8809138577861));
#39762=CARTESIAN_POINT('Ctrl Pts',(5.11532924657178,-19.2284281878553,11.6253905765652));
#39763=CARTESIAN_POINT('Ctrl Pts',(4.66055289221914,-19.9067491525735,11.0708606665398));
#39764=CARTESIAN_POINT('Ctrl Pts',(4.70663959852945,-20.0253941374096,11.8162652162982));
#39765=CARTESIAN_POINT('Ctrl Pts',(5.33671507340206,-19.7249240680384,11.5245844638735));
#39766=CARTESIAN_POINT('Ctrl Pts',(4.71841700146108,-20.0625785423806,11.0410534672954));
#39767=CARTESIAN_POINT('Ctrl Pts',(4.75782043068565,-20.1754680451165,11.7967713101401));
#39768=CARTESIAN_POINT('Ctrl Pts',(5.40297422211345,-19.8963363966978,11.4935556590183));
#39769=CARTESIAN_POINT('Ctrl Pts',(4.81755437339946,-20.3765661077494,10.989129292382));
#39770=CARTESIAN_POINT('Ctrl Pts',(4.84482745319202,-20.475027517611,11.763343730263));
#39771=CARTESIAN_POINT('Ctrl Pts',(5.51649463909981,-20.2417227184453,11.4395034432688));
#39772=CARTESIAN_POINT('Ctrl Pts',(4.85917039071759,-20.5353092899111,10.9668478951731));
#39773=CARTESIAN_POINT('Ctrl Pts',(4.88061071522663,-20.6245738078917,11.7494242977742));
#39774=CARTESIAN_POINT('Ctrl Pts',(5.56414839021614,-20.4163402188943,11.4163088747902));
#39775=CARTESIAN_POINT('Ctrl Pts',(4.96045166571747,-21.0168172842587,10.9120800914172));
#39776=CARTESIAN_POINT('Ctrl Pts',(4.96782306317245,-21.0775974027918,11.7153595058825));
#39777=CARTESIAN_POINT('Ctrl Pts',(5.6801237512663,-20.9459990127004,11.359296487993));
#39778=CARTESIAN_POINT('Ctrl Pts',(4.99680880416774,-21.3448363866039,10.8916763988236));
#39779=CARTESIAN_POINT('Ctrl Pts',(4.99733458881033,-21.3762759056631,11.7036358385787));
#39780=CARTESIAN_POINT('Ctrl Pts',(5.72175565143888,-21.3068199155008,11.3380565795594));
#39781=CARTESIAN_POINT('Ctrl Pts',(4.99980122230293,-21.6804159506306,10.890014011117));
#39782=CARTESIAN_POINT('Ctrl Pts',(4.99983385337131,-21.6840753054423,11.7026485840482));
#39783=CARTESIAN_POINT('Ctrl Pts',(5.72518221930917,-21.6759575456936,11.3363260607529));
#40792=UNCERTAINTY_MEASURE_WITH_UNIT(LENGTH_MEASURE(0.01),#40810,
'DISTANCE_ACCURACY_VALUE',
'Maximum model space distance between geometric entities at asserted c
onnectivities');
#40799=UNCERTAINTY_MEASURE_WITH_UNIT(LENGTH_MEASURE(0.01),#40810,
'DISTANCE_ACCURACY_VALUE',
'Maximum model space distance between geometric entities at asserted c
onnectivities');
#40802=(
GEOMETRIC_REPRESENTATION_CONTEXT(3)
GLOBAL_UNCERTAINTY_ASSIGNED_CONTEXT((#40792))
GLOBAL_UNIT_ASSIGNED_CONTEXT((#40810,#40812,#40813))
REPRESENTATION_CONTEXT('','3D')
);
#40809=(
GEOMETRIC_REPRESENTATION_CONTEXT(3)
GLOBAL_UNCERTAINTY_ASSIGNED_CONTEXT((#40799))
GLOBAL_UNIT_ASSIGNED_CONTEXT((#40810,#40812,#40813))
REPRESENTATION_CONTEXT('','3D')
);
#40810=(
LENGTH_UNIT()
NAMED_UNIT(*)
SI_UNIT(.MILLI.,.METRE.)
);
#40812=(
NAMED_UNIT(*)
PLANE_ANGLE_UNIT()
SI_UNIT($,.RADIAN.)
);
#40813=(
NAMED_UNIT(*)
SI_UNIT($,.STERADIAN.)
SOLID_ANGLE_UNIT()
);
#40816=SHAPE_DEFINITION_REPRESENTATION(#40825,#40858);
#40825=PRODUCT_DEFINITION_SHAPE('',$,#40868);
#40858=SHAPE_REPRESENTATION('',(#6698),#40802);
#40865=PRODUCT_DEFINITION_CONTEXT('part definition',#40894,'design');
#40868=PRODUCT_DEFINITION('Rod','Rod',#40877,#40865);
#40877=PRODUCT_DEFINITION_FORMATION('',$,#40898);
#40894=APPLICATION_CONTEXT(
'Core Data for Automotive Mechanical Design Process');
#40895=PRODUCT_CONTEXT('part definition',#40894,'mechanical');
#40898=PRODUCT('Rod','Rod',$,(#40895));
#40907=PRESENTATION_STYLE_ASSIGNMENT((#40912));
#40912=SURFACE_STYLE_USAGE(.BOTH.,#40917);
#40917=SURFACE_SIDE_STYLE('',(#40922));
#40922=SURFACE_STYLE_FILL_AREA(#40927);
#40927=FILL_AREA_STYLE('Opaque(122,133,145)',(#40932));
#40932=FILL_AREA_STYLE_COLOUR('Opaque(122,133,145)',#40937);
#40937=COLOUR_RGB('Opaque(122,133,145)',0.47843137254902,0.52156862745098,
0.568627450980392);
ENDSEC;
END-ISO-10303-21;
